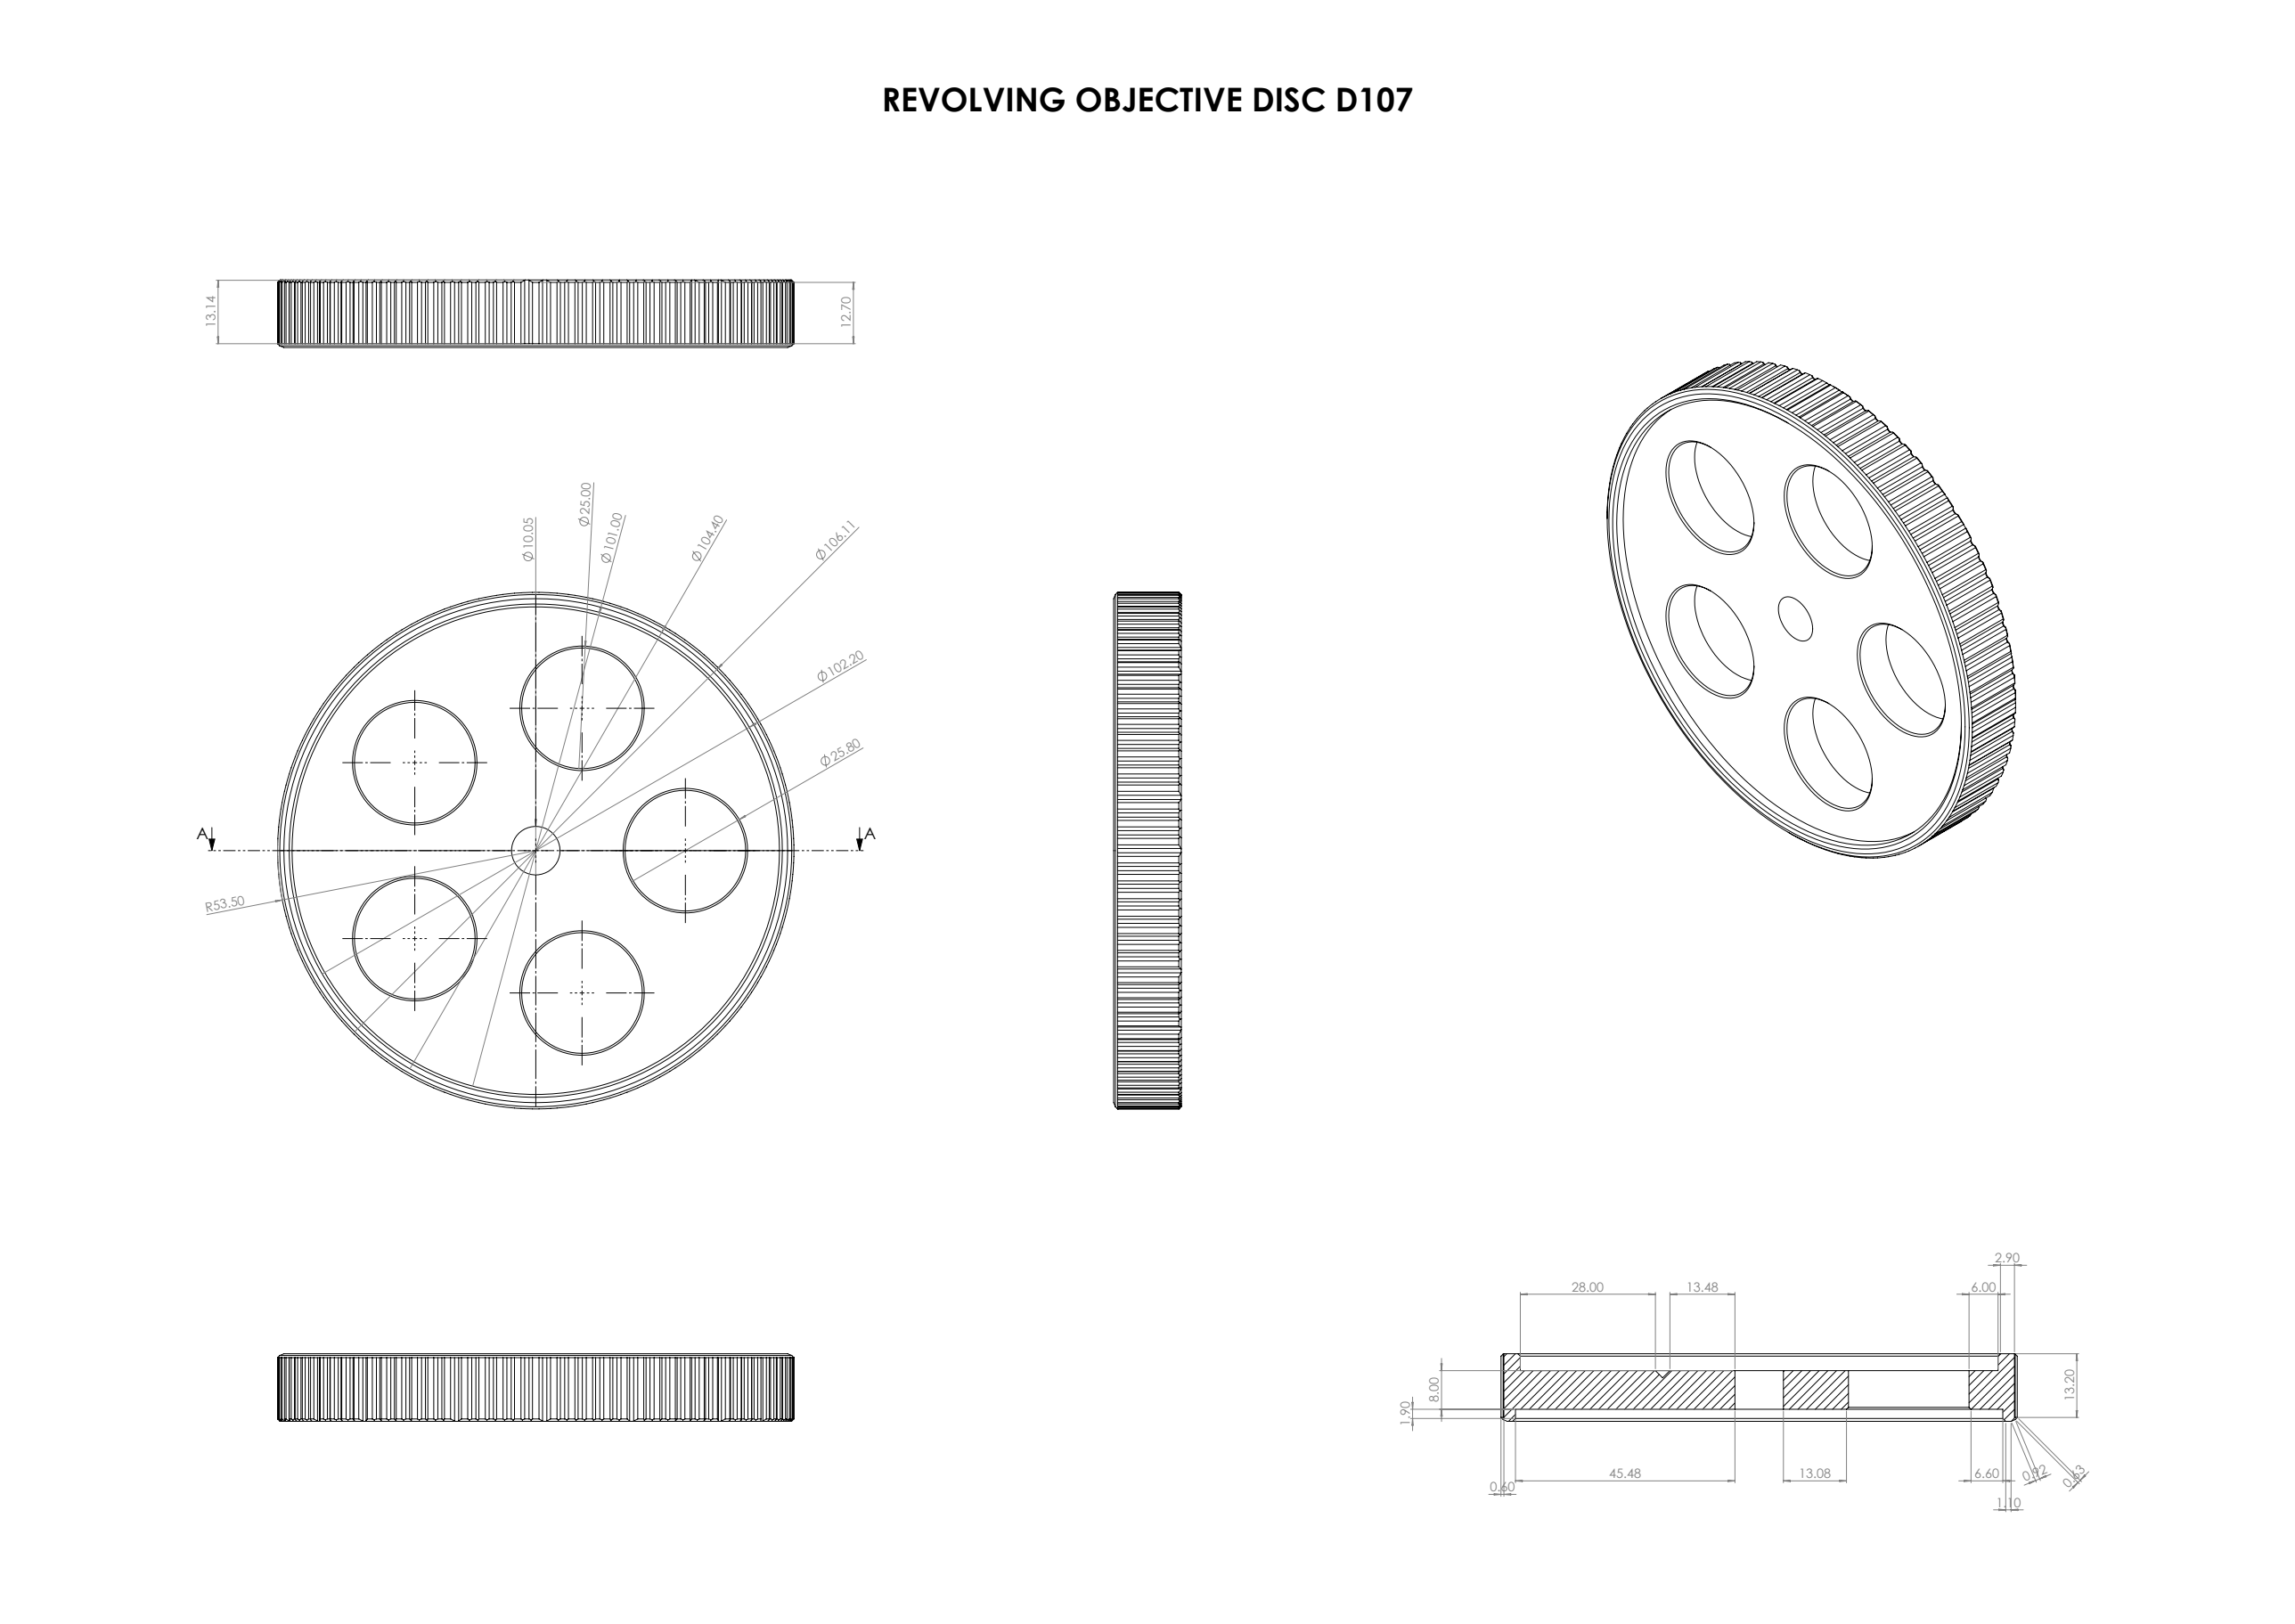
ISO-10303-21;
HEADER;
/* Generated by software containing ST-Developer
 * from STEP Tools, Inc. (www.steptools.com) 
 */

FILE_DESCRIPTION(
/* description */ (''),
/* implementation_level */ '2;1');

FILE_NAME(
/* name */ '02_Revolving_Objective_Disc_D107.step',
/* time_stamp */ '2026-10-21T02:03:06-07:00',
/* author */ (''),
/* organization */ (''),
/* preprocessor_version */ 'ST-DEVELOPER v20.2',
/* originating_system */ 'Autodesk Translation Framework v15.15.0.0',
/* authorisation */ '');

FILE_SCHEMA (('AUTOMOTIVE_DESIGN { 1 0 10303 214 3 1 1 }'));
ENDSEC;

DATA;
#10=MECHANICAL_DESIGN_GEOMETRIC_PRESENTATION_REPRESENTATION('',(#116),#38528);
#92=SHAPE_REPRESENTATION_RELATIONSHIP('SRR','None',#38577,#104);
#104=ADVANCED_BREP_SHAPE_REPRESENTATION('',(#128),#38517);
#116=STYLED_ITEM('',(#38720),#128);
#128=MANIFOLD_SOLID_BREP('Body1',#17073);
#146=CYLINDRICAL_SURFACE('',#17325,53.5);
#147=CYLINDRICAL_SURFACE('',#17331,53.5);
#148=CYLINDRICAL_SURFACE('',#17337,0.700000000000003);
#149=CYLINDRICAL_SURFACE('',#17344,0.700000000000003);
#150=CYLINDRICAL_SURFACE('',#17347,0.700000000000003);
#151=CYLINDRICAL_SURFACE('',#17356,0.700000000000003);
#152=CYLINDRICAL_SURFACE('',#17361,0.700000000000003);
#153=CYLINDRICAL_SURFACE('',#17368,53.5);
#154=CYLINDRICAL_SURFACE('',#17377,53.5);
#155=CYLINDRICAL_SURFACE('',#17384,53.5);
#156=CYLINDRICAL_SURFACE('',#17391,53.5);
#157=CYLINDRICAL_SURFACE('',#17398,53.5);
#158=CYLINDRICAL_SURFACE('',#17405,53.5);
#159=CYLINDRICAL_SURFACE('',#17412,53.5);
#160=CYLINDRICAL_SURFACE('',#17419,53.5);
#161=CYLINDRICAL_SURFACE('',#17426,53.5);
#162=CYLINDRICAL_SURFACE('',#17602,0.700000000000003);
#163=CYLINDRICAL_SURFACE('',#17608,0.700000000000003);
#164=CYLINDRICAL_SURFACE('',#17614,0.700000000000003);
#165=CYLINDRICAL_SURFACE('',#17620,0.700000000000003);
#166=CYLINDRICAL_SURFACE('',#17623,53.5);
#167=CYLINDRICAL_SURFACE('',#17631,53.5);
#168=CYLINDRICAL_SURFACE('',#17637,53.5);
#169=CYLINDRICAL_SURFACE('',#17643,53.5);
#170=CYLINDRICAL_SURFACE('',#17649,53.5);
#171=CYLINDRICAL_SURFACE('',#17655,53.5);
#172=CYLINDRICAL_SURFACE('',#17661,53.5);
#173=CYLINDRICAL_SURFACE('',#17670,53.5);
#174=CYLINDRICAL_SURFACE('',#17672,53.5);
#175=CYLINDRICAL_SURFACE('',#17674,53.5);
#176=CYLINDRICAL_SURFACE('',#17687,0.700000000000003);
#177=CYLINDRICAL_SURFACE('',#17689,0.700000000000003);
#178=CYLINDRICAL_SURFACE('',#17691,0.700000000000003);
#179=CYLINDRICAL_SURFACE('',#17693,0.700000000000003);
#180=CYLINDRICAL_SURFACE('',#17695,0.700000000000003);
#181=CYLINDRICAL_SURFACE('',#17697,0.700000000000003);
#182=CYLINDRICAL_SURFACE('',#17702,0.700000000000003);
#183=CYLINDRICAL_SURFACE('',#17710,0.700000000000003);
#184=CYLINDRICAL_SURFACE('',#17716,0.700000000000003);
#185=CYLINDRICAL_SURFACE('',#17722,0.700000000000003);
#186=CYLINDRICAL_SURFACE('',#17725,53.5);
#187=CYLINDRICAL_SURFACE('',#17733,53.5);
#188=CYLINDRICAL_SURFACE('',#17739,53.5);
#189=CYLINDRICAL_SURFACE('',#17745,53.5);
#190=CYLINDRICAL_SURFACE('',#17751,53.5);
#191=CYLINDRICAL_SURFACE('',#17757,53.5);
#192=CYLINDRICAL_SURFACE('',#17766,53.5);
#193=CYLINDRICAL_SURFACE('',#17768,53.5);
#194=CYLINDRICAL_SURFACE('',#17770,53.5);
#195=CYLINDRICAL_SURFACE('',#17772,53.5);
#196=CYLINDRICAL_SURFACE('',#17783,0.700000000000003);
#197=CYLINDRICAL_SURFACE('',#17785,0.700000000000003);
#198=CYLINDRICAL_SURFACE('',#17787,0.700000000000003);
#199=CYLINDRICAL_SURFACE('',#17789,0.700000000000003);
#200=CYLINDRICAL_SURFACE('',#17791,0.700000000000003);
#201=CYLINDRICAL_SURFACE('',#17796,0.700000000000003);
#202=CYLINDRICAL_SURFACE('',#17802,0.700000000000003);
#203=CYLINDRICAL_SURFACE('',#17808,0.700000000000003);
#204=CYLINDRICAL_SURFACE('',#17814,0.700000000000003);
#205=CYLINDRICAL_SURFACE('',#17820,0.700000000000003);
#206=CYLINDRICAL_SURFACE('',#17823,53.5);
#207=CYLINDRICAL_SURFACE('',#17831,53.5);
#208=CYLINDRICAL_SURFACE('',#17837,53.5);
#209=CYLINDRICAL_SURFACE('',#17843,53.5);
#210=CYLINDRICAL_SURFACE('',#17849,53.5);
#211=CYLINDRICAL_SURFACE('',#17862,53.5);
#212=CYLINDRICAL_SURFACE('',#17864,53.5);
#213=CYLINDRICAL_SURFACE('',#17866,53.5);
#214=CYLINDRICAL_SURFACE('',#17868,53.5);
#215=CYLINDRICAL_SURFACE('',#17870,53.5);
#216=CYLINDRICAL_SURFACE('',#17879,0.700000000000003);
#217=CYLINDRICAL_SURFACE('',#17881,0.700000000000003);
#218=CYLINDRICAL_SURFACE('',#17883,0.700000000000003);
#219=CYLINDRICAL_SURFACE('',#17885,0.700000000000003);
#220=CYLINDRICAL_SURFACE('',#17890,0.700000000000003);
#221=CYLINDRICAL_SURFACE('',#17898,0.700000000000003);
#222=CYLINDRICAL_SURFACE('',#17904,0.700000000000003);
#223=CYLINDRICAL_SURFACE('',#17910,0.700000000000003);
#224=CYLINDRICAL_SURFACE('',#17916,0.700000000000003);
#225=CYLINDRICAL_SURFACE('',#17922,0.700000000000003);
#226=CYLINDRICAL_SURFACE('',#17925,53.5);
#227=CYLINDRICAL_SURFACE('',#17933,53.5);
#228=CYLINDRICAL_SURFACE('',#17939,53.5);
#229=CYLINDRICAL_SURFACE('',#17945,53.5);
#230=CYLINDRICAL_SURFACE('',#17958,53.5);
#231=CYLINDRICAL_SURFACE('',#17960,53.5);
#232=CYLINDRICAL_SURFACE('',#17962,53.5);
#233=CYLINDRICAL_SURFACE('',#17964,53.5);
#234=CYLINDRICAL_SURFACE('',#17966,53.5);
#235=CYLINDRICAL_SURFACE('',#17968,53.5);
#236=CYLINDRICAL_SURFACE('',#17975,0.700000000000003);
#237=CYLINDRICAL_SURFACE('',#17977,0.700000000000003);
#238=CYLINDRICAL_SURFACE('',#17979,0.700000000000003);
#239=CYLINDRICAL_SURFACE('',#17984,0.700000000000003);
#240=CYLINDRICAL_SURFACE('',#17990,0.700000000000003);
#241=CYLINDRICAL_SURFACE('',#17996,0.700000000000003);
#242=CYLINDRICAL_SURFACE('',#18002,0.700000000000003);
#243=CYLINDRICAL_SURFACE('',#18008,0.700000000000003);
#244=CYLINDRICAL_SURFACE('',#18014,0.700000000000003);
#245=CYLINDRICAL_SURFACE('',#18020,0.700000000000003);
#246=CYLINDRICAL_SURFACE('',#18023,53.5);
#247=CYLINDRICAL_SURFACE('',#18031,53.5);
#248=CYLINDRICAL_SURFACE('',#18037,53.5);
#249=CYLINDRICAL_SURFACE('',#18054,53.5);
#250=CYLINDRICAL_SURFACE('',#18056,53.5);
#251=CYLINDRICAL_SURFACE('',#18058,53.5);
#252=CYLINDRICAL_SURFACE('',#18060,53.5);
#253=CYLINDRICAL_SURFACE('',#18062,53.5);
#254=CYLINDRICAL_SURFACE('',#18064,53.5);
#255=CYLINDRICAL_SURFACE('',#18066,53.5);
#256=CYLINDRICAL_SURFACE('',#18071,0.700000000000003);
#257=CYLINDRICAL_SURFACE('',#18073,0.700000000000003);
#258=CYLINDRICAL_SURFACE('',#18078,0.700000000000003);
#259=CYLINDRICAL_SURFACE('',#18084,0.700000000000003);
#260=CYLINDRICAL_SURFACE('',#18090,0.700000000000003);
#261=CYLINDRICAL_SURFACE('',#18096,0.700000000000003);
#262=CYLINDRICAL_SURFACE('',#18102,0.700000000000003);
#263=CYLINDRICAL_SURFACE('',#18108,0.700000000000003);
#264=CYLINDRICAL_SURFACE('',#18114,0.700000000000003);
#265=CYLINDRICAL_SURFACE('',#18120,0.700000000000003);
#266=CYLINDRICAL_SURFACE('',#18123,53.5);
#267=CYLINDRICAL_SURFACE('',#18131,53.5);
#268=CYLINDRICAL_SURFACE('',#18150,53.5);
#269=CYLINDRICAL_SURFACE('',#18152,53.5);
#270=CYLINDRICAL_SURFACE('',#18154,53.5);
#271=CYLINDRICAL_SURFACE('',#18156,53.5);
#272=CYLINDRICAL_SURFACE('',#18158,53.5);
#273=CYLINDRICAL_SURFACE('',#18160,53.5);
#274=CYLINDRICAL_SURFACE('',#18162,53.5);
#275=CYLINDRICAL_SURFACE('',#18164,53.5);
#276=CYLINDRICAL_SURFACE('',#18167,0.700000000000003);
#277=CYLINDRICAL_SURFACE('',#18172,53.5);
#278=CYLINDRICAL_SURFACE('',#18178,53.5);
#279=CYLINDRICAL_SURFACE('',#18184,53.5);
#280=CYLINDRICAL_SURFACE('',#18190,53.5);
#281=CYLINDRICAL_SURFACE('',#18196,53.5);
#282=CYLINDRICAL_SURFACE('',#18202,53.5);
#283=CYLINDRICAL_SURFACE('',#18208,53.5);
#284=CYLINDRICAL_SURFACE('',#18214,53.5);
#285=CYLINDRICAL_SURFACE('',#18220,53.5);
#286=CYLINDRICAL_SURFACE('',#18223,0.700000000000003);
#287=CYLINDRICAL_SURFACE('',#18244,0.700000000000003);
#288=CYLINDRICAL_SURFACE('',#18246,0.700000000000003);
#289=CYLINDRICAL_SURFACE('',#18248,0.700000000000003);
#290=CYLINDRICAL_SURFACE('',#18250,0.700000000000003);
#291=CYLINDRICAL_SURFACE('',#18252,0.700000000000003);
#292=CYLINDRICAL_SURFACE('',#18254,0.700000000000003);
#293=CYLINDRICAL_SURFACE('',#18256,0.700000000000003);
#294=CYLINDRICAL_SURFACE('',#18258,0.700000000000003);
#295=CYLINDRICAL_SURFACE('',#18262,49.5);
#296=CYLINDRICAL_SURFACE('',#18281,0.700000000000003);
#297=CYLINDRICAL_SURFACE('',#18283,0.700000000000003);
#298=CYLINDRICAL_SURFACE('',#18285,0.700000000000003);
#299=CYLINDRICAL_SURFACE('',#18287,0.700000000000003);
#300=CYLINDRICAL_SURFACE('',#18289,0.700000000000003);
#301=CYLINDRICAL_SURFACE('',#18291,0.700000000000003);
#302=CYLINDRICAL_SURFACE('',#18293,0.700000000000003);
#303=CYLINDRICAL_SURFACE('',#18295,0.700000000000003);
#304=CYLINDRICAL_SURFACE('',#18297,0.700000000000003);
#305=CYLINDRICAL_SURFACE('',#18300,0.700000000000003);
#306=CYLINDRICAL_SURFACE('',#18306,0.700000000000003);
#307=CYLINDRICAL_SURFACE('',#18312,0.700000000000003);
#308=CYLINDRICAL_SURFACE('',#18318,0.700000000000003);
#309=CYLINDRICAL_SURFACE('',#18324,0.700000000000003);
#310=CYLINDRICAL_SURFACE('',#18330,0.700000000000003);
#311=CYLINDRICAL_SURFACE('',#18453,12.5);
#312=CYLINDRICAL_SURFACE('',#18457,12.5);
#313=CYLINDRICAL_SURFACE('',#18461,12.5);
#314=CYLINDRICAL_SURFACE('',#18465,12.5);
#315=CYLINDRICAL_SURFACE('',#18469,12.5);
#316=CYLINDRICAL_SURFACE('',#18473,50.5);
#317=CYLINDRICAL_SURFACE('',#18474,53.5);
#318=CYLINDRICAL_SURFACE('',#18475,53.5);
#319=CYLINDRICAL_SURFACE('',#18476,53.5);
#320=CYLINDRICAL_SURFACE('',#18477,53.5);
#321=CYLINDRICAL_SURFACE('',#18478,53.5);
#322=CYLINDRICAL_SURFACE('',#18479,53.5);
#323=CYLINDRICAL_SURFACE('',#18480,53.5);
#324=CYLINDRICAL_SURFACE('',#18481,53.5);
#325=CYLINDRICAL_SURFACE('',#18482,53.5);
#326=CYLINDRICAL_SURFACE('',#18483,53.5);
#327=CYLINDRICAL_SURFACE('',#18490,0.700000000000003);
#328=CYLINDRICAL_SURFACE('',#18502,0.700000000000003);
#329=CYLINDRICAL_SURFACE('',#18514,0.700000000000003);
#330=CYLINDRICAL_SURFACE('',#18558,0.700000000000003);
#331=CYLINDRICAL_SURFACE('',#18568,0.700000000000003);
#332=CYLINDRICAL_SURFACE('',#18580,0.700000000000003);
#333=CYLINDRICAL_SURFACE('',#18596,5.025);
#431=B_SPLINE_CURVE_WITH_KNOTS('',3,(#24013,#24014,#24015,#24016),
 .UNSPECIFIED.,.F.,.F.,(4,4),(0.165217092335985,0.177184346430037),
 .UNSPECIFIED.);
#432=B_SPLINE_CURVE_WITH_KNOTS('',3,(#24020,#24021,#24022,#24023),
 .UNSPECIFIED.,.F.,.F.,(4,4),(0.,0.0446132763744268),.UNSPECIFIED.);
#433=B_SPLINE_CURVE_WITH_KNOTS('',3,(#24050,#24051,#24052,#24053),
 .UNSPECIFIED.,.F.,.F.,(4,4),(0.0319696744346156,0.0766821311551608),
 .UNSPECIFIED.);
#434=B_SPLINE_CURVE_WITH_KNOTS('',3,(#24057,#24058,#24059,#24060),
 .UNSPECIFIED.,.F.,.F.,(4,4),(0.077355308281931,0.0893225623759921),
 .UNSPECIFIED.);
#435=B_SPLINE_CURVE_WITH_KNOTS('',3,(#24072,#24073,#24074,#24075),
 .UNSPECIFIED.,.F.,.F.,(4,4),(0.165217092335986,0.177184346430046),
 .UNSPECIFIED.);
#436=B_SPLINE_CURVE_WITH_KNOTS('',3,(#24102,#24103,#24104,#24105),
 .UNSPECIFIED.,.F.,.F.,(4,4),(0.0319696744346149,0.0766821311551634),
 .UNSPECIFIED.);
#437=B_SPLINE_CURVE_WITH_KNOTS('',3,(#24108,#24109,#24110,#24111),
 .UNSPECIFIED.,.F.,.F.,(4,4),(0.0319696744346139,0.0766821311551655),
 .UNSPECIFIED.);
#438=B_SPLINE_CURVE_WITH_KNOTS('',3,(#24136,#24137,#24138,#24139),
 .UNSPECIFIED.,.F.,.F.,(4,4),(0.031969674434604,0.0766821311551636),
 .UNSPECIFIED.);
#439=B_SPLINE_CURVE_WITH_KNOTS('',3,(#24164,#24165,#24166,#24167),
 .UNSPECIFIED.,.F.,.F.,(4,4),(0.0319696744346154,0.0766821311551577),
 .UNSPECIFIED.);
#440=B_SPLINE_CURVE_WITH_KNOTS('',3,(#24170,#24171,#24172,#24173),
 .UNSPECIFIED.,.F.,.F.,(4,4),(0.0319696744346157,0.0766821311551629),
 .UNSPECIFIED.);
#441=B_SPLINE_CURVE_WITH_KNOTS('',3,(#24207,#24208,#24209,#24210),
 .UNSPECIFIED.,.F.,.F.,(4,4),(0.0773553082819434,0.089322562375993),
 .UNSPECIFIED.);
#442=B_SPLINE_CURVE_WITH_KNOTS('',3,(#24214,#24215,#24216,#24217),
 .UNSPECIFIED.,.F.,.F.,(4,4),(-0.177184216772292,-0.165217092335991),
 .UNSPECIFIED.);
#443=B_SPLINE_CURVE_WITH_KNOTS('',3,(#24225,#24226,#24227,#24228),
 .UNSPECIFIED.,.F.,.F.,(4,4),(0.,0.0964441447221119),.UNSPECIFIED.);
#444=B_SPLINE_CURVE_WITH_KNOTS('',3,(#24230,#24231,#24232,#24233),
 .UNSPECIFIED.,.F.,.F.,(4,4),(0.336279561120239,0.348246685406907),
 .UNSPECIFIED.);
#445=B_SPLINE_CURVE_WITH_KNOTS('',3,(#24258,#24259,#24260,#24261),
 .UNSPECIFIED.,.F.,.F.,(4,4),(0.0319696744346043,0.0766821311551631),
 .UNSPECIFIED.);
#446=B_SPLINE_CURVE_WITH_KNOTS('',3,(#24265,#24266,#24267,#24268),
 .UNSPECIFIED.,.F.,.F.,(4,4),(-0.0893225623759883,-0.0773554379396765),
 .UNSPECIFIED.);
#447=B_SPLINE_CURVE_WITH_KNOTS('',3,(#24269,#24270,#24271,#24272),
 .UNSPECIFIED.,.F.,.F.,(4,4),(0.,0.0964441447217045),.UNSPECIFIED.);
#448=B_SPLINE_CURVE_WITH_KNOTS('',3,(#24296,#24297,#24298,#24299),
 .UNSPECIFIED.,.F.,.F.,(4,4),(0.0319696744346058,0.0766821311551602),
 .UNSPECIFIED.);
#449=B_SPLINE_CURVE_WITH_KNOTS('',3,(#24302,#24303,#24304,#24305),
 .UNSPECIFIED.,.F.,.F.,(4,4),(0.0319696744346046,0.0766821311551621),
 .UNSPECIFIED.);
#450=B_SPLINE_CURVE_WITH_KNOTS('',3,(#24341,#24342,#24343,#24344),
 .UNSPECIFIED.,.F.,.F.,(4,4),(0.0319696744346149,0.0766821311551593),
 .UNSPECIFIED.);
#451=B_SPLINE_CURVE_WITH_KNOTS('',3,(#24347,#24348,#24349,#24350),
 .UNSPECIFIED.,.F.,.F.,(4,4),(0.0319696744346029,0.0766821311551658),
 .UNSPECIFIED.);
#452=B_SPLINE_CURVE_WITH_KNOTS('',3,(#24386,#24387,#24388,#24389),
 .UNSPECIFIED.,.F.,.F.,(4,4),(0.0319696744346075,0.0766821311551552),
 .UNSPECIFIED.);
#453=B_SPLINE_CURVE_WITH_KNOTS('',3,(#24392,#24393,#24394,#24395),
 .UNSPECIFIED.,.F.,.F.,(4,4),(0.0319696744346153,0.0766821311551614),
 .UNSPECIFIED.);
#454=B_SPLINE_CURVE_WITH_KNOTS('',3,(#24431,#24432,#24433,#24434),
 .UNSPECIFIED.,.F.,.F.,(4,4),(0.0319696744346164,0.0766821311551606),
 .UNSPECIFIED.);
#455=B_SPLINE_CURVE_WITH_KNOTS('',3,(#24437,#24438,#24439,#24440),
 .UNSPECIFIED.,.F.,.F.,(4,4),(0.0319696744346151,0.0766821311551609),
 .UNSPECIFIED.);
#456=B_SPLINE_CURVE_WITH_KNOTS('',3,(#24476,#24477,#24478,#24479),
 .UNSPECIFIED.,.F.,.F.,(4,4),(0.0319696744346051,0.076682131155159),
 .UNSPECIFIED.);
#457=B_SPLINE_CURVE_WITH_KNOTS('',3,(#24482,#24483,#24484,#24485),
 .UNSPECIFIED.,.F.,.F.,(4,4),(0.0319696744346129,0.0766821311551604),
 .UNSPECIFIED.);
#458=B_SPLINE_CURVE_WITH_KNOTS('',3,(#24521,#24522,#24523,#24524),
 .UNSPECIFIED.,.F.,.F.,(4,4),(0.0319696744346068,0.0766821311551503),
 .UNSPECIFIED.);
#459=B_SPLINE_CURVE_WITH_KNOTS('',3,(#24527,#24528,#24529,#24530),
 .UNSPECIFIED.,.F.,.F.,(4,4),(0.031969674434606,0.0766821311551618),
 .UNSPECIFIED.);
#460=B_SPLINE_CURVE_WITH_KNOTS('',3,(#24566,#24567,#24568,#24569),
 .UNSPECIFIED.,.F.,.F.,(4,4),(0.0319696744346057,0.0766821311551617),
 .UNSPECIFIED.);
#461=B_SPLINE_CURVE_WITH_KNOTS('',3,(#24572,#24573,#24574,#24575),
 .UNSPECIFIED.,.F.,.F.,(4,4),(0.0319696744346062,0.0766821311551594),
 .UNSPECIFIED.);
#462=B_SPLINE_CURVE_WITH_KNOTS('',3,(#24611,#24612,#24613,#24614),
 .UNSPECIFIED.,.F.,.F.,(4,4),(0.0319696744346062,0.0766821311551613),
 .UNSPECIFIED.);
#463=B_SPLINE_CURVE_WITH_KNOTS('',3,(#24617,#24618,#24619,#24620),
 .UNSPECIFIED.,.F.,.F.,(4,4),(0.0319696744346139,0.0766821311551679),
 .UNSPECIFIED.);
#464=B_SPLINE_CURVE_WITH_KNOTS('',3,(#24641,#24642,#24643,#24644,#24645,
#24646),.UNSPECIFIED.,.F.,.F.,(4,2,4),(1.36037627907923,1.38960835652673,
1.40296484627234),.UNSPECIFIED.);
#465=B_SPLINE_CURVE_WITH_KNOTS('',3,(#24662,#24663,#24664,#24665),
 .UNSPECIFIED.,.F.,.F.,(4,4),(0.16521709233599,0.177184216772299),
 .UNSPECIFIED.);
#466=B_SPLINE_CURVE_WITH_KNOTS('',3,(#24983,#24984,#24985,#24986),
 .UNSPECIFIED.,.F.,.F.,(4,4),(-0.0893225623759853,-0.0773554379396747),
 .UNSPECIFIED.);
#467=B_SPLINE_CURVE_WITH_KNOTS('',3,(#25013,#25014,#25015,#25016),
 .UNSPECIFIED.,.F.,.F.,(4,4),(0.0319696744346003,0.0766821311551615),
 .UNSPECIFIED.);
#468=B_SPLINE_CURVE_WITH_KNOTS('',3,(#25017,#25018,#25019,#25020),
 .UNSPECIFIED.,.F.,.F.,(4,4),(0.0319696744346077,0.0766821311551524),
 .UNSPECIFIED.);
#469=B_SPLINE_CURVE_WITH_KNOTS('',3,(#25055,#25056,#25057,#25058),
 .UNSPECIFIED.,.F.,.F.,(4,4),(0.0319696744346155,0.0766821311551595),
 .UNSPECIFIED.);
#470=B_SPLINE_CURVE_WITH_KNOTS('',3,(#25059,#25060,#25061,#25062),
 .UNSPECIFIED.,.F.,.F.,(4,4),(0.0319696744346145,0.0766821311551639),
 .UNSPECIFIED.);
#471=B_SPLINE_CURVE_WITH_KNOTS('',3,(#25097,#25098,#25099,#25100),
 .UNSPECIFIED.,.F.,.F.,(4,4),(0.0319696744346048,0.0766821311551673),
 .UNSPECIFIED.);
#472=B_SPLINE_CURVE_WITH_KNOTS('',3,(#25101,#25102,#25103,#25104),
 .UNSPECIFIED.,.F.,.F.,(4,4),(0.0319696744346148,0.0766821311551611),
 .UNSPECIFIED.);
#473=B_SPLINE_CURVE_WITH_KNOTS('',3,(#25147,#25148,#25149,#25150),
 .UNSPECIFIED.,.F.,.F.,(4,4),(0.0319696744346167,0.0766821311551506),
 .UNSPECIFIED.);
#474=B_SPLINE_CURVE_WITH_KNOTS('',3,(#25151,#25152,#25153,#25154),
 .UNSPECIFIED.,.F.,.F.,(4,4),(0.0773553082819305,0.0893225623759919),
 .UNSPECIFIED.);
#475=B_SPLINE_CURVE_WITH_KNOTS('',3,(#25189,#25190,#25191,#25192),
 .UNSPECIFIED.,.F.,.F.,(4,4),(0.0319696744346161,0.0766821311551558),
 .UNSPECIFIED.);
#476=B_SPLINE_CURVE_WITH_KNOTS('',3,(#25193,#25194,#25195,#25196),
 .UNSPECIFIED.,.F.,.F.,(4,4),(0.031969674434606,0.0766821311551616),
 .UNSPECIFIED.);
#477=B_SPLINE_CURVE_WITH_KNOTS('',3,(#25231,#25232,#25233,#25234),
 .UNSPECIFIED.,.F.,.F.,(4,4),(0.031969674434617,0.0766821311551659),
 .UNSPECIFIED.);
#478=B_SPLINE_CURVE_WITH_KNOTS('',3,(#25235,#25236,#25237,#25238),
 .UNSPECIFIED.,.F.,.F.,(4,4),(0.0319696744346159,0.0766821311551567),
 .UNSPECIFIED.);
#479=B_SPLINE_CURVE_WITH_KNOTS('',3,(#25273,#25274,#25275,#25276),
 .UNSPECIFIED.,.F.,.F.,(4,4),(0.0319696744346169,0.0766821311551513),
 .UNSPECIFIED.);
#480=B_SPLINE_CURVE_WITH_KNOTS('',3,(#25277,#25278,#25279,#25280),
 .UNSPECIFIED.,.F.,.F.,(4,4),(0.0319696744346152,0.0766821311551648),
 .UNSPECIFIED.);
#481=B_SPLINE_CURVE_WITH_KNOTS('',3,(#25315,#25316,#25317,#25318),
 .UNSPECIFIED.,.F.,.F.,(4,4),(0.0319696744346174,0.0766821311551486),
 .UNSPECIFIED.);
#482=B_SPLINE_CURVE_WITH_KNOTS('',3,(#25319,#25320,#25321,#25322),
 .UNSPECIFIED.,.F.,.F.,(4,4),(0.0319696744346054,0.0766821311551601),
 .UNSPECIFIED.);
#483=B_SPLINE_CURVE_WITH_KNOTS('',3,(#25357,#25358,#25359,#25360),
 .UNSPECIFIED.,.F.,.F.,(4,4),(0.165217092335987,0.177184346430039),
 .UNSPECIFIED.);
#484=B_SPLINE_CURVE_WITH_KNOTS('',3,(#25361,#25362,#25363,#25364),
 .UNSPECIFIED.,.F.,.F.,(4,4),(0.0319696744346053,0.0766821311551563),
 .UNSPECIFIED.);
#485=B_SPLINE_CURVE_WITH_KNOTS('',3,(#25377,#25378,#25379,#25380),
 .UNSPECIFIED.,.F.,.F.,(4,4),(0.,0.0964441447213629),.UNSPECIFIED.);
#486=B_SPLINE_CURVE_WITH_KNOTS('',3,(#25382,#25383,#25384,#25385),
 .UNSPECIFIED.,.F.,.F.,(4,4),(-0.0893225623759869,-0.0773554379396867),
 .UNSPECIFIED.);
#487=B_SPLINE_CURVE_WITH_KNOTS('',3,(#25445,#25446,#25447,#25448),
 .UNSPECIFIED.,.F.,.F.,(4,4),(0.,0.0446132763744278),.UNSPECIFIED.);
#488=B_SPLINE_CURVE_WITH_KNOTS('',3,(#25449,#25450,#25451,#25452),
 .UNSPECIFIED.,.F.,.F.,(4,4),(0.0319696744346159,0.0766821311551664),
 .UNSPECIFIED.);
#489=B_SPLINE_CURVE_WITH_KNOTS('',3,(#25472,#25473,#25474,#25475),
 .UNSPECIFIED.,.F.,.F.,(4,4),(0.0319696744346157,0.0766821311551561),
 .UNSPECIFIED.);
#490=B_SPLINE_CURVE_WITH_KNOTS('',3,(#25493,#25494,#25495,#25496),
 .UNSPECIFIED.,.F.,.F.,(4,4),(0.0319696744346008,0.076682131155157),
 .UNSPECIFIED.);
#491=B_SPLINE_CURVE_WITH_KNOTS('',3,(#25531,#25532,#25533,#25534),
 .UNSPECIFIED.,.F.,.F.,(4,4),(0.0319696744346162,0.0766821311551517),
 .UNSPECIFIED.);
#492=B_SPLINE_CURVE_WITH_KNOTS('',3,(#25535,#25536,#25537,#25538),
 .UNSPECIFIED.,.F.,.F.,(4,4),(0.031969674434614,0.0766821311551579),
 .UNSPECIFIED.);
#493=B_SPLINE_CURVE_WITH_KNOTS('',3,(#25573,#25574,#25575,#25576),
 .UNSPECIFIED.,.F.,.F.,(4,4),(0.0319696744346152,0.0766821311551576),
 .UNSPECIFIED.);
#494=B_SPLINE_CURVE_WITH_KNOTS('',3,(#25577,#25578,#25579,#25580),
 .UNSPECIFIED.,.F.,.F.,(4,4),(0.0319696744346146,0.076682131155164),
 .UNSPECIFIED.);
#495=B_SPLINE_CURVE_WITH_KNOTS('',3,(#25603,#25604,#25605,#25606),
 .UNSPECIFIED.,.F.,.F.,(4,4),(0.165217092335987,0.177184346430036),
 .UNSPECIFIED.);
#496=B_SPLINE_CURVE_WITH_KNOTS('',3,(#25630,#25631,#25632,#25633),
 .UNSPECIFIED.,.F.,.F.,(4,4),(0.0319696744346059,0.0766821311551569),
 .UNSPECIFIED.);
#497=B_SPLINE_CURVE_WITH_KNOTS('',3,(#25634,#25635,#25636,#25637),
 .UNSPECIFIED.,.F.,.F.,(4,4),(0.0773553082819314,0.0893225623759902),
 .UNSPECIFIED.);
#498=B_SPLINE_CURVE_WITH_KNOTS('',3,(#25672,#25673,#25674,#25675),
 .UNSPECIFIED.,.F.,.F.,(4,4),(0.0319696744345999,0.0766821311551614),
 .UNSPECIFIED.);
#499=B_SPLINE_CURVE_WITH_KNOTS('',3,(#25676,#25677,#25678,#25679),
 .UNSPECIFIED.,.F.,.F.,(4,4),(0.0319696744346005,0.0766821311551545),
 .UNSPECIFIED.);
#500=B_SPLINE_CURVE_WITH_KNOTS('',3,(#25714,#25715,#25716,#25717),
 .UNSPECIFIED.,.F.,.F.,(4,4),(0.0319696744346044,0.0766821311551586),
 .UNSPECIFIED.);
#501=B_SPLINE_CURVE_WITH_KNOTS('',3,(#25718,#25719,#25720,#25721),
 .UNSPECIFIED.,.F.,.F.,(4,4),(0.0319696744346146,0.0766821311551602),
 .UNSPECIFIED.);
#502=B_SPLINE_CURVE_WITH_KNOTS('',3,(#25756,#25757,#25758,#25759),
 .UNSPECIFIED.,.F.,.F.,(4,4),(0.0319696744345999,0.0766821311551589),
 .UNSPECIFIED.);
#503=B_SPLINE_CURVE_WITH_KNOTS('',3,(#25760,#25761,#25762,#25763),
 .UNSPECIFIED.,.F.,.F.,(4,4),(0.0319696744346151,0.0766821311551586),
 .UNSPECIFIED.);
#504=B_SPLINE_CURVE_WITH_KNOTS('',3,(#25798,#25799,#25800,#25801),
 .UNSPECIFIED.,.F.,.F.,(4,4),(0.165217092335985,0.177184346430047),
 .UNSPECIFIED.);
#505=B_SPLINE_CURVE_WITH_KNOTS('',3,(#25802,#25803,#25804,#25805),
 .UNSPECIFIED.,.F.,.F.,(4,4),(0.,0.0446132763744527),.UNSPECIFIED.);
#506=B_SPLINE_CURVE_WITH_KNOTS('',3,(#25818,#25819,#25820,#25821),
 .UNSPECIFIED.,.F.,.F.,(4,4),(0.,0.0964441447213381),.UNSPECIFIED.);
#507=B_SPLINE_CURVE_WITH_KNOTS('',3,(#25823,#25824,#25825,#25826),
 .UNSPECIFIED.,.F.,.F.,(4,4),(-0.0893225623759864,-0.0773554379396737),
 .UNSPECIFIED.);
#508=B_SPLINE_CURVE_WITH_KNOTS('',3,(#25884,#25885,#25886,#25887),
 .UNSPECIFIED.,.F.,.F.,(4,4),(0.0319696744346151,0.0766821311551646),
 .UNSPECIFIED.);
#509=B_SPLINE_CURVE_WITH_KNOTS('',3,(#25888,#25889,#25890,#25891),
 .UNSPECIFIED.,.F.,.F.,(4,4),(0.0319696744346152,0.0766821311551612),
 .UNSPECIFIED.);
#510=B_SPLINE_CURVE_WITH_KNOTS('',3,(#25926,#25927,#25928,#25929),
 .UNSPECIFIED.,.F.,.F.,(4,4),(0.031969674434616,0.0766821311551564),
 .UNSPECIFIED.);
#511=B_SPLINE_CURVE_WITH_KNOTS('',3,(#25930,#25931,#25932,#25933),
 .UNSPECIFIED.,.F.,.F.,(4,4),(0.0319696744346053,0.0766821311551682),
 .UNSPECIFIED.);
#512=B_SPLINE_CURVE_WITH_KNOTS('',3,(#25968,#25969,#25970,#25971),
 .UNSPECIFIED.,.F.,.F.,(4,4),(0.0319696744346154,0.0766821311551632),
 .UNSPECIFIED.);
#513=B_SPLINE_CURVE_WITH_KNOTS('',3,(#25972,#25973,#25974,#25975),
 .UNSPECIFIED.,.F.,.F.,(4,4),(0.0319696744346182,0.0766821311551516),
 .UNSPECIFIED.);
#514=B_SPLINE_CURVE_WITH_KNOTS('',3,(#26010,#26011,#26012,#26013),
 .UNSPECIFIED.,.F.,.F.,(4,4),(0.0319696744346054,0.076682131155166),
 .UNSPECIFIED.);
#515=B_SPLINE_CURVE_WITH_KNOTS('',3,(#26014,#26015,#26016,#26017),
 .UNSPECIFIED.,.F.,.F.,(4,4),(0.0319696744346067,0.0766821311551598),
 .UNSPECIFIED.);
#516=B_SPLINE_CURVE_WITH_KNOTS('',3,(#26052,#26053,#26054,#26055),
 .UNSPECIFIED.,.F.,.F.,(4,4),(0.0319696744346162,0.0766821311551578),
 .UNSPECIFIED.);
#517=B_SPLINE_CURVE_WITH_KNOTS('',3,(#26056,#26057,#26058,#26059),
 .UNSPECIFIED.,.F.,.F.,(4,4),(0.0319696744346034,0.0766821311551686),
 .UNSPECIFIED.);
#518=B_SPLINE_CURVE_WITH_KNOTS('',3,(#26082,#26083,#26084,#26085),
 .UNSPECIFIED.,.F.,.F.,(4,4),(0.165217092335987,0.17718434643005),
 .UNSPECIFIED.);
#519=B_SPLINE_CURVE_WITH_KNOTS('',3,(#26109,#26110,#26111,#26112),
 .UNSPECIFIED.,.F.,.F.,(4,4),(0.0319696744346091,0.0766821311551474),
 .UNSPECIFIED.);
#520=B_SPLINE_CURVE_WITH_KNOTS('',3,(#26113,#26114,#26115,#26116),
 .UNSPECIFIED.,.F.,.F.,(4,4),(0.077355308281932,0.0893225623759954),
 .UNSPECIFIED.);
#521=B_SPLINE_CURVE_WITH_KNOTS('',3,(#26151,#26152,#26153,#26154),
 .UNSPECIFIED.,.F.,.F.,(4,4),(0.0319696744346146,0.0766821311551647),
 .UNSPECIFIED.);
#522=B_SPLINE_CURVE_WITH_KNOTS('',3,(#26155,#26156,#26157,#26158),
 .UNSPECIFIED.,.F.,.F.,(4,4),(0.0319696744346137,0.0766821311551644),
 .UNSPECIFIED.);
#523=B_SPLINE_CURVE_WITH_KNOTS('',3,(#26193,#26194,#26195,#26196),
 .UNSPECIFIED.,.F.,.F.,(4,4),(0.0319696744346069,0.0766821311551582),
 .UNSPECIFIED.);
#524=B_SPLINE_CURVE_WITH_KNOTS('',3,(#26197,#26198,#26199,#26200),
 .UNSPECIFIED.,.F.,.F.,(4,4),(0.0319696744346155,0.0766821311551643),
 .UNSPECIFIED.);
#525=B_SPLINE_CURVE_WITH_KNOTS('',3,(#26235,#26236,#26237,#26238),
 .UNSPECIFIED.,.F.,.F.,(4,4),(0.165217092335985,0.177184346430037),
 .UNSPECIFIED.);
#526=B_SPLINE_CURVE_WITH_KNOTS('',3,(#26239,#26240,#26241,#26242),
 .UNSPECIFIED.,.F.,.F.,(4,4),(0.031969674434605,0.0766821311551589),
 .UNSPECIFIED.);
#527=B_SPLINE_CURVE_WITH_KNOTS('',3,(#26255,#26256,#26257,#26258),
 .UNSPECIFIED.,.F.,.F.,(4,4),(0.,0.0964441447218811),.UNSPECIFIED.);
#528=B_SPLINE_CURVE_WITH_KNOTS('',3,(#26260,#26261,#26262,#26263),
 .UNSPECIFIED.,.F.,.F.,(4,4),(-0.0893225623759877,-0.0773554379396747),
 .UNSPECIFIED.);
#529=B_SPLINE_CURVE_WITH_KNOTS('',3,(#26323,#26324,#26325,#26326),
 .UNSPECIFIED.,.F.,.F.,(4,4),(0.,0.0446132763744454),.UNSPECIFIED.);
#530=B_SPLINE_CURVE_WITH_KNOTS('',3,(#26327,#26328,#26329,#26330),
 .UNSPECIFIED.,.F.,.F.,(4,4),(0.0319696744346051,0.0766821311551664),
 .UNSPECIFIED.);
#531=B_SPLINE_CURVE_WITH_KNOTS('',3,(#26350,#26351,#26352,#26353),
 .UNSPECIFIED.,.F.,.F.,(4,4),(0.0319696744346155,0.0766821311551594),
 .UNSPECIFIED.);
#532=B_SPLINE_CURVE_WITH_KNOTS('',3,(#26371,#26372,#26373,#26374),
 .UNSPECIFIED.,.F.,.F.,(4,4),(0.0319696744346062,0.0766821311551557),
 .UNSPECIFIED.);
#533=B_SPLINE_CURVE_WITH_KNOTS('',3,(#26409,#26410,#26411,#26412),
 .UNSPECIFIED.,.F.,.F.,(4,4),(0.0319696744346158,0.07668213115516),
 .UNSPECIFIED.);
#534=B_SPLINE_CURVE_WITH_KNOTS('',3,(#26413,#26414,#26415,#26416),
 .UNSPECIFIED.,.F.,.F.,(4,4),(0.0319696744346155,0.0766821311551679),
 .UNSPECIFIED.);
#535=B_SPLINE_CURVE_WITH_KNOTS('',3,(#26451,#26452,#26453,#26454),
 .UNSPECIFIED.,.F.,.F.,(4,4),(0.0319696744346141,0.0766821311551622),
 .UNSPECIFIED.);
#536=B_SPLINE_CURVE_WITH_KNOTS('',3,(#26455,#26456,#26457,#26458),
 .UNSPECIFIED.,.F.,.F.,(4,4),(0.0319696744346023,0.0766821311551525),
 .UNSPECIFIED.);
#537=B_SPLINE_CURVE_WITH_KNOTS('',3,(#26493,#26494,#26495,#26496),
 .UNSPECIFIED.,.F.,.F.,(4,4),(0.0319696744346052,0.0766821311551627),
 .UNSPECIFIED.);
#538=B_SPLINE_CURVE_WITH_KNOTS('',3,(#26497,#26498,#26499,#26500),
 .UNSPECIFIED.,.F.,.F.,(4,4),(0.031969674434614,0.076682131155166),
 .UNSPECIFIED.);
#539=B_SPLINE_CURVE_WITH_KNOTS('',3,(#26535,#26536,#26537,#26538),
 .UNSPECIFIED.,.F.,.F.,(4,4),(0.0319696744345985,0.0766821311551622),
 .UNSPECIFIED.);
#540=B_SPLINE_CURVE_WITH_KNOTS('',3,(#26539,#26540,#26541,#26542),
 .UNSPECIFIED.,.F.,.F.,(4,4),(0.031969674434617,0.0766821311551562),
 .UNSPECIFIED.);
#541=B_SPLINE_CURVE_WITH_KNOTS('',3,(#26565,#26566,#26567,#26568),
 .UNSPECIFIED.,.F.,.F.,(4,4),(0.165217092335983,0.177184346430045),
 .UNSPECIFIED.);
#542=B_SPLINE_CURVE_WITH_KNOTS('',3,(#26592,#26593,#26594,#26595),
 .UNSPECIFIED.,.F.,.F.,(4,4),(0.0319696744346161,0.0766821311551627),
 .UNSPECIFIED.);
#543=B_SPLINE_CURVE_WITH_KNOTS('',3,(#26596,#26597,#26598,#26599),
 .UNSPECIFIED.,.F.,.F.,(4,4),(0.0773553082819429,0.089322562375992),
 .UNSPECIFIED.);
#544=B_SPLINE_CURVE_WITH_KNOTS('',3,(#26634,#26635,#26636,#26637),
 .UNSPECIFIED.,.F.,.F.,(4,4),(0.0319696744346067,0.0766821311551616),
 .UNSPECIFIED.);
#545=B_SPLINE_CURVE_WITH_KNOTS('',3,(#26638,#26639,#26640,#26641),
 .UNSPECIFIED.,.F.,.F.,(4,4),(0.0319696744346059,0.0766821311551612),
 .UNSPECIFIED.);
#546=B_SPLINE_CURVE_WITH_KNOTS('',3,(#26676,#26677,#26678,#26679),
 .UNSPECIFIED.,.F.,.F.,(4,4),(0.165217092335982,0.177184346430035),
 .UNSPECIFIED.);
#547=B_SPLINE_CURVE_WITH_KNOTS('',3,(#26680,#26681,#26682,#26683),
 .UNSPECIFIED.,.F.,.F.,(4,4),(0.,0.0446132763744144),.UNSPECIFIED.);
#548=B_SPLINE_CURVE_WITH_KNOTS('',3,(#26696,#26697,#26698,#26699),
 .UNSPECIFIED.,.F.,.F.,(4,4),(0.,0.0964441447215326),.UNSPECIFIED.);
#549=B_SPLINE_CURVE_WITH_KNOTS('',3,(#26701,#26702,#26703,#26704),
 .UNSPECIFIED.,.F.,.F.,(4,4),(-0.0893225623759896,-0.077355437939685),
 .UNSPECIFIED.);
#550=B_SPLINE_CURVE_WITH_KNOTS('',3,(#26762,#26763,#26764,#26765),
 .UNSPECIFIED.,.F.,.F.,(4,4),(0.0319696744346159,0.0766821311551599),
 .UNSPECIFIED.);
#551=B_SPLINE_CURVE_WITH_KNOTS('',3,(#26766,#26767,#26768,#26769),
 .UNSPECIFIED.,.F.,.F.,(4,4),(0.0319696744346145,0.0766821311551639),
 .UNSPECIFIED.);
#552=B_SPLINE_CURVE_WITH_KNOTS('',3,(#26804,#26805,#26806,#26807),
 .UNSPECIFIED.,.F.,.F.,(4,4),(0.0319696744346048,0.0766821311551603),
 .UNSPECIFIED.);
#553=B_SPLINE_CURVE_WITH_KNOTS('',3,(#26808,#26809,#26810,#26811),
 .UNSPECIFIED.,.F.,.F.,(4,4),(0.0319696744346048,0.0766821311551578),
 .UNSPECIFIED.);
#554=B_SPLINE_CURVE_WITH_KNOTS('',3,(#26846,#26847,#26848,#26849),
 .UNSPECIFIED.,.F.,.F.,(4,4),(0.0319696744346148,0.0766821311551675),
 .UNSPECIFIED.);
#555=B_SPLINE_CURVE_WITH_KNOTS('',3,(#26850,#26851,#26852,#26853),
 .UNSPECIFIED.,.F.,.F.,(4,4),(0.0319696744346143,0.0766821311551628),
 .UNSPECIFIED.);
#556=B_SPLINE_CURVE_WITH_KNOTS('',3,(#26888,#26889,#26890,#26891),
 .UNSPECIFIED.,.F.,.F.,(4,4),(0.031969674434616,0.07668213115516),
 .UNSPECIFIED.);
#557=B_SPLINE_CURVE_WITH_KNOTS('',3,(#26892,#26893,#26894,#26895),
 .UNSPECIFIED.,.F.,.F.,(4,4),(0.0319696744346167,0.0766821311551533),
 .UNSPECIFIED.);
#558=B_SPLINE_CURVE_WITH_KNOTS('',3,(#26930,#26931,#26932,#26933),
 .UNSPECIFIED.,.F.,.F.,(4,4),(0.031969674434616,0.0766821311551576),
 .UNSPECIFIED.);
#559=B_SPLINE_CURVE_WITH_KNOTS('',3,(#26934,#26935,#26936,#26937),
 .UNSPECIFIED.,.F.,.F.,(4,4),(0.0319696744346139,0.0766821311551655),
 .UNSPECIFIED.);
#560=B_SPLINE_CURVE_WITH_KNOTS('',3,(#26972,#26973,#26974,#26975),
 .UNSPECIFIED.,.F.,.F.,(4,4),(0.0319696744346157,0.0766821311551638),
 .UNSPECIFIED.);
#561=B_SPLINE_CURVE_WITH_KNOTS('',3,(#26976,#26977,#26978,#26979),
 .UNSPECIFIED.,.F.,.F.,(4,4),(0.0319696744346155,0.0766821311551616),
 .UNSPECIFIED.);
#562=B_SPLINE_CURVE_WITH_KNOTS('',3,(#27014,#27015,#27016,#27017),
 .UNSPECIFIED.,.F.,.F.,(4,4),(0.0319696744346065,0.0766821311551571),
 .UNSPECIFIED.);
#563=B_SPLINE_CURVE_WITH_KNOTS('',3,(#27018,#27019,#27020,#27021),
 .UNSPECIFIED.,.F.,.F.,(4,4),(0.0319696744346042,0.0766821311551645),
 .UNSPECIFIED.);
#564=B_SPLINE_CURVE_WITH_KNOTS('',3,(#27044,#27045,#27046,#27047),
 .UNSPECIFIED.,.F.,.F.,(4,4),(0.165217092335988,0.177184346430048),
 .UNSPECIFIED.);
#565=B_SPLINE_CURVE_WITH_KNOTS('',3,(#27071,#27072,#27073,#27074),
 .UNSPECIFIED.,.F.,.F.,(4,4),(0.0319696744346034,0.0766821311551701),
 .UNSPECIFIED.);
#566=B_SPLINE_CURVE_WITH_KNOTS('',3,(#27075,#27076,#27077,#27078),
 .UNSPECIFIED.,.F.,.F.,(4,4),(0.0773553082819422,0.0893225623759928),
 .UNSPECIFIED.);
#567=B_SPLINE_CURVE_WITH_KNOTS('',3,(#27113,#27114,#27115,#27116),
 .UNSPECIFIED.,.F.,.F.,(4,4),(0.165217092335984,0.177184346430047),
 .UNSPECIFIED.);
#568=B_SPLINE_CURVE_WITH_KNOTS('',3,(#27117,#27118,#27119,#27120),
 .UNSPECIFIED.,.F.,.F.,(4,4),(0.0319696744346047,0.0766821311551648),
 .UNSPECIFIED.);
#569=B_SPLINE_CURVE_WITH_KNOTS('',3,(#27133,#27134,#27135,#27136),
 .UNSPECIFIED.,.F.,.F.,(4,4),(0.,0.0964441447216793),.UNSPECIFIED.);
#570=B_SPLINE_CURVE_WITH_KNOTS('',3,(#27138,#27139,#27140,#27141),
 .UNSPECIFIED.,.F.,.F.,(4,4),(-0.0893225623759868,-0.077355437939685),
 .UNSPECIFIED.);
#571=B_SPLINE_CURVE_WITH_KNOTS('',3,(#27201,#27202,#27203,#27204),
 .UNSPECIFIED.,.F.,.F.,(4,4),(0.0319696744346011,0.0766821311551579),
 .UNSPECIFIED.);
#572=B_SPLINE_CURVE_WITH_KNOTS('',3,(#27205,#27206,#27207,#27208),
 .UNSPECIFIED.,.F.,.F.,(4,4),(0.031969674434615,0.0766821311551662),
 .UNSPECIFIED.);
#573=B_SPLINE_CURVE_WITH_KNOTS('',3,(#27243,#27244,#27245,#27246),
 .UNSPECIFIED.,.F.,.F.,(4,4),(0.0319696744346163,0.0766821311551522),
 .UNSPECIFIED.);
#574=B_SPLINE_CURVE_WITH_KNOTS('',3,(#27247,#27248,#27249,#27250),
 .UNSPECIFIED.,.F.,.F.,(4,4),(0.0319696744346142,0.0766821311551595),
 .UNSPECIFIED.);
#575=B_SPLINE_CURVE_WITH_KNOTS('',3,(#27285,#27286,#27287,#27288),
 .UNSPECIFIED.,.F.,.F.,(4,4),(0.0319696744346053,0.0766821311551585),
 .UNSPECIFIED.);
#576=B_SPLINE_CURVE_WITH_KNOTS('',3,(#27289,#27290,#27291,#27292),
 .UNSPECIFIED.,.F.,.F.,(4,4),(0.0319696744346046,0.0766821311551665),
 .UNSPECIFIED.);
#577=B_SPLINE_CURVE_WITH_KNOTS('',3,(#27327,#27328,#27329,#27330),
 .UNSPECIFIED.,.F.,.F.,(4,4),(0.0319696744346158,0.0766821311551619),
 .UNSPECIFIED.);
#578=B_SPLINE_CURVE_WITH_KNOTS('',3,(#27331,#27332,#27333,#27334),
 .UNSPECIFIED.,.F.,.F.,(4,4),(0.0319696744346162,0.0766821311551531),
 .UNSPECIFIED.);
#579=B_SPLINE_CURVE_WITH_KNOTS('',3,(#27369,#27370,#27371,#27372),
 .UNSPECIFIED.,.F.,.F.,(4,4),(0.0319696744346129,0.0766821311551683),
 .UNSPECIFIED.);
#580=B_SPLINE_CURVE_WITH_KNOTS('',3,(#27373,#27374,#27375,#27376),
 .UNSPECIFIED.,.F.,.F.,(4,4),(0.0319696744346159,0.0766821311551596),
 .UNSPECIFIED.);
#581=B_SPLINE_CURVE_WITH_KNOTS('',3,(#27411,#27412,#27413,#27414),
 .UNSPECIFIED.,.F.,.F.,(4,4),(0.0319696744346056,0.076682131155164),
 .UNSPECIFIED.);
#582=B_SPLINE_CURVE_WITH_KNOTS('',3,(#27415,#27416,#27417,#27418),
 .UNSPECIFIED.,.F.,.F.,(4,4),(0.031969674434616,0.0766821311551558),
 .UNSPECIFIED.);
#583=B_SPLINE_CURVE_WITH_KNOTS('',3,(#27453,#27454,#27455,#27456),
 .UNSPECIFIED.,.F.,.F.,(4,4),(0.0319696744346056,0.0766821311551581),
 .UNSPECIFIED.);
#584=B_SPLINE_CURVE_WITH_KNOTS('',3,(#27457,#27458,#27459,#27460),
 .UNSPECIFIED.,.F.,.F.,(4,4),(0.0319696744346045,0.0766821311551705),
 .UNSPECIFIED.);
#585=B_SPLINE_CURVE_WITH_KNOTS('',3,(#27495,#27496,#27497,#27498),
 .UNSPECIFIED.,.F.,.F.,(4,4),(0.0319696744346149,0.0766821311551601),
 .UNSPECIFIED.);
#586=B_SPLINE_CURVE_WITH_KNOTS('',3,(#27499,#27500,#27501,#27502),
 .UNSPECIFIED.,.F.,.F.,(4,4),(0.0319696744346128,0.0766821311551717),
 .UNSPECIFIED.);
#587=B_SPLINE_CURVE_WITH_KNOTS('',3,(#27525,#27526,#27527,#27528),
 .UNSPECIFIED.,.F.,.F.,(4,4),(0.165217092335982,0.177184346430046),
 .UNSPECIFIED.);
#588=B_SPLINE_CURVE_WITH_KNOTS('',3,(#27552,#27553,#27554,#27555),
 .UNSPECIFIED.,.F.,.F.,(4,4),(0.165217092335986,0.177184346430048),
 .UNSPECIFIED.);
#589=B_SPLINE_CURVE_WITH_KNOTS('',3,(#27556,#27557,#27558,#27559),
 .UNSPECIFIED.,.F.,.F.,(4,4),(0.077355308281931,0.0893225623759923),
 .UNSPECIFIED.);
#590=B_SPLINE_CURVE_WITH_KNOTS('',3,(#27572,#27573,#27574,#27575),
 .UNSPECIFIED.,.F.,.F.,(4,4),(0.,0.096444144720994),.UNSPECIFIED.);
#591=B_SPLINE_CURVE_WITH_KNOTS('',3,(#27577,#27578,#27579,#27580),
 .UNSPECIFIED.,.F.,.F.,(4,4),(-0.0893225623759868,-0.0773554379396859),
 .UNSPECIFIED.);
#592=B_SPLINE_CURVE_WITH_KNOTS('',3,(#27635,#27636,#27637,#27638),
 .UNSPECIFIED.,.F.,.F.,(4,4),(0.0319696744346056,0.0766821311551627),
 .UNSPECIFIED.);
#593=B_SPLINE_CURVE_WITH_KNOTS('',3,(#27673,#27674,#27675,#27676),
 .UNSPECIFIED.,.F.,.F.,(4,4),(0.0319696744346165,0.0766821311551601),
 .UNSPECIFIED.);
#594=B_SPLINE_CURVE_WITH_KNOTS('',3,(#27677,#27678,#27679,#27680),
 .UNSPECIFIED.,.F.,.F.,(4,4),(0.0319696744346167,0.0766821311551504),
 .UNSPECIFIED.);
#595=B_SPLINE_CURVE_WITH_KNOTS('',3,(#27715,#27716,#27717,#27718),
 .UNSPECIFIED.,.F.,.F.,(4,4),(0.031969674434606,0.0766821311551567),
 .UNSPECIFIED.);
#596=B_SPLINE_CURVE_WITH_KNOTS('',3,(#27719,#27720,#27721,#27722),
 .UNSPECIFIED.,.F.,.F.,(4,4),(0.0319696744346156,0.0766821311551527),
 .UNSPECIFIED.);
#597=B_SPLINE_CURVE_WITH_KNOTS('',3,(#27757,#27758,#27759,#27760),
 .UNSPECIFIED.,.F.,.F.,(4,4),(0.0319696744346135,0.0766821311551671),
 .UNSPECIFIED.);
#598=B_SPLINE_CURVE_WITH_KNOTS('',3,(#27761,#27762,#27763,#27764),
 .UNSPECIFIED.,.F.,.F.,(4,4),(0.0319696744346146,0.076682131155166),
 .UNSPECIFIED.);
#599=B_SPLINE_CURVE_WITH_KNOTS('',3,(#27799,#27800,#27801,#27802),
 .UNSPECIFIED.,.F.,.F.,(4,4),(0.0319696744346137,0.0766821311551702),
 .UNSPECIFIED.);
#600=B_SPLINE_CURVE_WITH_KNOTS('',3,(#27803,#27804,#27805,#27806),
 .UNSPECIFIED.,.F.,.F.,(4,4),(0.0319696744346153,0.0766821311551645),
 .UNSPECIFIED.);
#601=B_SPLINE_CURVE_WITH_KNOTS('',3,(#27841,#27842,#27843,#27844),
 .UNSPECIFIED.,.F.,.F.,(4,4),(0.0319696744346044,0.0766821311551661),
 .UNSPECIFIED.);
#602=B_SPLINE_CURVE_WITH_KNOTS('',3,(#27845,#27846,#27847,#27848),
 .UNSPECIFIED.,.F.,.F.,(4,4),(0.031969674434616,0.0766821311551596),
 .UNSPECIFIED.);
#603=B_SPLINE_CURVE_WITH_KNOTS('',3,(#27883,#27884,#27885,#27886),
 .UNSPECIFIED.,.F.,.F.,(4,4),(0.0319696744346171,0.0766821311551567),
 .UNSPECIFIED.);
#604=B_SPLINE_CURVE_WITH_KNOTS('',3,(#27887,#27888,#27889,#27890),
 .UNSPECIFIED.,.F.,.F.,(4,4),(0.0319696744346159,0.0766821311551545),
 .UNSPECIFIED.);
#605=B_SPLINE_CURVE_WITH_KNOTS('',3,(#27925,#27926,#27927,#27928),
 .UNSPECIFIED.,.F.,.F.,(4,4),(0.0319696744346147,0.0766821311551627),
 .UNSPECIFIED.);
#606=B_SPLINE_CURVE_WITH_KNOTS('',3,(#27929,#27930,#27931,#27932),
 .UNSPECIFIED.,.F.,.F.,(4,4),(0.031969674434614,0.0766821311551628),
 .UNSPECIFIED.);
#607=B_SPLINE_CURVE_WITH_KNOTS('',3,(#27967,#27968,#27969,#27970),
 .UNSPECIFIED.,.F.,.F.,(4,4),(0.0319696744346007,0.0766821311551619),
 .UNSPECIFIED.);
#608=B_SPLINE_CURVE_WITH_KNOTS('',3,(#27971,#27972,#27973,#27974),
 .UNSPECIFIED.,.F.,.F.,(4,4),(0.0319696744346149,0.0766821311551584),
 .UNSPECIFIED.);
#609=B_SPLINE_CURVE_WITH_KNOTS('',3,(#28090,#28091,#28092,#28093),
 .UNSPECIFIED.,.F.,.F.,(4,4),(0.,0.0964441447212768),.UNSPECIFIED.);
#610=B_SPLINE_CURVE_WITH_KNOTS('',3,(#28098,#28099,#28100,#28101),
 .UNSPECIFIED.,.F.,.F.,(4,4),(0.,0.0964441447214986),.UNSPECIFIED.);
#611=B_SPLINE_CURVE_WITH_KNOTS('',3,(#28102,#28103,#28104,#28105),
 .UNSPECIFIED.,.F.,.F.,(4,4),(0.336279561120233,0.34824668540691),
 .UNSPECIFIED.);
#612=B_SPLINE_CURVE_WITH_KNOTS('',3,(#28117,#28118,#28119,#28120),
 .UNSPECIFIED.,.F.,.F.,(4,4),(-0.0893225623759864,-0.0773554379396748),
 .UNSPECIFIED.);
#613=B_SPLINE_CURVE_WITH_KNOTS('',3,(#28129,#28130,#28131,#28132),
 .UNSPECIFIED.,.F.,.F.,(4,4),(0.,0.0964441447214225),.UNSPECIFIED.);
#614=B_SPLINE_CURVE_WITH_KNOTS('',3,(#28136,#28137,#28138,#28139),
 .UNSPECIFIED.,.F.,.F.,(4,4),(0.,0.096444144721337),.UNSPECIFIED.);
#615=B_SPLINE_CURVE_WITH_KNOTS('',3,(#28140,#28141,#28142,#28143),
 .UNSPECIFIED.,.F.,.F.,(4,4),(-0.0893225623759897,-0.0773554379396767),
 .UNSPECIFIED.);
#616=B_SPLINE_CURVE_WITH_KNOTS('',3,(#28150,#28151,#28152,#28153),
 .UNSPECIFIED.,.F.,.F.,(4,4),(-0.177184216772303,-0.165217092335987),
 .UNSPECIFIED.);
#617=B_SPLINE_CURVE_WITH_KNOTS('',3,(#28162,#28163,#28164,#28165),
 .UNSPECIFIED.,.F.,.F.,(4,4),(0.,0.0964441447210733),.UNSPECIFIED.);
#618=B_SPLINE_CURVE_WITH_KNOTS('',3,(#28170,#28171,#28172,#28173),
 .UNSPECIFIED.,.F.,.F.,(4,4),(0.,0.0964441447210223),.UNSPECIFIED.);
#619=B_SPLINE_CURVE_WITH_KNOTS('',3,(#28174,#28175,#28176,#28177),
 .UNSPECIFIED.,.F.,.F.,(4,4),(-0.177184216772304,-0.165217092335993),
 .UNSPECIFIED.);
#620=B_SPLINE_CURVE_WITH_KNOTS('',3,(#28189,#28190,#28191,#28192),
 .UNSPECIFIED.,.F.,.F.,(4,4),(-0.0893225623759886,-0.0773554379396872),
 .UNSPECIFIED.);
#621=B_SPLINE_CURVE_WITH_KNOTS('',3,(#28201,#28202,#28203,#28204),
 .UNSPECIFIED.,.F.,.F.,(4,4),(0.,0.0964441447215364),.UNSPECIFIED.);
#622=B_SPLINE_CURVE_WITH_KNOTS('',3,(#28208,#28209,#28210,#28211),
 .UNSPECIFIED.,.F.,.F.,(4,4),(0.,0.0964441447215273),.UNSPECIFIED.);
#623=B_SPLINE_CURVE_WITH_KNOTS('',3,(#28212,#28213,#28214,#28215),
 .UNSPECIFIED.,.F.,.F.,(4,4),(-0.0893225623759895,-0.077355437939685),
 .UNSPECIFIED.);
#624=B_SPLINE_CURVE_WITH_KNOTS('',3,(#28222,#28223,#28224,#28225),
 .UNSPECIFIED.,.F.,.F.,(4,4),(-0.177184216772292,-0.165217092335987),
 .UNSPECIFIED.);
#625=B_SPLINE_CURVE_WITH_KNOTS('',3,(#28234,#28235,#28236,#28237),
 .UNSPECIFIED.,.F.,.F.,(4,4),(0.,0.0964441447214411),.UNSPECIFIED.);
#626=B_SPLINE_CURVE_WITH_KNOTS('',3,(#28242,#28243,#28244,#28245),
 .UNSPECIFIED.,.F.,.F.,(4,4),(0.,0.0964441447215376),.UNSPECIFIED.);
#627=B_SPLINE_CURVE_WITH_KNOTS('',3,(#28246,#28247,#28248,#28249),
 .UNSPECIFIED.,.F.,.F.,(4,4),(-0.177184216772293,-0.165217092335991),
 .UNSPECIFIED.);
#628=B_SPLINE_CURVE_WITH_KNOTS('',3,(#28261,#28262,#28263,#28264),
 .UNSPECIFIED.,.F.,.F.,(4,4),(-0.0893225623759893,-0.0773554379396748),
 .UNSPECIFIED.);
#629=B_SPLINE_CURVE_WITH_KNOTS('',3,(#28270,#28271,#28272,#28273),
 .UNSPECIFIED.,.F.,.F.,(4,4),(0.,0.0964441447215519),.UNSPECIFIED.);
#630=B_SPLINE_CURVE_WITH_KNOTS('',3,(#28277,#28278,#28279,#28280),
 .UNSPECIFIED.,.F.,.F.,(4,4),(0.,0.0964441447216442),.UNSPECIFIED.);
#855=CONICAL_SURFACE('',#17328,53.25,0.785398163397446);
#856=CONICAL_SURFACE('',#17334,53.25,0.785398163397446);
#857=CONICAL_SURFACE('',#17341,0.950000000000001,0.785398163397444);
#858=CONICAL_SURFACE('',#17350,0.950000000000001,0.785398163397445);
#859=CONICAL_SURFACE('',#17353,0.950000000000004,0.785398163397449);
#860=CONICAL_SURFACE('',#17364,53.25,0.785398163397446);
#861=CONICAL_SURFACE('',#17371,53.25,0.785398163397446);
#862=CONICAL_SURFACE('',#17374,53.25,0.785398163397446);
#863=CONICAL_SURFACE('',#17381,53.25,0.785398163397455);
#864=CONICAL_SURFACE('',#17388,53.25,0.785398163397446);
#865=CONICAL_SURFACE('',#17395,53.25,0.785398163397446);
#866=CONICAL_SURFACE('',#17402,53.25,0.785398163397446);
#867=CONICAL_SURFACE('',#17409,53.25,0.785398163397446);
#868=CONICAL_SURFACE('',#17416,53.25,0.785398163397446);
#869=CONICAL_SURFACE('',#17423,53.25,0.785398163397446);
#870=CONICAL_SURFACE('',#17429,0.950000000000002,0.785398163397447);
#871=CONICAL_SURFACE('',#17432,53.25,0.785398163397437);
#872=CONICAL_SURFACE('',#17435,53.25,0.785398163397455);
#873=CONICAL_SURFACE('',#17438,53.25,0.785398163397437);
#874=CONICAL_SURFACE('',#17606,0.950000000000002,0.785398163397447);
#875=CONICAL_SURFACE('',#17612,0.950000000000002,0.785398163397446);
#876=CONICAL_SURFACE('',#17618,0.950000000000005,0.785398163397452);
#877=CONICAL_SURFACE('',#17626,53.25,0.785398163397446);
#878=CONICAL_SURFACE('',#17629,53.25,0.785398163397437);
#879=CONICAL_SURFACE('',#17635,53.25,0.785398163397446);
#880=CONICAL_SURFACE('',#17641,53.25,0.785398163397446);
#881=CONICAL_SURFACE('',#17647,53.25,0.785398163397446);
#882=CONICAL_SURFACE('',#17653,53.25,0.785398163397455);
#883=CONICAL_SURFACE('',#17659,53.25,0.785398163397437);
#884=CONICAL_SURFACE('',#17664,53.25,0.785398163397437);
#885=CONICAL_SURFACE('',#17666,53.25,0.785398163397446);
#886=CONICAL_SURFACE('',#17668,53.25,0.785398163397437);
#887=CONICAL_SURFACE('',#17677,0.950000000000005,0.785398163397451);
#888=CONICAL_SURFACE('',#17679,0.950000000000004,0.78539816339745);
#889=CONICAL_SURFACE('',#17681,0.950000000000002,0.785398163397445);
#890=CONICAL_SURFACE('',#17683,0.950000000000003,0.785398163397449);
#891=CONICAL_SURFACE('',#17685,0.950000000000004,0.78539816339745);
#892=CONICAL_SURFACE('',#17700,0.950000000000005,0.785398163397451);
#893=CONICAL_SURFACE('',#17705,53.25,0.785398163397437);
#894=CONICAL_SURFACE('',#17708,0.950000000000001,0.785398163397444);
#895=CONICAL_SURFACE('',#17714,0.950000000000003,0.785398163397448);
#896=CONICAL_SURFACE('',#17720,0.950000000000003,0.785398163397447);
#897=CONICAL_SURFACE('',#17728,53.25,0.785398163397437);
#898=CONICAL_SURFACE('',#17731,53.25,0.785398163397437);
#899=CONICAL_SURFACE('',#17737,53.25,0.785398163397446);
#900=CONICAL_SURFACE('',#17743,53.25,0.785398163397446);
#901=CONICAL_SURFACE('',#17749,53.25,0.785398163397446);
#902=CONICAL_SURFACE('',#17755,53.25,0.785398163397446);
#903=CONICAL_SURFACE('',#17760,53.25,0.785398163397446);
#904=CONICAL_SURFACE('',#17762,53.25,0.785398163397437);
#905=CONICAL_SURFACE('',#17764,53.25,0.785398163397437);
#906=CONICAL_SURFACE('',#17775,0.950000000000002,0.785398163397446);
#907=CONICAL_SURFACE('',#17777,0.950000000000002,0.785398163397447);
#908=CONICAL_SURFACE('',#17779,0.950000000000003,0.785398163397448);
#909=CONICAL_SURFACE('',#17781,0.950000000000001,0.785398163397444);
#910=CONICAL_SURFACE('',#17794,0.950000000000002,0.785398163397447);
#911=CONICAL_SURFACE('',#17800,0.950000000000004,0.78539816339745);
#912=CONICAL_SURFACE('',#17806,0.950000000000003,0.785398163397449);
#913=CONICAL_SURFACE('',#17812,0.950000000000002,0.785398163397445);
#914=CONICAL_SURFACE('',#17818,0.950000000000004,0.78539816339745);
#915=CONICAL_SURFACE('',#17826,53.25,0.785398163397446);
#916=CONICAL_SURFACE('',#17829,53.25,0.785398163397446);
#917=CONICAL_SURFACE('',#17835,53.25,0.785398163397446);
#918=CONICAL_SURFACE('',#17841,53.25,0.785398163397446);
#919=CONICAL_SURFACE('',#17847,53.25,0.785398163397446);
#920=CONICAL_SURFACE('',#17852,53.25,0.785398163397446);
#921=CONICAL_SURFACE('',#17854,53.25,0.785398163397446);
#922=CONICAL_SURFACE('',#17856,53.25,0.785398163397455);
#923=CONICAL_SURFACE('',#17858,53.25,0.785398163397446);
#924=CONICAL_SURFACE('',#17860,53.25,0.785398163397446);
#925=CONICAL_SURFACE('',#17873,0.950000000000003,0.785398163397447);
#926=CONICAL_SURFACE('',#17875,0.950000000000005,0.785398163397452);
#927=CONICAL_SURFACE('',#17877,0.950000000000002,0.785398163397446);
#928=CONICAL_SURFACE('',#17888,0.950000000000001,0.785398163397445);
#929=CONICAL_SURFACE('',#17893,53.25,0.785398163397437);
#930=CONICAL_SURFACE('',#17896,0.950000000000003,0.785398163397449);
#931=CONICAL_SURFACE('',#17902,0.950000000000001,0.785398163397444);
#932=CONICAL_SURFACE('',#17908,0.950000000000004,0.785398163397449);
#933=CONICAL_SURFACE('',#17914,0.950000000000004,0.78539816339745);
#934=CONICAL_SURFACE('',#17920,0.950000000000001,0.785398163397444);
#935=CONICAL_SURFACE('',#17928,53.25,0.785398163397446);
#936=CONICAL_SURFACE('',#17931,53.25,0.785398163397437);
#937=CONICAL_SURFACE('',#17937,53.25,0.785398163397446);
#938=CONICAL_SURFACE('',#17943,53.25,0.785398163397455);
#939=CONICAL_SURFACE('',#17948,53.25,0.785398163397455);
#940=CONICAL_SURFACE('',#17950,53.25,0.785398163397437);
#941=CONICAL_SURFACE('',#17952,53.25,0.785398163397437);
#942=CONICAL_SURFACE('',#17954,53.25,0.785398163397446);
#943=CONICAL_SURFACE('',#17956,53.25,0.785398163397455);
#944=CONICAL_SURFACE('',#17971,0.950000000000003,0.785398163397448);
#945=CONICAL_SURFACE('',#17973,0.950000000000001,0.785398163397445);
#946=CONICAL_SURFACE('',#17982,0.950000000000002,0.785398163397446);
#947=CONICAL_SURFACE('',#17988,0.950000000000004,0.78539816339745);
#948=CONICAL_SURFACE('',#17994,0.950000000000002,0.785398163397447);
#949=CONICAL_SURFACE('',#18000,0.950000000000002,0.785398163397445);
#950=CONICAL_SURFACE('',#18006,0.950000000000001,0.785398163397444);
#951=CONICAL_SURFACE('',#18012,0.950000000000004,0.78539816339745);
#952=CONICAL_SURFACE('',#18018,0.950000000000004,0.78539816339745);
#953=CONICAL_SURFACE('',#18026,53.25,0.785398163397437);
#954=CONICAL_SURFACE('',#18029,53.25,0.785398163397446);
#955=CONICAL_SURFACE('',#18035,53.25,0.785398163397446);
#956=CONICAL_SURFACE('',#18040,53.25,0.785398163397446);
#957=CONICAL_SURFACE('',#18042,53.25,0.785398163397446);
#958=CONICAL_SURFACE('',#18044,53.25,0.785398163397437);
#959=CONICAL_SURFACE('',#18046,53.25,0.785398163397446);
#960=CONICAL_SURFACE('',#18048,53.25,0.785398163397437);
#961=CONICAL_SURFACE('',#18050,53.25,0.785398163397446);
#962=CONICAL_SURFACE('',#18052,53.25,0.785398163397446);
#963=CONICAL_SURFACE('',#18069,0.950000000000002,0.785398163397447);
#964=CONICAL_SURFACE('',#18076,0.950000000000001,0.785398163397444);
#965=CONICAL_SURFACE('',#18082,0.950000000000003,0.785398163397448);
#966=CONICAL_SURFACE('',#18088,0.950000000000003,0.785398163397447);
#967=CONICAL_SURFACE('',#18094,0.950000000000002,0.785398163397446);
#968=CONICAL_SURFACE('',#18100,0.950000000000005,0.785398163397452);
#969=CONICAL_SURFACE('',#18106,0.950000000000004,0.78539816339745);
#970=CONICAL_SURFACE('',#18112,0.950000000000002,0.785398163397445);
#971=CONICAL_SURFACE('',#18118,0.950000000000003,0.785398163397449);
#972=CONICAL_SURFACE('',#18126,53.25,0.785398163397455);
#973=CONICAL_SURFACE('',#18129,53.25,0.785398163397446);
#974=CONICAL_SURFACE('',#18134,53.25,0.785398163397437);
#975=CONICAL_SURFACE('',#18136,53.25,0.785398163397437);
#976=CONICAL_SURFACE('',#18138,53.25,0.785398163397446);
#977=CONICAL_SURFACE('',#18140,53.25,0.785398163397437);
#978=CONICAL_SURFACE('',#18142,53.25,0.785398163397446);
#979=CONICAL_SURFACE('',#18144,53.25,0.785398163397446);
#980=CONICAL_SURFACE('',#18146,53.25,0.785398163397446);
#981=CONICAL_SURFACE('',#18148,53.25,0.785398163397446);
#982=CONICAL_SURFACE('',#18170,53.25,0.785398163397446);
#983=CONICAL_SURFACE('',#18176,53.25,0.785398163397446);
#984=CONICAL_SURFACE('',#18182,53.25,0.785398163397446);
#985=CONICAL_SURFACE('',#18188,53.25,0.785398163397446);
#986=CONICAL_SURFACE('',#18194,53.25,0.785398163397446);
#987=CONICAL_SURFACE('',#18200,53.25,0.785398163397437);
#988=CONICAL_SURFACE('',#18206,53.25,0.785398163397446);
#989=CONICAL_SURFACE('',#18212,53.25,0.785398163397446);
#990=CONICAL_SURFACE('',#18218,53.25,0.785398163397446);
#991=CONICAL_SURFACE('',#18226,0.950000000000001,0.785398163397444);
#992=CONICAL_SURFACE('',#18228,0.950000000000004,0.78539816339745);
#993=CONICAL_SURFACE('',#18230,0.950000000000003,0.785398163397449);
#994=CONICAL_SURFACE('',#18232,0.950000000000002,0.785398163397445);
#995=CONICAL_SURFACE('',#18234,0.950000000000004,0.78539816339745);
#996=CONICAL_SURFACE('',#18236,0.950000000000005,0.785398163397452);
#997=CONICAL_SURFACE('',#18238,0.950000000000002,0.785398163397446);
#998=CONICAL_SURFACE('',#18240,0.950000000000003,0.785398163397447);
#999=CONICAL_SURFACE('',#18242,0.950000000000003,0.785398163397448);
#1000=CONICAL_SURFACE('',#18260,49.75,0.785398163397446);
#1001=CONICAL_SURFACE('',#18265,0.950000000000004,0.78539816339745);
#1002=CONICAL_SURFACE('',#18267,0.950000000000004,0.78539816339745);
#1003=CONICAL_SURFACE('',#18269,0.950000000000001,0.785398163397444);
#1004=CONICAL_SURFACE('',#18271,0.950000000000001,0.785398163397445);
#1005=CONICAL_SURFACE('',#18273,0.950000000000002,0.785398163397447);
#1006=CONICAL_SURFACE('',#18275,0.950000000000004,0.78539816339745);
#1007=CONICAL_SURFACE('',#18277,0.950000000000002,0.785398163397446);
#1008=CONICAL_SURFACE('',#18279,0.950000000000002,0.785398163397447);
#1009=CONICAL_SURFACE('',#18303,53.25,0.785398163397437);
#1010=CONICAL_SURFACE('',#18309,53.25,0.785398163397446);
#1011=CONICAL_SURFACE('',#18315,53.25,0.785398163397437);
#1012=CONICAL_SURFACE('',#18321,53.25,0.785398163397455);
#1013=CONICAL_SURFACE('',#18327,53.25,0.785398163397446);
#1014=CONICAL_SURFACE('',#18333,53.25,0.785398163397455);
#1015=CONICAL_SURFACE('',#18336,52.6267766952966,1.17809724509617);
#1016=CONICAL_SURFACE('',#18341,53.1,0.785398163397448);
#1017=CONICAL_SURFACE('',#18443,12.7,0.785398163397448);
#1018=CONICAL_SURFACE('',#18455,12.7,0.785398163397448);
#1019=CONICAL_SURFACE('',#18459,12.7,0.785398163397448);
#1020=CONICAL_SURFACE('',#18463,12.7,0.785398163397448);
#1021=CONICAL_SURFACE('',#18467,12.7,0.785398163397448);
#1022=CONICAL_SURFACE('',#18471,50.8,0.785398163397444);
#1023=CONICAL_SURFACE('',#18586,1.5,0.785398163397448);
#1024=CONICAL_SURFACE('',#18588,1.5,0.785398163397448);
#1025=CONICAL_SURFACE('',#18590,1.5,0.785398163397448);
#1026=CONICAL_SURFACE('',#18592,1.5,0.785398163397448);
#1027=CONICAL_SURFACE('',#18594,1.5,0.785398163397448);
#1053=(
BOUNDED_CURVE()
B_SPLINE_CURVE(2,(#23997,#23998,#23999),.UNSPECIFIED.,.F.,.F.)
B_SPLINE_CURVE_WITH_KNOTS((3,3),(0.014211217125653,0.110567648737549),
 .UNSPECIFIED.)
CURVE()
GEOMETRIC_REPRESENTATION_ITEM()
RATIONAL_B_SPLINE_CURVE((1.00000961767885,1.00003742651076,1.00000019074343))
REPRESENTATION_ITEM('')
);
#1054=(
BOUNDED_CURVE()
B_SPLINE_CURVE(2,(#24024,#24025,#24026),.UNSPECIFIED.,.F.,.F.)
B_SPLINE_CURVE_WITH_KNOTS((3,3),(0.000246247416175969,0.0445514940289779),
 .UNSPECIFIED.)
CURVE()
GEOMETRIC_REPRESENTATION_ITEM()
RATIONAL_B_SPLINE_CURVE((1.00000019074342,1.00001731196463,1.00002068136762))
REPRESENTATION_ITEM('')
);
#1055=(
BOUNDED_CURVE()
B_SPLINE_CURVE(2,(#24030,#24031,#24032),.UNSPECIFIED.,.F.,.F.)
B_SPLINE_CURVE_WITH_KNOTS((3,3),(0.0662613029802821,0.11056581047863),
 .UNSPECIFIED.)
CURVE()
GEOMETRIC_REPRESENTATION_ITEM()
RATIONAL_B_SPLINE_CURVE((1.00002056800856,1.00001716071035,1.00000000159957))
REPRESENTATION_ITEM('')
);
#1056=(
BOUNDED_CURVE()
B_SPLINE_CURVE(2,(#24039,#24040,#24041),.UNSPECIFIED.,.F.,.F.)
B_SPLINE_CURVE_WITH_KNOTS((3,3),(7.8655962319518E-6,0.0612396373727806),
 .UNSPECIFIED.)
CURVE()
GEOMETRIC_REPRESENTATION_ITEM()
RATIONAL_B_SPLINE_CURVE((1.0000191574532,1.07458139657232,1.05821963517917))
REPRESENTATION_ITEM('')
);
#1057=(
BOUNDED_CURVE()
B_SPLINE_CURVE(2,(#24061,#24062,#24063),.UNSPECIFIED.,.F.,.F.)
B_SPLINE_CURVE_WITH_KNOTS((3,3),(0.000246247416178877,0.0966026790274259),
 .UNSPECIFIED.)
CURVE()
GEOMETRIC_REPRESENTATION_ITEM()
RATIONAL_B_SPLINE_CURVE((1.00000019074342,1.00003742650866,1.00000961767831))
REPRESENTATION_ITEM('')
);
#1058=(
BOUNDED_CURVE()
B_SPLINE_CURVE(2,(#24082,#24083,#24084),.UNSPECIFIED.,.F.,.F.)
B_SPLINE_CURVE_WITH_KNOTS((3,3),(0.0660091927117484,0.110314456526714),
 .UNSPECIFIED.)
CURVE()
GEOMETRIC_REPRESENTATION_ITEM()
RATIONAL_B_SPLINE_CURVE((1.00002048940956,1.0000171214116,1.00000000159591))
REPRESENTATION_ITEM('')
);
#1059=(
BOUNDED_CURVE()
B_SPLINE_CURVE(2,(#24091,#24092,#24093),.UNSPECIFIED.,.F.,.F.)
B_SPLINE_CURVE_WITH_KNOTS((3,3),(7.86559624534418E-6,0.0612396373727898),
 .UNSPECIFIED.)
CURVE()
GEOMETRIC_REPRESENTATION_ITEM()
RATIONAL_B_SPLINE_CURVE((1.00001915745323,1.07458139657225,1.05821963517912))
REPRESENTATION_ITEM('')
);
#1060=(
BOUNDED_CURVE()
B_SPLINE_CURVE(2,(#24098,#24099,#24100),.UNSPECIFIED.,.F.,.F.)
B_SPLINE_CURVE_WITH_KNOTS((3,3),(0.039202339545078,0.100434111321632),
 .UNSPECIFIED.)
CURVE()
GEOMETRIC_REPRESENTATION_ITEM()
RATIONAL_B_SPLINE_CURVE((1.05821963517908,1.0745813965722,1.00001915745321))
REPRESENTATION_ITEM('')
);
#1061=(
BOUNDED_CURVE()
B_SPLINE_CURVE(2,(#24123,#24124,#24125),.UNSPECIFIED.,.F.,.F.)
B_SPLINE_CURVE_WITH_KNOTS((3,3),(2.06502885214965E-6,0.0443073288438628),
 .UNSPECIFIED.)
CURVE()
GEOMETRIC_REPRESENTATION_ITEM()
RATIONAL_B_SPLINE_CURVE((1.00000000159591,1.00001712140826,1.00002048940556))
REPRESENTATION_ITEM('')
);
#1062=(
BOUNDED_CURVE()
B_SPLINE_CURVE(2,(#24127,#24128,#24129),.UNSPECIFIED.,.F.,.F.)
B_SPLINE_CURVE_WITH_KNOTS((3,3),(0.0392023395450862,0.100434111321651),
 .UNSPECIFIED.)
CURVE()
GEOMETRIC_REPRESENTATION_ITEM()
RATIONAL_B_SPLINE_CURVE((1.0582196351792,1.07458139657236,1.00001915745321))
REPRESENTATION_ITEM('')
);
#1063=(
BOUNDED_CURVE()
B_SPLINE_CURVE(2,(#24144,#24145,#24146),.UNSPECIFIED.,.F.,.F.)
B_SPLINE_CURVE_WITH_KNOTS((3,3),(0.0660091927116512,0.110314456526713),
 .UNSPECIFIED.)
CURVE()
GEOMETRIC_REPRESENTATION_ITEM()
RATIONAL_B_SPLINE_CURVE((1.00002048940626,1.00001712140884,1.00000000159591))
REPRESENTATION_ITEM('')
);
#1064=(
BOUNDED_CURVE()
B_SPLINE_CURVE(2,(#24153,#24154,#24155),.UNSPECIFIED.,.F.,.F.)
B_SPLINE_CURVE_WITH_KNOTS((3,3),(7.86559624825463E-6,0.0612396373727913),
 .UNSPECIFIED.)
CURVE()
GEOMETRIC_REPRESENTATION_ITEM()
RATIONAL_B_SPLINE_CURVE((1.00001915745324,1.07458139657224,1.0582196351791))
REPRESENTATION_ITEM('')
);
#1065=(
BOUNDED_CURVE()
B_SPLINE_CURVE(2,(#24160,#24161,#24162),.UNSPECIFIED.,.F.,.F.)
B_SPLINE_CURVE_WITH_KNOTS((3,3),(0.0392023395450792,0.100434111321637),
 .UNSPECIFIED.)
CURVE()
GEOMETRIC_REPRESENTATION_ITEM()
RATIONAL_B_SPLINE_CURVE((1.05821963517906,1.07458139657217,1.00001915745318))
REPRESENTATION_ITEM('')
);
#1066=(
BOUNDED_CURVE()
B_SPLINE_CURVE(2,(#24183,#24184,#24185),.UNSPECIFIED.,.F.,.F.)
B_SPLINE_CURVE_WITH_KNOTS((3,3),(2.06502885258463E-6,0.0443073288438806),
 .UNSPECIFIED.)
CURVE()
GEOMETRIC_REPRESENTATION_ITEM()
RATIONAL_B_SPLINE_CURVE((1.00000000159591,1.00001712141144,1.00002048940937))
REPRESENTATION_ITEM('')
);
#1067=(
BOUNDED_CURVE()
B_SPLINE_CURVE(2,(#24191,#24192,#24193),.UNSPECIFIED.,.F.,.F.)
B_SPLINE_CURVE_WITH_KNOTS((3,3),(2.06499351918632E-6,0.0443065724919368),
 .UNSPECIFIED.)
CURVE()
GEOMETRIC_REPRESENTATION_ITEM()
RATIONAL_B_SPLINE_CURVE((1.00000000159957,1.00001716071329,1.00002056801208))
REPRESENTATION_ITEM('')
);
#1068=(
BOUNDED_CURVE()
B_SPLINE_CURVE(2,(#24201,#24202,#24203),.UNSPECIFIED.,.F.,.F.)
B_SPLINE_CURVE_WITH_KNOTS((3,3),(0.000246247280288311,0.0966026259860039),
 .UNSPECIFIED.)
CURVE()
GEOMETRIC_REPRESENTATION_ITEM()
RATIONAL_B_SPLINE_CURVE((1.00000019075751,1.00003742928082,1.00000962320604))
REPRESENTATION_ITEM('')
);
#1069=(
BOUNDED_CURVE()
B_SPLINE_CURVE(2,(#24238,#24239,#24240),.UNSPECIFIED.,.F.,.F.)
B_SPLINE_CURVE_WITH_KNOTS((3,3),(0.0662687847811497,0.110573269834419),
 .UNSPECIFIED.)
CURVE()
GEOMETRIC_REPRESENTATION_ITEM()
RATIONAL_B_SPLINE_CURVE((1.00002057035038,1.00001716188432,1.00000000159968))
REPRESENTATION_ITEM('')
);
#1070=(
BOUNDED_CURVE()
B_SPLINE_CURVE(2,(#24247,#24248,#24249),.UNSPECIFIED.,.F.,.F.)
B_SPLINE_CURVE_WITH_KNOTS((3,3),(7.86559623378178E-6,0.0612396373727884),
 .UNSPECIFIED.)
CURVE()
GEOMETRIC_REPRESENTATION_ITEM()
RATIONAL_B_SPLINE_CURVE((1.00001915745321,1.07458139657226,1.05821963517913))
REPRESENTATION_ITEM('')
);
#1071=(
BOUNDED_CURVE()
B_SPLINE_CURVE(2,(#24280,#24281,#24282),.UNSPECIFIED.,.F.,.F.)
B_SPLINE_CURVE_WITH_KNOTS((3,3),(2.06502884978116E-6,0.0443073288439222),
 .UNSPECIFIED.)
CURVE()
GEOMETRIC_REPRESENTATION_ITEM()
RATIONAL_B_SPLINE_CURVE((1.00000000159591,1.0000171214099,1.00002048940752))
REPRESENTATION_ITEM('')
);
#1072=(
BOUNDED_CURVE()
B_SPLINE_CURVE(2,(#24284,#24285,#24286),.UNSPECIFIED.,.F.,.F.)
B_SPLINE_CURVE_WITH_KNOTS((3,3),(0.0392023395450863,0.100434111321653),
 .UNSPECIFIED.)
CURVE()
GEOMETRIC_REPRESENTATION_ITEM()
RATIONAL_B_SPLINE_CURVE((1.0582196351792,1.07458139657235,1.00001915745318))
REPRESENTATION_ITEM('')
);
#1073=(
BOUNDED_CURVE()
B_SPLINE_CURVE(2,(#24292,#24293,#24294),.UNSPECIFIED.,.F.,.F.)
B_SPLINE_CURVE_WITH_KNOTS((3,3),(0.0660091927117005,0.110314456526681),
 .UNSPECIFIED.)
CURVE()
GEOMETRIC_REPRESENTATION_ITEM()
RATIONAL_B_SPLINE_CURVE((1.00002048940979,1.0000171214118,1.00000000159591))
REPRESENTATION_ITEM('')
);
#1074=(
BOUNDED_CURVE()
B_SPLINE_CURVE(2,(#24315,#24316,#24317),.UNSPECIFIED.,.F.,.F.)
B_SPLINE_CURVE_WITH_KNOTS((3,3),(7.86559623866961E-6,0.0612396373727917),
 .UNSPECIFIED.)
CURVE()
GEOMETRIC_REPRESENTATION_ITEM()
RATIONAL_B_SPLINE_CURVE((1.00001915745322,1.07458139657226,1.05821963517913))
REPRESENTATION_ITEM('')
);
#1075=(
BOUNDED_CURVE()
B_SPLINE_CURVE(2,(#24325,#24326,#24327),.UNSPECIFIED.,.F.,.F.)
B_SPLINE_CURVE_WITH_KNOTS((3,3),(2.06502884929736E-6,0.0443073288439272),
 .UNSPECIFIED.)
CURVE()
GEOMETRIC_REPRESENTATION_ITEM()
RATIONAL_B_SPLINE_CURVE((1.00000000159591,1.0000171214054,1.00002048940214))
REPRESENTATION_ITEM('')
);
#1076=(
BOUNDED_CURVE()
B_SPLINE_CURVE(2,(#24329,#24330,#24331),.UNSPECIFIED.,.F.,.F.)
B_SPLINE_CURVE_WITH_KNOTS((3,3),(0.0392023395450894,0.100434111321656),
 .UNSPECIFIED.)
CURVE()
GEOMETRIC_REPRESENTATION_ITEM()
RATIONAL_B_SPLINE_CURVE((1.05821963517919,1.07458139657234,1.00001915745318))
REPRESENTATION_ITEM('')
);
#1077=(
BOUNDED_CURVE()
B_SPLINE_CURVE(2,(#24337,#24338,#24339),.UNSPECIFIED.,.F.,.F.)
B_SPLINE_CURVE_WITH_KNOTS((3,3),(0.066009192711667,0.110314456526716),
 .UNSPECIFIED.)
CURVE()
GEOMETRIC_REPRESENTATION_ITEM()
RATIONAL_B_SPLINE_CURVE((1.00002048940695,1.00001712140941,1.00000000159591))
REPRESENTATION_ITEM('')
);
#1078=(
BOUNDED_CURVE()
B_SPLINE_CURVE(2,(#24360,#24361,#24362),.UNSPECIFIED.,.F.,.F.)
B_SPLINE_CURVE_WITH_KNOTS((3,3),(7.86559624154099E-6,0.061239637372789),
 .UNSPECIFIED.)
CURVE()
GEOMETRIC_REPRESENTATION_ITEM()
RATIONAL_B_SPLINE_CURVE((1.00001915745323,1.07458139657237,1.05821963517921))
REPRESENTATION_ITEM('')
);
#1079=(
BOUNDED_CURVE()
B_SPLINE_CURVE(2,(#24370,#24371,#24372),.UNSPECIFIED.,.F.,.F.)
B_SPLINE_CURVE_WITH_KNOTS((3,3),(2.06502884995711E-6,0.0443073288438823),
 .UNSPECIFIED.)
CURVE()
GEOMETRIC_REPRESENTATION_ITEM()
RATIONAL_B_SPLINE_CURVE((1.00000000159591,1.00001712141098,1.00002048940882))
REPRESENTATION_ITEM('')
);
#1080=(
BOUNDED_CURVE()
B_SPLINE_CURVE(2,(#24374,#24375,#24376),.UNSPECIFIED.,.F.,.F.)
B_SPLINE_CURVE_WITH_KNOTS((3,3),(0.0392023395450777,0.100434111321635),
 .UNSPECIFIED.)
CURVE()
GEOMETRIC_REPRESENTATION_ITEM()
RATIONAL_B_SPLINE_CURVE((1.05821963517909,1.07458139657222,1.0000191574532))
REPRESENTATION_ITEM('')
);
#1081=(
BOUNDED_CURVE()
B_SPLINE_CURVE(2,(#24382,#24383,#24384),.UNSPECIFIED.,.F.,.F.)
B_SPLINE_CURVE_WITH_KNOTS((3,3),(0.066009192711704,0.110314456526683),
 .UNSPECIFIED.)
CURVE()
GEOMETRIC_REPRESENTATION_ITEM()
RATIONAL_B_SPLINE_CURVE((1.0000204894117,1.00001712141339,1.00000000159591))
REPRESENTATION_ITEM('')
);
#1082=(
BOUNDED_CURVE()
B_SPLINE_CURVE(2,(#24405,#24406,#24407),.UNSPECIFIED.,.F.,.F.)
B_SPLINE_CURVE_WITH_KNOTS((3,3),(7.86559624762531E-6,0.0612396373728004),
 .UNSPECIFIED.)
CURVE()
GEOMETRIC_REPRESENTATION_ITEM()
RATIONAL_B_SPLINE_CURVE((1.00001915745324,1.07458139657236,1.0582196351792))
REPRESENTATION_ITEM('')
);
#1083=(
BOUNDED_CURVE()
B_SPLINE_CURVE(2,(#24415,#24416,#24417),.UNSPECIFIED.,.F.,.F.)
B_SPLINE_CURVE_WITH_KNOTS((3,3),(2.06502884960702E-6,0.0443073288440253),
 .UNSPECIFIED.)
CURVE()
GEOMETRIC_REPRESENTATION_ITEM()
RATIONAL_B_SPLINE_CURVE((1.00000000159591,1.00001712140153,1.00002048939751))
REPRESENTATION_ITEM('')
);
#1084=(
BOUNDED_CURVE()
B_SPLINE_CURVE(2,(#24419,#24420,#24421),.UNSPECIFIED.,.F.,.F.)
B_SPLINE_CURVE_WITH_KNOTS((3,3),(0.0392023395450754,0.100434111321632),
 .UNSPECIFIED.)
CURVE()
GEOMETRIC_REPRESENTATION_ITEM()
RATIONAL_B_SPLINE_CURVE((1.05821963517911,1.07458139657224,1.00001915745321))
REPRESENTATION_ITEM('')
);
#1085=(
BOUNDED_CURVE()
B_SPLINE_CURVE(2,(#24427,#24428,#24429),.UNSPECIFIED.,.F.,.F.)
B_SPLINE_CURVE_WITH_KNOTS((3,3),(0.066009192711622,0.110314456526713),
 .UNSPECIFIED.)
CURVE()
GEOMETRIC_REPRESENTATION_ITEM()
RATIONAL_B_SPLINE_CURVE((1.00002048940407,1.00001712140701,1.00000000159591))
REPRESENTATION_ITEM('')
);
#1086=(
BOUNDED_CURVE()
B_SPLINE_CURVE(2,(#24450,#24451,#24452),.UNSPECIFIED.,.F.,.F.)
B_SPLINE_CURVE_WITH_KNOTS((3,3),(7.86559623771071E-6,0.0612396373727852),
 .UNSPECIFIED.)
CURVE()
GEOMETRIC_REPRESENTATION_ITEM()
RATIONAL_B_SPLINE_CURVE((1.00001915745322,1.07458139657238,1.05821963517921))
REPRESENTATION_ITEM('')
);
#1087=(
BOUNDED_CURVE()
B_SPLINE_CURVE(2,(#24460,#24461,#24462),.UNSPECIFIED.,.F.,.F.)
B_SPLINE_CURVE_WITH_KNOTS((3,3),(2.06502884816085E-6,0.0443073288439097),
 .UNSPECIFIED.)
CURVE()
GEOMETRIC_REPRESENTATION_ITEM()
RATIONAL_B_SPLINE_CURVE((1.00000000159591,1.00001712140925,1.00002048940675))
REPRESENTATION_ITEM('')
);
#1088=(
BOUNDED_CURVE()
B_SPLINE_CURVE(2,(#24464,#24465,#24466),.UNSPECIFIED.,.F.,.F.)
B_SPLINE_CURVE_WITH_KNOTS((3,3),(0.0392023395450782,0.100434111321637),
 .UNSPECIFIED.)
CURVE()
GEOMETRIC_REPRESENTATION_ITEM()
RATIONAL_B_SPLINE_CURVE((1.05821963517907,1.07458139657219,1.00001915745318))
REPRESENTATION_ITEM('')
);
#1089=(
BOUNDED_CURVE()
B_SPLINE_CURVE(2,(#24472,#24473,#24474),.UNSPECIFIED.,.F.,.F.)
B_SPLINE_CURVE_WITH_KNOTS((3,3),(0.0660091927116034,0.110314456526687),
 .UNSPECIFIED.)
CURVE()
GEOMETRIC_REPRESENTATION_ITEM()
RATIONAL_B_SPLINE_CURVE((1.00002048940631,1.00001712140889,1.00000000159591))
REPRESENTATION_ITEM('')
);
#1090=(
BOUNDED_CURVE()
B_SPLINE_CURVE(2,(#24495,#24496,#24497),.UNSPECIFIED.,.F.,.F.)
B_SPLINE_CURVE_WITH_KNOTS((3,3),(7.86559625577519E-6,0.061239637372806),
 .UNSPECIFIED.)
CURVE()
GEOMETRIC_REPRESENTATION_ITEM()
RATIONAL_B_SPLINE_CURVE((1.00001915745326,1.07458139657232,1.05821963517917))
REPRESENTATION_ITEM('')
);
#1091=(
BOUNDED_CURVE()
B_SPLINE_CURVE(2,(#24505,#24506,#24507),.UNSPECIFIED.,.F.,.F.)
B_SPLINE_CURVE_WITH_KNOTS((3,3),(2.06502884983613E-6,0.0443073288439088),
 .UNSPECIFIED.)
CURVE()
GEOMETRIC_REPRESENTATION_ITEM()
RATIONAL_B_SPLINE_CURVE((1.00000000159591,1.00001712140953,1.00002048940709))
REPRESENTATION_ITEM('')
);
#1092=(
BOUNDED_CURVE()
B_SPLINE_CURVE(2,(#24509,#24510,#24511),.UNSPECIFIED.,.F.,.F.)
B_SPLINE_CURVE_WITH_KNOTS((3,3),(0.0392023395450886,0.10043411132165),
 .UNSPECIFIED.)
CURVE()
GEOMETRIC_REPRESENTATION_ITEM()
RATIONAL_B_SPLINE_CURVE((1.05821963517901,1.07458139657211,1.00001915745323))
REPRESENTATION_ITEM('')
);
#1093=(
BOUNDED_CURVE()
B_SPLINE_CURVE(2,(#24517,#24518,#24519),.UNSPECIFIED.,.F.,.F.)
B_SPLINE_CURVE_WITH_KNOTS((3,3),(0.0660091927116451,0.110314456526683),
 .UNSPECIFIED.)
CURVE()
GEOMETRIC_REPRESENTATION_ITEM()
RATIONAL_B_SPLINE_CURVE((1.00002048940605,1.00001712140867,1.00000000159591))
REPRESENTATION_ITEM('')
);
#1094=(
BOUNDED_CURVE()
B_SPLINE_CURVE(2,(#24540,#24541,#24542),.UNSPECIFIED.,.F.,.F.)
B_SPLINE_CURVE_WITH_KNOTS((3,3),(7.86559624689154E-6,0.061239637372801),
 .UNSPECIFIED.)
CURVE()
GEOMETRIC_REPRESENTATION_ITEM()
RATIONAL_B_SPLINE_CURVE((1.00001915745324,1.07458139657241,1.05821963517924))
REPRESENTATION_ITEM('')
);
#1095=(
BOUNDED_CURVE()
B_SPLINE_CURVE(2,(#24550,#24551,#24552),.UNSPECIFIED.,.F.,.F.)
B_SPLINE_CURVE_WITH_KNOTS((3,3),(2.0650288490547E-6,0.0443073288439657),
 .UNSPECIFIED.)
CURVE()
GEOMETRIC_REPRESENTATION_ITEM()
RATIONAL_B_SPLINE_CURVE((1.00000000159591,1.00001712141033,1.00002048940803))
REPRESENTATION_ITEM('')
);
#1096=(
BOUNDED_CURVE()
B_SPLINE_CURVE(2,(#24554,#24555,#24556),.UNSPECIFIED.,.F.,.F.)
B_SPLINE_CURVE_WITH_KNOTS((3,3),(0.0392023395450856,0.100434111321651),
 .UNSPECIFIED.)
CURVE()
GEOMETRIC_REPRESENTATION_ITEM()
RATIONAL_B_SPLINE_CURVE((1.0582196351791,1.07458139657223,1.0000191574532))
REPRESENTATION_ITEM('')
);
#1097=(
BOUNDED_CURVE()
B_SPLINE_CURVE(2,(#24562,#24563,#24564),.UNSPECIFIED.,.F.,.F.)
B_SPLINE_CURVE_WITH_KNOTS((3,3),(0.0660091927115862,0.110314456526683),
 .UNSPECIFIED.)
CURVE()
GEOMETRIC_REPRESENTATION_ITEM()
RATIONAL_B_SPLINE_CURVE((1.00002048940501,1.00001712140779,1.00000000159591))
REPRESENTATION_ITEM('')
);
#1098=(
BOUNDED_CURVE()
B_SPLINE_CURVE(2,(#24585,#24586,#24587),.UNSPECIFIED.,.F.,.F.)
B_SPLINE_CURVE_WITH_KNOTS((3,3),(7.86559623861992E-6,0.0612396373727923),
 .UNSPECIFIED.)
CURVE()
GEOMETRIC_REPRESENTATION_ITEM()
RATIONAL_B_SPLINE_CURVE((1.00001915745322,1.07458139657228,1.05821963517915))
REPRESENTATION_ITEM('')
);
#1099=(
BOUNDED_CURVE()
B_SPLINE_CURVE(2,(#24595,#24596,#24597),.UNSPECIFIED.,.F.,.F.)
B_SPLINE_CURVE_WITH_KNOTS((3,3),(2.06502884791252E-6,0.0443073288439309),
 .UNSPECIFIED.)
CURVE()
GEOMETRIC_REPRESENTATION_ITEM()
RATIONAL_B_SPLINE_CURVE((1.00000000159591,1.00001712140764,1.00002048940482))
REPRESENTATION_ITEM('')
);
#1100=(
BOUNDED_CURVE()
B_SPLINE_CURVE(2,(#24599,#24600,#24601),.UNSPECIFIED.,.F.,.F.)
B_SPLINE_CURVE_WITH_KNOTS((3,3),(0.0392023395450768,0.100434111321634),
 .UNSPECIFIED.)
CURVE()
GEOMETRIC_REPRESENTATION_ITEM()
RATIONAL_B_SPLINE_CURVE((1.05821963517911,1.07458139657224,1.00001915745319))
REPRESENTATION_ITEM('')
);
#1101=(
BOUNDED_CURVE()
B_SPLINE_CURVE(2,(#24607,#24608,#24609),.UNSPECIFIED.,.F.,.F.)
B_SPLINE_CURVE_WITH_KNOTS((3,3),(0.0660091927116233,0.11031445652668),
 .UNSPECIFIED.)
CURVE()
GEOMETRIC_REPRESENTATION_ITEM()
RATIONAL_B_SPLINE_CURVE((1.00002048941031,1.00001712141222,1.00000000159591))
REPRESENTATION_ITEM('')
);
#1102=(
BOUNDED_CURVE()
B_SPLINE_CURVE(2,(#24630,#24631,#24632),.UNSPECIFIED.,.F.,.F.)
B_SPLINE_CURVE_WITH_KNOTS((3,3),(7.8735648790627E-6,0.0613120861126728),
 .UNSPECIFIED.)
CURVE()
GEOMETRIC_REPRESENTATION_ITEM()
RATIONAL_B_SPLINE_CURVE((1.00001920106114,1.0747638688358,1.05857900734984))
REPRESENTATION_ITEM('')
);
#1103=(
BOUNDED_CURVE()
B_SPLINE_CURVE(2,(#24637,#24638,#24639),.UNSPECIFIED.,.F.,.F.)
B_SPLINE_CURVE_WITH_KNOTS((3,3),(0.0392028994779419,0.100212511691547),
 .UNSPECIFIED.)
CURVE()
GEOMETRIC_REPRESENTATION_ITEM()
RATIONAL_B_SPLINE_CURVE((1.06060654550647,1.0784249750017,1.00491903156505))
REPRESENTATION_ITEM('')
);
#1104=(
BOUNDED_CURVE()
B_SPLINE_CURVE(2,(#24658,#24659,#24660),.UNSPECIFIED.,.F.,.F.)
B_SPLINE_CURVE_WITH_KNOTS((3,3),(2.36858664140126,2.48027053188039),
 .UNSPECIFIED.)
CURVE()
GEOMETRIC_REPRESENTATION_ITEM()
RATIONAL_B_SPLINE_CURVE((1.00156925623442,1.0009208220165,1.00020774873445))
REPRESENTATION_ITEM('')
);
#1105=(
BOUNDED_CURVE()
B_SPLINE_CURVE(2,(#24994,#24995,#24996),.UNSPECIFIED.,.F.,.F.)
B_SPLINE_CURVE_WITH_KNOTS((3,3),(0.066268784781115,0.11057326983442),
 .UNSPECIFIED.)
CURVE()
GEOMETRIC_REPRESENTATION_ITEM()
RATIONAL_B_SPLINE_CURVE((1.00002057034838,1.00001716188265,1.00000000159968))
REPRESENTATION_ITEM('')
);
#1106=(
BOUNDED_CURVE()
B_SPLINE_CURVE(2,(#25003,#25004,#25005),.UNSPECIFIED.,.F.,.F.)
B_SPLINE_CURVE_WITH_KNOTS((3,3),(7.86559624521441E-6,0.0612396373727986),
 .UNSPECIFIED.)
CURVE()
GEOMETRIC_REPRESENTATION_ITEM()
RATIONAL_B_SPLINE_CURVE((1.00001915745323,1.07458139657223,1.05821963517911))
REPRESENTATION_ITEM('')
);
#1107=(
BOUNDED_CURVE()
B_SPLINE_CURVE(2,(#25010,#25011,#25012),.UNSPECIFIED.,.F.,.F.)
B_SPLINE_CURVE_WITH_KNOTS((3,3),(0.039202339545088,0.100434111321661),
 .UNSPECIFIED.)
CURVE()
GEOMETRIC_REPRESENTATION_ITEM()
RATIONAL_B_SPLINE_CURVE((1.05821963517928,1.07458139657247,1.00001915745322))
REPRESENTATION_ITEM('')
);
#1108=(
BOUNDED_CURVE()
B_SPLINE_CURVE(2,(#25030,#25031,#25032),.UNSPECIFIED.,.F.,.F.)
B_SPLINE_CURVE_WITH_KNOTS((3,3),(2.06502885058066E-6,0.0443073288438408),
 .UNSPECIFIED.)
CURVE()
GEOMETRIC_REPRESENTATION_ITEM()
RATIONAL_B_SPLINE_CURVE((1.00000000159591,1.00001712141098,1.00002048940882))
REPRESENTATION_ITEM('')
);
#1109=(
BOUNDED_CURVE()
B_SPLINE_CURVE(2,(#25036,#25037,#25038),.UNSPECIFIED.,.F.,.F.)
B_SPLINE_CURVE_WITH_KNOTS((3,3),(0.066009192711637,0.110314456526716),
 .UNSPECIFIED.)
CURVE()
GEOMETRIC_REPRESENTATION_ITEM()
RATIONAL_B_SPLINE_CURVE((1.00002048940915,1.00001712141126,1.00000000159591))
REPRESENTATION_ITEM('')
);
#1110=(
BOUNDED_CURVE()
B_SPLINE_CURVE(2,(#25045,#25046,#25047),.UNSPECIFIED.,.F.,.F.)
B_SPLINE_CURVE_WITH_KNOTS((3,3),(7.86559623619297E-6,0.06123963737278),
 .UNSPECIFIED.)
CURVE()
GEOMETRIC_REPRESENTATION_ITEM()
RATIONAL_B_SPLINE_CURVE((1.00001915745321,1.0745813965721,1.058219635179))
REPRESENTATION_ITEM('')
);
#1111=(
BOUNDED_CURVE()
B_SPLINE_CURVE(2,(#25052,#25053,#25054),.UNSPECIFIED.,.F.,.F.)
B_SPLINE_CURVE_WITH_KNOTS((3,3),(0.039202339545078,0.100434111321636),
 .UNSPECIFIED.)
CURVE()
GEOMETRIC_REPRESENTATION_ITEM()
RATIONAL_B_SPLINE_CURVE((1.05821963517909,1.07458139657222,1.0000191574532))
REPRESENTATION_ITEM('')
);
#1112=(
BOUNDED_CURVE()
B_SPLINE_CURVE(2,(#25072,#25073,#25074),.UNSPECIFIED.,.F.,.F.)
B_SPLINE_CURVE_WITH_KNOTS((3,3),(2.06502885091957E-6,0.0443073288439418),
 .UNSPECIFIED.)
CURVE()
GEOMETRIC_REPRESENTATION_ITEM()
RATIONAL_B_SPLINE_CURVE((1.00000000159591,1.00001712141366,1.00002048941202))
REPRESENTATION_ITEM('')
);
#1113=(
BOUNDED_CURVE()
B_SPLINE_CURVE(2,(#25078,#25079,#25080),.UNSPECIFIED.,.F.,.F.)
B_SPLINE_CURVE_WITH_KNOTS((3,3),(0.066009192711676,0.110314456526716),
 .UNSPECIFIED.)
CURVE()
GEOMETRIC_REPRESENTATION_ITEM()
RATIONAL_B_SPLINE_CURVE((1.00002048941196,1.0000171214136,1.00000000159591))
REPRESENTATION_ITEM('')
);
#1114=(
BOUNDED_CURVE()
B_SPLINE_CURVE(2,(#25087,#25088,#25089),.UNSPECIFIED.,.F.,.F.)
B_SPLINE_CURVE_WITH_KNOTS((3,3),(7.86559624634883E-6,0.0612396373727915),
 .UNSPECIFIED.)
CURVE()
GEOMETRIC_REPRESENTATION_ITEM()
RATIONAL_B_SPLINE_CURVE((1.00001915745324,1.07458139657221,1.05821963517909))
REPRESENTATION_ITEM('')
);
#1115=(
BOUNDED_CURVE()
B_SPLINE_CURVE(2,(#25094,#25095,#25096),.UNSPECIFIED.,.F.,.F.)
B_SPLINE_CURVE_WITH_KNOTS((3,3),(0.0392023395450874,0.100434111321651),
 .UNSPECIFIED.)
CURVE()
GEOMETRIC_REPRESENTATION_ITEM()
RATIONAL_B_SPLINE_CURVE((1.05821963517914,1.07458139657228,1.00001915745321))
REPRESENTATION_ITEM('')
);
#1116=(
BOUNDED_CURVE()
B_SPLINE_CURVE(2,(#25111,#25112,#25113),.UNSPECIFIED.,.F.,.F.)
B_SPLINE_CURVE_WITH_KNOTS((3,3),(0.0142112171257214,0.110567648737575),
 .UNSPECIFIED.)
CURVE()
GEOMETRIC_REPRESENTATION_ITEM()
RATIONAL_B_SPLINE_CURVE((1.00000961767768,1.0000374265062,1.0000001907434))
REPRESENTATION_ITEM('')
);
#1117=(
BOUNDED_CURVE()
B_SPLINE_CURVE(2,(#25124,#25125,#25126),.UNSPECIFIED.,.F.,.F.)
B_SPLINE_CURVE_WITH_KNOTS((3,3),(0.000246247416174898,0.0445514940289623),
 .UNSPECIFIED.)
CURVE()
GEOMETRIC_REPRESENTATION_ITEM()
RATIONAL_B_SPLINE_CURVE((1.00000019074344,1.00001731196687,1.00002068137031))
REPRESENTATION_ITEM('')
);
#1118=(
BOUNDED_CURVE()
B_SPLINE_CURVE(2,(#25136,#25137,#25138),.UNSPECIFIED.,.F.,.F.)
B_SPLINE_CURVE_WITH_KNOTS((3,3),(0.000246247416180695,0.0966026790274006),
 .UNSPECIFIED.)
CURVE()
GEOMETRIC_REPRESENTATION_ITEM()
RATIONAL_B_SPLINE_CURVE((1.00000019074341,1.00003742650782,1.00000961767809))
REPRESENTATION_ITEM('')
);
#1119=(
BOUNDED_CURVE()
B_SPLINE_CURVE(2,(#25144,#25145,#25146),.UNSPECIFIED.,.F.,.F.)
B_SPLINE_CURVE_WITH_KNOTS((3,3),(0.0662624021247591,0.110567648737568),
 .UNSPECIFIED.)
CURVE()
GEOMETRIC_REPRESENTATION_ITEM()
RATIONAL_B_SPLINE_CURVE((1.00002068136531,1.00001731196269,1.0000001907434))
REPRESENTATION_ITEM('')
);
#1120=(
BOUNDED_CURVE()
B_SPLINE_CURVE(2,(#25164,#25165,#25166),.UNSPECIFIED.,.F.,.F.)
B_SPLINE_CURVE_WITH_KNOTS((3,3),(7.86559624155621E-6,0.0612396373727861),
 .UNSPECIFIED.)
CURVE()
GEOMETRIC_REPRESENTATION_ITEM()
RATIONAL_B_SPLINE_CURVE((1.00001915745323,1.07458139657213,1.05821963517903))
REPRESENTATION_ITEM('')
);
#1121=(
BOUNDED_CURVE()
B_SPLINE_CURVE(2,(#25174,#25175,#25176),.UNSPECIFIED.,.F.,.F.)
B_SPLINE_CURVE_WITH_KNOTS((3,3),(2.06502885047952E-6,0.0443073288439063),
 .UNSPECIFIED.)
CURVE()
GEOMETRIC_REPRESENTATION_ITEM()
RATIONAL_B_SPLINE_CURVE((1.00000000159591,1.00001712141005,1.00002048940771))
REPRESENTATION_ITEM('')
);
#1122=(
BOUNDED_CURVE()
B_SPLINE_CURVE(2,(#25178,#25179,#25180),.UNSPECIFIED.,.F.,.F.)
B_SPLINE_CURVE_WITH_KNOTS((3,3),(0.039202339545091,0.100434111321655),
 .UNSPECIFIED.)
CURVE()
GEOMETRIC_REPRESENTATION_ITEM()
RATIONAL_B_SPLINE_CURVE((1.05821963517907,1.07458139657219,1.0000191574532))
REPRESENTATION_ITEM('')
);
#1123=(
BOUNDED_CURVE()
B_SPLINE_CURVE(2,(#25186,#25187,#25188),.UNSPECIFIED.,.F.,.F.)
B_SPLINE_CURVE_WITH_KNOTS((3,3),(0.0660091927117379,0.110314456526716),
 .UNSPECIFIED.)
CURVE()
GEOMETRIC_REPRESENTATION_ITEM()
RATIONAL_B_SPLINE_CURVE((1.00002048940992,1.0000171214119,1.00000000159591))
REPRESENTATION_ITEM('')
);
#1124=(
BOUNDED_CURVE()
B_SPLINE_CURVE(2,(#25206,#25207,#25208),.UNSPECIFIED.,.F.,.F.)
B_SPLINE_CURVE_WITH_KNOTS((3,3),(7.86559624404147E-6,0.0612396373727875),
 .UNSPECIFIED.)
CURVE()
GEOMETRIC_REPRESENTATION_ITEM()
RATIONAL_B_SPLINE_CURVE((1.00001915745323,1.07458139657229,1.05821963517915))
REPRESENTATION_ITEM('')
);
#1125=(
BOUNDED_CURVE()
B_SPLINE_CURVE(2,(#25216,#25217,#25218),.UNSPECIFIED.,.F.,.F.)
B_SPLINE_CURVE_WITH_KNOTS((3,3),(2.06502885034354E-6,0.0443073288439307),
 .UNSPECIFIED.)
CURVE()
GEOMETRIC_REPRESENTATION_ITEM()
RATIONAL_B_SPLINE_CURVE((1.00000000159591,1.00001712141048,1.00002048940822))
REPRESENTATION_ITEM('')
);
#1126=(
BOUNDED_CURVE()
B_SPLINE_CURVE(2,(#25220,#25221,#25222),.UNSPECIFIED.,.F.,.F.)
B_SPLINE_CURVE_WITH_KNOTS((3,3),(0.039202339545077,0.100434111321635),
 .UNSPECIFIED.)
CURVE()
GEOMETRIC_REPRESENTATION_ITEM()
RATIONAL_B_SPLINE_CURVE((1.05821963517913,1.07458139657227,1.00001915745318))
REPRESENTATION_ITEM('')
);
#1127=(
BOUNDED_CURVE()
B_SPLINE_CURVE(2,(#25228,#25229,#25230),.UNSPECIFIED.,.F.,.F.)
B_SPLINE_CURVE_WITH_KNOTS((3,3),(0.0660091927115155,0.110314456526713),
 .UNSPECIFIED.)
CURVE()
GEOMETRIC_REPRESENTATION_ITEM()
RATIONAL_B_SPLINE_CURVE((1.00002048939951,1.0000171214032,1.00000000159591))
REPRESENTATION_ITEM('')
);
#1128=(
BOUNDED_CURVE()
B_SPLINE_CURVE(2,(#25248,#25249,#25250),.UNSPECIFIED.,.F.,.F.)
B_SPLINE_CURVE_WITH_KNOTS((3,3),(7.8655962495386E-6,0.0612396373727939),
 .UNSPECIFIED.)
CURVE()
GEOMETRIC_REPRESENTATION_ITEM()
RATIONAL_B_SPLINE_CURVE((1.00001915745324,1.07458139657231,1.05821963517916))
REPRESENTATION_ITEM('')
);
#1129=(
BOUNDED_CURVE()
B_SPLINE_CURVE(2,(#25258,#25259,#25260),.UNSPECIFIED.,.F.,.F.)
B_SPLINE_CURVE_WITH_KNOTS((3,3),(2.06502884777574E-6,0.0443073288439337),
 .UNSPECIFIED.)
CURVE()
GEOMETRIC_REPRESENTATION_ITEM()
RATIONAL_B_SPLINE_CURVE((1.00000000159591,1.00001712140949,1.00002048940703))
REPRESENTATION_ITEM('')
);
#1130=(
BOUNDED_CURVE()
B_SPLINE_CURVE(2,(#25262,#25263,#25264),.UNSPECIFIED.,.F.,.F.)
B_SPLINE_CURVE_WITH_KNOTS((3,3),(0.0392023395450778,0.100434111321633),
 .UNSPECIFIED.)
CURVE()
GEOMETRIC_REPRESENTATION_ITEM()
RATIONAL_B_SPLINE_CURVE((1.05821963517902,1.07458139657213,1.00001915745319))
REPRESENTATION_ITEM('')
);
#1131=(
BOUNDED_CURVE()
B_SPLINE_CURVE(2,(#25270,#25271,#25272),.UNSPECIFIED.,.F.,.F.)
B_SPLINE_CURVE_WITH_KNOTS((3,3),(0.0660091927116281,0.110314456526714),
 .UNSPECIFIED.)
CURVE()
GEOMETRIC_REPRESENTATION_ITEM()
RATIONAL_B_SPLINE_CURVE((1.00002048941071,1.00001712141256,1.00000000159591))
REPRESENTATION_ITEM('')
);
#1132=(
BOUNDED_CURVE()
B_SPLINE_CURVE(2,(#25290,#25291,#25292),.UNSPECIFIED.,.F.,.F.)
B_SPLINE_CURVE_WITH_KNOTS((3,3),(7.86559623181466E-6,0.061239637372782),
 .UNSPECIFIED.)
CURVE()
GEOMETRIC_REPRESENTATION_ITEM()
RATIONAL_B_SPLINE_CURVE((1.0000191574532,1.07458139657242,1.05821963517925))
REPRESENTATION_ITEM('')
);
#1133=(
BOUNDED_CURVE()
B_SPLINE_CURVE(2,(#25300,#25301,#25302),.UNSPECIFIED.,.F.,.F.)
B_SPLINE_CURVE_WITH_KNOTS((3,3),(2.06502885033157E-6,0.0443073288437829),
 .UNSPECIFIED.)
CURVE()
GEOMETRIC_REPRESENTATION_ITEM()
RATIONAL_B_SPLINE_CURVE((1.00000000159591,1.00001712141826,1.00002048941753))
REPRESENTATION_ITEM('')
);
#1134=(
BOUNDED_CURVE()
B_SPLINE_CURVE(2,(#25304,#25305,#25306),.UNSPECIFIED.,.F.,.F.)
B_SPLINE_CURVE_WITH_KNOTS((3,3),(0.0392023395450864,0.100434111321655),
 .UNSPECIFIED.)
CURVE()
GEOMETRIC_REPRESENTATION_ITEM()
RATIONAL_B_SPLINE_CURVE((1.05821963517922,1.07458139657238,1.00001915745319))
REPRESENTATION_ITEM('')
);
#1135=(
BOUNDED_CURVE()
B_SPLINE_CURVE(2,(#25312,#25313,#25314),.UNSPECIFIED.,.F.,.F.)
B_SPLINE_CURVE_WITH_KNOTS((3,3),(0.06600919271163,0.110314456526716),
 .UNSPECIFIED.)
CURVE()
GEOMETRIC_REPRESENTATION_ITEM()
RATIONAL_B_SPLINE_CURVE((1.00002048941218,1.00001712141379,1.00000000159591))
REPRESENTATION_ITEM('')
);
#1136=(
BOUNDED_CURVE()
B_SPLINE_CURVE(2,(#25332,#25333,#25334),.UNSPECIFIED.,.F.,.F.)
B_SPLINE_CURVE_WITH_KNOTS((3,3),(7.86559623262009E-6,0.0612396373727778),
 .UNSPECIFIED.)
CURVE()
GEOMETRIC_REPRESENTATION_ITEM()
RATIONAL_B_SPLINE_CURVE((1.0000191574532,1.07458139657217,1.05821963517906))
REPRESENTATION_ITEM('')
);
#1137=(
BOUNDED_CURVE()
B_SPLINE_CURVE(2,(#25342,#25343,#25344),.UNSPECIFIED.,.F.,.F.)
B_SPLINE_CURVE_WITH_KNOTS((3,3),(2.06499351855609E-6,0.0443065724917911),
 .UNSPECIFIED.)
CURVE()
GEOMETRIC_REPRESENTATION_ITEM()
RATIONAL_B_SPLINE_CURVE((1.00000000159957,1.00001716071458,1.00002056801363))
REPRESENTATION_ITEM('')
);
#1138=(
BOUNDED_CURVE()
B_SPLINE_CURVE(2,(#25346,#25347,#25348),.UNSPECIFIED.,.F.,.F.)
B_SPLINE_CURVE_WITH_KNOTS((3,3),(0.0392023395450884,0.100434111321656),
 .UNSPECIFIED.)
CURVE()
GEOMETRIC_REPRESENTATION_ITEM()
RATIONAL_B_SPLINE_CURVE((1.05821963517918,1.07458139657233,1.00001915745319))
REPRESENTATION_ITEM('')
);
#1139=(
BOUNDED_CURVE()
B_SPLINE_CURVE(2,(#25354,#25355,#25356),.UNSPECIFIED.,.F.,.F.)
B_SPLINE_CURVE_WITH_KNOTS((3,3),(0.0142112171256352,0.110567648737535),
 .UNSPECIFIED.)
CURVE()
GEOMETRIC_REPRESENTATION_ITEM()
RATIONAL_B_SPLINE_CURVE((1.00000961767813,1.00003742650796,1.00000019074341))
REPRESENTATION_ITEM('')
);
#1140=(
BOUNDED_CURVE()
B_SPLINE_CURVE(2,(#25426,#25427,#25428),.UNSPECIFIED.,.F.,.F.)
B_SPLINE_CURVE_WITH_KNOTS((3,3),(0.0662606539244614,0.110565163369973),
 .UNSPECIFIED.)
CURVE()
GEOMETRIC_REPRESENTATION_ITEM()
RATIONAL_B_SPLINE_CURVE((1.00002056781072,1.00001716061294,1.00000000159956))
REPRESENTATION_ITEM('')
);
#1141=(
BOUNDED_CURVE()
B_SPLINE_CURVE(2,(#25435,#25436,#25437),.UNSPECIFIED.,.F.,.F.)
B_SPLINE_CURVE_WITH_KNOTS((3,3),(7.86559624220057E-6,0.0612396373727874),
 .UNSPECIFIED.)
CURVE()
GEOMETRIC_REPRESENTATION_ITEM()
RATIONAL_B_SPLINE_CURVE((1.00001915745323,1.07458139657226,1.05821963517912))
REPRESENTATION_ITEM('')
);
#1142=(
BOUNDED_CURVE()
B_SPLINE_CURVE(2,(#25442,#25443,#25444),.UNSPECIFIED.,.F.,.F.)
B_SPLINE_CURVE_WITH_KNOTS((3,3),(0.0392023395450873,0.100434111321653),
 .UNSPECIFIED.)
CURVE()
GEOMETRIC_REPRESENTATION_ITEM()
RATIONAL_B_SPLINE_CURVE((1.05821963517917,1.07458139657232,1.00001915745321))
REPRESENTATION_ITEM('')
);
#1143=(
BOUNDED_CURVE()
B_SPLINE_CURVE(2,(#25462,#25463,#25464),.UNSPECIFIED.,.F.,.F.)
B_SPLINE_CURVE_WITH_KNOTS((3,3),(2.06502885188068E-6,0.0443073288438163),
 .UNSPECIFIED.)
CURVE()
GEOMETRIC_REPRESENTATION_ITEM()
RATIONAL_B_SPLINE_CURVE((1.00000000159591,1.00001712140878,1.00002048940618))
REPRESENTATION_ITEM('')
);
#1144=(
BOUNDED_CURVE()
B_SPLINE_CURVE(2,(#25469,#25470,#25471),.UNSPECIFIED.,.F.,.F.)
B_SPLINE_CURVE_WITH_KNOTS((3,3),(0.0660091927116148,0.110314456526714),
 .UNSPECIFIED.)
CURVE()
GEOMETRIC_REPRESENTATION_ITEM()
RATIONAL_B_SPLINE_CURVE((1.00002048940315,1.00001712140625,1.00000000159591))
REPRESENTATION_ITEM('')
);
#1145=(
BOUNDED_CURVE()
B_SPLINE_CURVE(2,(#25483,#25484,#25485),.UNSPECIFIED.,.F.,.F.)
B_SPLINE_CURVE_WITH_KNOTS((3,3),(7.86559624218418E-6,0.0612396373727888),
 .UNSPECIFIED.)
CURVE()
GEOMETRIC_REPRESENTATION_ITEM()
RATIONAL_B_SPLINE_CURVE((1.00001915745323,1.07458139657228,1.05821963517914))
REPRESENTATION_ITEM('')
);
#1146=(
BOUNDED_CURVE()
B_SPLINE_CURVE(2,(#25490,#25491,#25492),.UNSPECIFIED.,.F.,.F.)
B_SPLINE_CURVE_WITH_KNOTS((3,3),(0.039202339545094,0.100434111321663),
 .UNSPECIFIED.)
CURVE()
GEOMETRIC_REPRESENTATION_ITEM()
RATIONAL_B_SPLINE_CURVE((1.05821963517907,1.07458139657219,1.00001915745321))
REPRESENTATION_ITEM('')
);
#1147=(
BOUNDED_CURVE()
B_SPLINE_CURVE(2,(#25506,#25507,#25508),.UNSPECIFIED.,.F.,.F.)
B_SPLINE_CURVE_WITH_KNOTS((3,3),(2.06502885290881E-6,0.0443073288438236),
 .UNSPECIFIED.)
CURVE()
GEOMETRIC_REPRESENTATION_ITEM()
RATIONAL_B_SPLINE_CURVE((1.00000000159591,1.0000171214084,1.00002048940573))
REPRESENTATION_ITEM('')
);
#1148=(
BOUNDED_CURVE()
B_SPLINE_CURVE(2,(#25512,#25513,#25514),.UNSPECIFIED.,.F.,.F.)
B_SPLINE_CURVE_WITH_KNOTS((3,3),(0.0660091927116525,0.110314456526715),
 .UNSPECIFIED.)
CURVE()
GEOMETRIC_REPRESENTATION_ITEM()
RATIONAL_B_SPLINE_CURVE((1.00002048941054,1.00001712141242,1.00000000159591))
REPRESENTATION_ITEM('')
);
#1149=(
BOUNDED_CURVE()
B_SPLINE_CURVE(2,(#25521,#25522,#25523),.UNSPECIFIED.,.F.,.F.)
B_SPLINE_CURVE_WITH_KNOTS((3,3),(7.86559624776651E-6,0.0612396373727933),
 .UNSPECIFIED.)
CURVE()
GEOMETRIC_REPRESENTATION_ITEM()
RATIONAL_B_SPLINE_CURVE((1.00001915745324,1.07458139657231,1.05821963517916))
REPRESENTATION_ITEM('')
);
#1150=(
BOUNDED_CURVE()
B_SPLINE_CURVE(2,(#25528,#25529,#25530),.UNSPECIFIED.,.F.,.F.)
B_SPLINE_CURVE_WITH_KNOTS((3,3),(0.0392023395450758,0.100434111321633),
 .UNSPECIFIED.)
CURVE()
GEOMETRIC_REPRESENTATION_ITEM()
RATIONAL_B_SPLINE_CURVE((1.05821963517916,1.07458139657231,1.00001915745321))
REPRESENTATION_ITEM('')
);
#1151=(
BOUNDED_CURVE()
B_SPLINE_CURVE(2,(#25548,#25549,#25550),.UNSPECIFIED.,.F.,.F.)
B_SPLINE_CURVE_WITH_KNOTS((3,3),(2.06502885179237E-6,0.0443073288439585),
 .UNSPECIFIED.)
CURVE()
GEOMETRIC_REPRESENTATION_ITEM()
RATIONAL_B_SPLINE_CURVE((1.00000000159591,1.00001712140818,1.00002048940547))
REPRESENTATION_ITEM('')
);
#1152=(
BOUNDED_CURVE()
B_SPLINE_CURVE(2,(#25554,#25555,#25556),.UNSPECIFIED.,.F.,.F.)
B_SPLINE_CURVE_WITH_KNOTS((3,3),(0.0660091927116068,0.110314456526714),
 .UNSPECIFIED.)
CURVE()
GEOMETRIC_REPRESENTATION_ITEM()
RATIONAL_B_SPLINE_CURVE((1.00002048940856,1.00001712141077,1.00000000159591))
REPRESENTATION_ITEM('')
);
#1153=(
BOUNDED_CURVE()
B_SPLINE_CURVE(2,(#25563,#25564,#25565),.UNSPECIFIED.,.F.,.F.)
B_SPLINE_CURVE_WITH_KNOTS((3,3),(7.86559623936065E-6,0.0612396373727857),
 .UNSPECIFIED.)
CURVE()
GEOMETRIC_REPRESENTATION_ITEM()
RATIONAL_B_SPLINE_CURVE((1.00001915745322,1.07458139657226,1.05821963517912))
REPRESENTATION_ITEM('')
);
#1154=(
BOUNDED_CURVE()
B_SPLINE_CURVE(2,(#25570,#25571,#25572),.UNSPECIFIED.,.F.,.F.)
B_SPLINE_CURVE_WITH_KNOTS((3,3),(0.0392023395450771,0.100434111321633),
 .UNSPECIFIED.)
CURVE()
GEOMETRIC_REPRESENTATION_ITEM()
RATIONAL_B_SPLINE_CURVE((1.05821963517909,1.07458139657222,1.00001915745321))
REPRESENTATION_ITEM('')
);
#1155=(
BOUNDED_CURVE()
B_SPLINE_CURVE(2,(#25588,#25589,#25590),.UNSPECIFIED.,.F.,.F.)
B_SPLINE_CURVE_WITH_KNOTS((3,3),(0.0142112171255719,0.110567648737547),
 .UNSPECIFIED.)
CURVE()
GEOMETRIC_REPRESENTATION_ITEM()
RATIONAL_B_SPLINE_CURVE((1.00000961768055,1.0000374265174,1.00000019074346))
REPRESENTATION_ITEM('')
);
#1156=(
BOUNDED_CURVE()
B_SPLINE_CURVE(2,(#25607,#25608,#25609),.UNSPECIFIED.,.F.,.F.)
B_SPLINE_CURVE_WITH_KNOTS((3,3),(0.000246247416175262,0.0445514940288951),
 .UNSPECIFIED.)
CURVE()
GEOMETRIC_REPRESENTATION_ITEM()
RATIONAL_B_SPLINE_CURVE((1.00000019074347,1.00001731196895,1.00002068137279))
REPRESENTATION_ITEM('')
);
#1157=(
BOUNDED_CURVE()
B_SPLINE_CURVE(2,(#25619,#25620,#25621),.UNSPECIFIED.,.F.,.F.)
B_SPLINE_CURVE_WITH_KNOTS((3,3),(0.00024624741617372,0.0966026790275413),
 .UNSPECIFIED.)
CURVE()
GEOMETRIC_REPRESENTATION_ITEM()
RATIONAL_B_SPLINE_CURVE((1.00000019074349,1.00003742652381,1.0000096176822))
REPRESENTATION_ITEM('')
);
#1158=(
BOUNDED_CURVE()
B_SPLINE_CURVE(2,(#25627,#25628,#25629),.UNSPECIFIED.,.F.,.F.)
B_SPLINE_CURVE_WITH_KNOTS((3,3),(0.0662624021246591,0.110567648737537),
 .UNSPECIFIED.)
CURVE()
GEOMETRIC_REPRESENTATION_ITEM()
RATIONAL_B_SPLINE_CURVE((1.00002068136771,1.0000173119647,1.00000019074342))
REPRESENTATION_ITEM('')
);
#1159=(
BOUNDED_CURVE()
B_SPLINE_CURVE(2,(#25647,#25648,#25649),.UNSPECIFIED.,.F.,.F.)
B_SPLINE_CURVE_WITH_KNOTS((3,3),(7.86559625117043E-6,0.0612396373728031),
 .UNSPECIFIED.)
CURVE()
GEOMETRIC_REPRESENTATION_ITEM()
RATIONAL_B_SPLINE_CURVE((1.00001915745325,1.07458139657221,1.05821963517909))
REPRESENTATION_ITEM('')
);
#1160=(
BOUNDED_CURVE()
B_SPLINE_CURVE(2,(#25657,#25658,#25659),.UNSPECIFIED.,.F.,.F.)
B_SPLINE_CURVE_WITH_KNOTS((3,3),(2.06502885156182E-6,0.0443073288437527),
 .UNSPECIFIED.)
CURVE()
GEOMETRIC_REPRESENTATION_ITEM()
RATIONAL_B_SPLINE_CURVE((1.00000000159591,1.00001712141345,1.00002048941177))
REPRESENTATION_ITEM('')
);
#1161=(
BOUNDED_CURVE()
B_SPLINE_CURVE(2,(#25661,#25662,#25663),.UNSPECIFIED.,.F.,.F.)
B_SPLINE_CURVE_WITH_KNOTS((3,3),(0.0392023395450928,0.100434111321662),
 .UNSPECIFIED.)
CURVE()
GEOMETRIC_REPRESENTATION_ITEM()
RATIONAL_B_SPLINE_CURVE((1.05821963517921,1.07458139657238,1.00001915745323))
REPRESENTATION_ITEM('')
);
#1162=(
BOUNDED_CURVE()
B_SPLINE_CURVE(2,(#25669,#25670,#25671),.UNSPECIFIED.,.F.,.F.)
B_SPLINE_CURVE_WITH_KNOTS((3,3),(0.0660091927115642,0.110314456526669),
 .UNSPECIFIED.)
CURVE()
GEOMETRIC_REPRESENTATION_ITEM()
RATIONAL_B_SPLINE_CURVE((1.00002048940194,1.00001712140523,1.00000000159591))
REPRESENTATION_ITEM('')
);
#1163=(
BOUNDED_CURVE()
B_SPLINE_CURVE(2,(#25689,#25690,#25691),.UNSPECIFIED.,.F.,.F.)
B_SPLINE_CURVE_WITH_KNOTS((3,3),(7.86559623322606E-6,0.0612396373727938),
 .UNSPECIFIED.)
CURVE()
GEOMETRIC_REPRESENTATION_ITEM()
RATIONAL_B_SPLINE_CURVE((1.0000191574532,1.07458139657236,1.05821963517921))
REPRESENTATION_ITEM('')
);
#1164=(
BOUNDED_CURVE()
B_SPLINE_CURVE(2,(#25699,#25700,#25701),.UNSPECIFIED.,.F.,.F.)
B_SPLINE_CURVE_WITH_KNOTS((3,3),(2.06502884885516E-6,0.0443073288438225),
 .UNSPECIFIED.)
CURVE()
GEOMETRIC_REPRESENTATION_ITEM()
RATIONAL_B_SPLINE_CURVE((1.00000000159591,1.00001712141336,1.00002048941166))
REPRESENTATION_ITEM('')
);
#1165=(
BOUNDED_CURVE()
B_SPLINE_CURVE(2,(#25703,#25704,#25705),.UNSPECIFIED.,.F.,.F.)
B_SPLINE_CURVE_WITH_KNOTS((3,3),(0.0392023395450786,0.100434111321634),
 .UNSPECIFIED.)
CURVE()
GEOMETRIC_REPRESENTATION_ITEM()
RATIONAL_B_SPLINE_CURVE((1.05821963517908,1.07458139657221,1.00001915745319))
REPRESENTATION_ITEM('')
);
#1166=(
BOUNDED_CURVE()
B_SPLINE_CURVE(2,(#25711,#25712,#25713),.UNSPECIFIED.,.F.,.F.)
B_SPLINE_CURVE_WITH_KNOTS((3,3),(0.0660091927118087,0.110314456526683),
 .UNSPECIFIED.)
CURVE()
GEOMETRIC_REPRESENTATION_ITEM()
RATIONAL_B_SPLINE_CURVE((1.00002048941584,1.00001712141684,1.00000000159591))
REPRESENTATION_ITEM('')
);
#1167=(
BOUNDED_CURVE()
B_SPLINE_CURVE(2,(#25731,#25732,#25733),.UNSPECIFIED.,.F.,.F.)
B_SPLINE_CURVE_WITH_KNOTS((3,3),(7.8655962357978E-6,0.061239637372792),
 .UNSPECIFIED.)
CURVE()
GEOMETRIC_REPRESENTATION_ITEM()
RATIONAL_B_SPLINE_CURVE((1.00001915745321,1.07458139657234,1.0582196351792))
REPRESENTATION_ITEM('')
);
#1168=(
BOUNDED_CURVE()
B_SPLINE_CURVE(2,(#25741,#25742,#25743),.UNSPECIFIED.,.F.,.F.)
B_SPLINE_CURVE_WITH_KNOTS((3,3),(2.06502885395743E-6,0.044307328843898),
 .UNSPECIFIED.)
CURVE()
GEOMETRIC_REPRESENTATION_ITEM()
RATIONAL_B_SPLINE_CURVE((1.00000000159591,1.00001712141084,1.00002048940865))
REPRESENTATION_ITEM('')
);
#1169=(
BOUNDED_CURVE()
B_SPLINE_CURVE(2,(#25745,#25746,#25747),.UNSPECIFIED.,.F.,.F.)
B_SPLINE_CURVE_WITH_KNOTS((3,3),(0.0392023395450774,0.100434111321634),
 .UNSPECIFIED.)
CURVE()
GEOMETRIC_REPRESENTATION_ITEM()
RATIONAL_B_SPLINE_CURVE((1.05821963517915,1.0745813965723,1.0000191574532))
REPRESENTATION_ITEM('')
);
#1170=(
BOUNDED_CURVE()
B_SPLINE_CURVE(2,(#25753,#25754,#25755),.UNSPECIFIED.,.F.,.F.)
B_SPLINE_CURVE_WITH_KNOTS((3,3),(0.0660091927117082,0.110314456526671),
 .UNSPECIFIED.)
CURVE()
GEOMETRIC_REPRESENTATION_ITEM()
RATIONAL_B_SPLINE_CURVE((1.00002048940984,1.00001712141184,1.00000000159591))
REPRESENTATION_ITEM('')
);
#1171=(
BOUNDED_CURVE()
B_SPLINE_CURVE(2,(#25773,#25774,#25775),.UNSPECIFIED.,.F.,.F.)
B_SPLINE_CURVE_WITH_KNOTS((3,3),(7.86559624864885E-6,0.0612396373728071),
 .UNSPECIFIED.)
CURVE()
GEOMETRIC_REPRESENTATION_ITEM()
RATIONAL_B_SPLINE_CURVE((1.00001915745324,1.07458139657234,1.05821963517919))
REPRESENTATION_ITEM('')
);
#1172=(
BOUNDED_CURVE()
B_SPLINE_CURVE(2,(#25783,#25784,#25785),.UNSPECIFIED.,.F.,.F.)
B_SPLINE_CURVE_WITH_KNOTS((3,3),(2.06499351570084E-6,0.0443065724918005),
 .UNSPECIFIED.)
CURVE()
GEOMETRIC_REPRESENTATION_ITEM()
RATIONAL_B_SPLINE_CURVE((1.00000000159957,1.00001716071775,1.00002056801743))
REPRESENTATION_ITEM('')
);
#1173=(
BOUNDED_CURVE()
B_SPLINE_CURVE(2,(#25787,#25788,#25789),.UNSPECIFIED.,.F.,.F.)
B_SPLINE_CURVE_WITH_KNOTS((3,3),(0.0392023395450912,0.100434111321662),
 .UNSPECIFIED.)
CURVE()
GEOMETRIC_REPRESENTATION_ITEM()
RATIONAL_B_SPLINE_CURVE((1.05821963517924,1.07458139657241,1.00001915745322))
REPRESENTATION_ITEM('')
);
#1174=(
BOUNDED_CURVE()
B_SPLINE_CURVE(2,(#25795,#25796,#25797),.UNSPECIFIED.,.F.,.F.)
B_SPLINE_CURVE_WITH_KNOTS((3,3),(0.0142112171255301,0.110567648737574),
 .UNSPECIFIED.)
CURVE()
GEOMETRIC_REPRESENTATION_ITEM()
RATIONAL_B_SPLINE_CURVE((1.00000961768267,1.00003742652563,1.0000001907435))
REPRESENTATION_ITEM('')
);
#1175=(
BOUNDED_CURVE()
B_SPLINE_CURVE(2,(#25865,#25866,#25867),.UNSPECIFIED.,.F.,.F.)
B_SPLINE_CURVE_WITH_KNOTS((3,3),(0.0662687847811601,0.110573269834452),
 .UNSPECIFIED.)
CURVE()
GEOMETRIC_REPRESENTATION_ITEM()
RATIONAL_B_SPLINE_CURVE((1.00002057034868,1.0000171618829,1.00000000159968))
REPRESENTATION_ITEM('')
);
#1176=(
BOUNDED_CURVE()
B_SPLINE_CURVE(2,(#25874,#25875,#25876),.UNSPECIFIED.,.F.,.F.)
B_SPLINE_CURVE_WITH_KNOTS((3,3),(7.86559624840906E-6,0.0612396373727937),
 .UNSPECIFIED.)
CURVE()
GEOMETRIC_REPRESENTATION_ITEM()
RATIONAL_B_SPLINE_CURVE((1.00001915745324,1.07458139657234,1.05821963517918))
REPRESENTATION_ITEM('')
);
#1177=(
BOUNDED_CURVE()
B_SPLINE_CURVE(2,(#25881,#25882,#25883),.UNSPECIFIED.,.F.,.F.)
B_SPLINE_CURVE_WITH_KNOTS((3,3),(0.0392023395450789,0.100434111321632),
 .UNSPECIFIED.)
CURVE()
GEOMETRIC_REPRESENTATION_ITEM()
RATIONAL_B_SPLINE_CURVE((1.05821963517911,1.07458139657224,1.00001915745322))
REPRESENTATION_ITEM('')
);
#1178=(
BOUNDED_CURVE()
B_SPLINE_CURVE(2,(#25901,#25902,#25903),.UNSPECIFIED.,.F.,.F.)
B_SPLINE_CURVE_WITH_KNOTS((3,3),(2.06502885157014E-6,0.0443073288439265),
 .UNSPECIFIED.)
CURVE()
GEOMETRIC_REPRESENTATION_ITEM()
RATIONAL_B_SPLINE_CURVE((1.00000000159591,1.00001712140936,1.00002048940688))
REPRESENTATION_ITEM('')
);
#1179=(
BOUNDED_CURVE()
B_SPLINE_CURVE(2,(#25907,#25908,#25909),.UNSPECIFIED.,.F.,.F.)
B_SPLINE_CURVE_WITH_KNOTS((3,3),(0.0660091927116283,0.110314456526686),
 .UNSPECIFIED.)
CURVE()
GEOMETRIC_REPRESENTATION_ITEM()
RATIONAL_B_SPLINE_CURVE((1.00002048940932,1.0000171214114,1.00000000159591))
REPRESENTATION_ITEM('')
);
#1180=(
BOUNDED_CURVE()
B_SPLINE_CURVE(2,(#25916,#25917,#25918),.UNSPECIFIED.,.F.,.F.)
B_SPLINE_CURVE_WITH_KNOTS((3,3),(7.86559624572803E-6,0.0612396373728016),
 .UNSPECIFIED.)
CURVE()
GEOMETRIC_REPRESENTATION_ITEM()
RATIONAL_B_SPLINE_CURVE((1.00001915745324,1.07458139657241,1.05821963517924))
REPRESENTATION_ITEM('')
);
#1181=(
BOUNDED_CURVE()
B_SPLINE_CURVE(2,(#25923,#25924,#25925),.UNSPECIFIED.,.F.,.F.)
B_SPLINE_CURVE_WITH_KNOTS((3,3),(0.0392023395450739,0.100434111321633),
 .UNSPECIFIED.)
CURVE()
GEOMETRIC_REPRESENTATION_ITEM()
RATIONAL_B_SPLINE_CURVE((1.05821963517925,1.07458139657243,1.00001915745321))
REPRESENTATION_ITEM('')
);
#1182=(
BOUNDED_CURVE()
B_SPLINE_CURVE(2,(#25943,#25944,#25945),.UNSPECIFIED.,.F.,.F.)
B_SPLINE_CURVE_WITH_KNOTS((3,3),(2.06502885149483E-6,0.0443073288439875),
 .UNSPECIFIED.)
CURVE()
GEOMETRIC_REPRESENTATION_ITEM()
RATIONAL_B_SPLINE_CURVE((1.00000000159591,1.00001712140408,1.00002048940056))
REPRESENTATION_ITEM('')
);
#1183=(
BOUNDED_CURVE()
B_SPLINE_CURVE(2,(#25949,#25950,#25951),.UNSPECIFIED.,.F.,.F.)
B_SPLINE_CURVE_WITH_KNOTS((3,3),(0.0660091927116748,0.110314456526719),
 .UNSPECIFIED.)
CURVE()
GEOMETRIC_REPRESENTATION_ITEM()
RATIONAL_B_SPLINE_CURVE((1.00002048940816,1.00001712141043,1.00000000159591))
REPRESENTATION_ITEM('')
);
#1184=(
BOUNDED_CURVE()
B_SPLINE_CURVE(2,(#25958,#25959,#25960),.UNSPECIFIED.,.F.,.F.)
B_SPLINE_CURVE_WITH_KNOTS((3,3),(7.86559623735724E-6,0.0612396373727826),
 .UNSPECIFIED.)
CURVE()
GEOMETRIC_REPRESENTATION_ITEM()
RATIONAL_B_SPLINE_CURVE((1.00001915745322,1.07458139657221,1.05821963517909))
REPRESENTATION_ITEM('')
);
#1185=(
BOUNDED_CURVE()
B_SPLINE_CURVE(2,(#25965,#25966,#25967),.UNSPECIFIED.,.F.,.F.)
B_SPLINE_CURVE_WITH_KNOTS((3,3),(0.03920233954508,0.100434111321635),
 .UNSPECIFIED.)
CURVE()
GEOMETRIC_REPRESENTATION_ITEM()
RATIONAL_B_SPLINE_CURVE((1.05821963517901,1.07458139657211,1.00001915745319))
REPRESENTATION_ITEM('')
);
#1186=(
BOUNDED_CURVE()
B_SPLINE_CURVE(2,(#25985,#25986,#25987),.UNSPECIFIED.,.F.,.F.)
B_SPLINE_CURVE_WITH_KNOTS((3,3),(2.06502885016307E-6,0.0443073288439128),
 .UNSPECIFIED.)
CURVE()
GEOMETRIC_REPRESENTATION_ITEM()
RATIONAL_B_SPLINE_CURVE((1.00000000159591,1.00001712140628,1.00002048940319))
REPRESENTATION_ITEM('')
);
#1187=(
BOUNDED_CURVE()
B_SPLINE_CURVE(2,(#25991,#25992,#25993),.UNSPECIFIED.,.F.,.F.)
B_SPLINE_CURVE_WITH_KNOTS((3,3),(0.0660091927116612,0.110314456526684),
 .UNSPECIFIED.)
CURVE()
GEOMETRIC_REPRESENTATION_ITEM()
RATIONAL_B_SPLINE_CURVE((1.0000204894059,1.00001712140854,1.00000000159591))
REPRESENTATION_ITEM('')
);
#1188=(
BOUNDED_CURVE()
B_SPLINE_CURVE(2,(#26000,#26001,#26002),.UNSPECIFIED.,.F.,.F.)
B_SPLINE_CURVE_WITH_KNOTS((3,3),(7.8655962337785E-6,0.0612396373727908),
 .UNSPECIFIED.)
CURVE()
GEOMETRIC_REPRESENTATION_ITEM()
RATIONAL_B_SPLINE_CURVE((1.00001915745321,1.0745813965724,1.05821963517924))
REPRESENTATION_ITEM('')
);
#1189=(
BOUNDED_CURVE()
B_SPLINE_CURVE(2,(#26007,#26008,#26009),.UNSPECIFIED.,.F.,.F.)
B_SPLINE_CURVE_WITH_KNOTS((3,3),(0.0392023395450855,0.100434111321653),
 .UNSPECIFIED.)
CURVE()
GEOMETRIC_REPRESENTATION_ITEM()
RATIONAL_B_SPLINE_CURVE((1.05821963517918,1.07458139657233,1.00001915745317))
REPRESENTATION_ITEM('')
);
#1190=(
BOUNDED_CURVE()
B_SPLINE_CURVE(2,(#26027,#26028,#26029),.UNSPECIFIED.,.F.,.F.)
B_SPLINE_CURVE_WITH_KNOTS((3,3),(2.06502884716521E-6,0.0443073288437792),
 .UNSPECIFIED.)
CURVE()
GEOMETRIC_REPRESENTATION_ITEM()
RATIONAL_B_SPLINE_CURVE((1.00000000159591,1.00001712141784,1.00002048941702))
REPRESENTATION_ITEM('')
);
#1191=(
BOUNDED_CURVE()
B_SPLINE_CURVE(2,(#26033,#26034,#26035),.UNSPECIFIED.,.F.,.F.)
B_SPLINE_CURVE_WITH_KNOTS((3,3),(0.0660091927116124,0.110314456526681),
 .UNSPECIFIED.)
CURVE()
GEOMETRIC_REPRESENTATION_ITEM()
RATIONAL_B_SPLINE_CURVE((1.00002048940556,1.00001712140826,1.00000000159591))
REPRESENTATION_ITEM('')
);
#1192=(
BOUNDED_CURVE()
B_SPLINE_CURVE(2,(#26042,#26043,#26044),.UNSPECIFIED.,.F.,.F.)
B_SPLINE_CURVE_WITH_KNOTS((3,3),(7.8655962373003E-6,0.0612396373727924),
 .UNSPECIFIED.)
CURVE()
GEOMETRIC_REPRESENTATION_ITEM()
RATIONAL_B_SPLINE_CURVE((1.00001915745321,1.07458139657233,1.05821963517918))
REPRESENTATION_ITEM('')
);
#1193=(
BOUNDED_CURVE()
B_SPLINE_CURVE(2,(#26049,#26050,#26051),.UNSPECIFIED.,.F.,.F.)
B_SPLINE_CURVE_WITH_KNOTS((3,3),(0.0392023395450769,0.100434111321635),
 .UNSPECIFIED.)
CURVE()
GEOMETRIC_REPRESENTATION_ITEM()
RATIONAL_B_SPLINE_CURVE((1.05821963517911,1.07458139657225,1.00001915745319))
REPRESENTATION_ITEM('')
);
#1194=(
BOUNDED_CURVE()
B_SPLINE_CURVE(2,(#26067,#26068,#26069),.UNSPECIFIED.,.F.,.F.)
B_SPLINE_CURVE_WITH_KNOTS((3,3),(0.0142112171257825,0.110567648737571),
 .UNSPECIFIED.)
CURVE()
GEOMETRIC_REPRESENTATION_ITEM()
RATIONAL_B_SPLINE_CURVE((1.00000961767676,1.00003742650262,1.00000019074339))
REPRESENTATION_ITEM('')
);
#1195=(
BOUNDED_CURVE()
B_SPLINE_CURVE(2,(#26086,#26087,#26088),.UNSPECIFIED.,.F.,.F.)
B_SPLINE_CURVE_WITH_KNOTS((3,3),(0.000246247416175026,0.0445514940289875),
 .UNSPECIFIED.)
CURVE()
GEOMETRIC_REPRESENTATION_ITEM()
RATIONAL_B_SPLINE_CURVE((1.0000001907434,1.00001731196304,1.00002068136573))
REPRESENTATION_ITEM('')
);
#1196=(
BOUNDED_CURVE()
B_SPLINE_CURVE(2,(#26098,#26099,#26100),.UNSPECIFIED.,.F.,.F.)
B_SPLINE_CURVE_WITH_KNOTS((3,3),(0.000246247416182682,0.0966026790274295),
 .UNSPECIFIED.)
CURVE()
GEOMETRIC_REPRESENTATION_ITEM()
RATIONAL_B_SPLINE_CURVE((1.00000019074342,1.00003742650901,1.0000096176784))
REPRESENTATION_ITEM('')
);
#1197=(
BOUNDED_CURVE()
B_SPLINE_CURVE(2,(#26106,#26107,#26108),.UNSPECIFIED.,.F.,.F.)
B_SPLINE_CURVE_WITH_KNOTS((3,3),(0.0662624021247521,0.110567648737547),
 .UNSPECIFIED.)
CURVE()
GEOMETRIC_REPRESENTATION_ITEM()
RATIONAL_B_SPLINE_CURVE((1.00002068137426,1.00001731197018,1.00000019074348))
REPRESENTATION_ITEM('')
);
#1198=(
BOUNDED_CURVE()
B_SPLINE_CURVE(2,(#26126,#26127,#26128),.UNSPECIFIED.,.F.,.F.)
B_SPLINE_CURVE_WITH_KNOTS((3,3),(7.86559623455466E-6,0.0612396373727871),
 .UNSPECIFIED.)
CURVE()
GEOMETRIC_REPRESENTATION_ITEM()
RATIONAL_B_SPLINE_CURVE((1.00001915745321,1.07458139657209,1.058219635179))
REPRESENTATION_ITEM('')
);
#1199=(
BOUNDED_CURVE()
B_SPLINE_CURVE(2,(#26136,#26137,#26138),.UNSPECIFIED.,.F.,.F.)
B_SPLINE_CURVE_WITH_KNOTS((3,3),(2.06502884828757E-6,0.0443073288439917),
 .UNSPECIFIED.)
CURVE()
GEOMETRIC_REPRESENTATION_ITEM()
RATIONAL_B_SPLINE_CURVE((1.00000000159591,1.00001712140454,1.00002048940111))
REPRESENTATION_ITEM('')
);
#1200=(
BOUNDED_CURVE()
B_SPLINE_CURVE(2,(#26140,#26141,#26142),.UNSPECIFIED.,.F.,.F.)
B_SPLINE_CURVE_WITH_KNOTS((3,3),(0.0392023395450789,0.100434111321635),
 .UNSPECIFIED.)
CURVE()
GEOMETRIC_REPRESENTATION_ITEM()
RATIONAL_B_SPLINE_CURVE((1.05821963517905,1.07458139657217,1.0000191574532))
REPRESENTATION_ITEM('')
);
#1201=(
BOUNDED_CURVE()
B_SPLINE_CURVE(2,(#26148,#26149,#26150),.UNSPECIFIED.,.F.,.F.)
B_SPLINE_CURVE_WITH_KNOTS((3,3),(0.0660091927117031,0.110314456526714),
 .UNSPECIFIED.)
CURVE()
GEOMETRIC_REPRESENTATION_ITEM()
RATIONAL_B_SPLINE_CURVE((1.00002048941073,1.00001712141258,1.00000000159591))
REPRESENTATION_ITEM('')
);
#1202=(
BOUNDED_CURVE()
B_SPLINE_CURVE(2,(#26168,#26169,#26170),.UNSPECIFIED.,.F.,.F.)
B_SPLINE_CURVE_WITH_KNOTS((3,3),(7.8655962436939E-6,0.0612396373727877),
 .UNSPECIFIED.)
CURVE()
GEOMETRIC_REPRESENTATION_ITEM()
RATIONAL_B_SPLINE_CURVE((1.00001915745323,1.07458139657225,1.05821963517912))
REPRESENTATION_ITEM('')
);
#1203=(
BOUNDED_CURVE()
B_SPLINE_CURVE(2,(#26178,#26179,#26180),.UNSPECIFIED.,.F.,.F.)
B_SPLINE_CURVE_WITH_KNOTS((3,3),(2.06502885453414E-6,0.0443073288439499),
 .UNSPECIFIED.)
CURVE()
GEOMETRIC_REPRESENTATION_ITEM()
RATIONAL_B_SPLINE_CURVE((1.00000000159591,1.00001712140702,1.00002048940408))
REPRESENTATION_ITEM('')
);
#1204=(
BOUNDED_CURVE()
B_SPLINE_CURVE(2,(#26182,#26183,#26184),.UNSPECIFIED.,.F.,.F.)
B_SPLINE_CURVE_WITH_KNOTS((3,3),(0.0392023395450765,0.100434111321633),
 .UNSPECIFIED.)
CURVE()
GEOMETRIC_REPRESENTATION_ITEM()
RATIONAL_B_SPLINE_CURVE((1.0582196351791,1.07458139657223,1.00001915745321))
REPRESENTATION_ITEM('')
);
#1205=(
BOUNDED_CURVE()
B_SPLINE_CURVE(2,(#26190,#26191,#26192),.UNSPECIFIED.,.F.,.F.)
B_SPLINE_CURVE_WITH_KNOTS((3,3),(0.0660091927116513,0.110314456526682),
 .UNSPECIFIED.)
CURVE()
GEOMETRIC_REPRESENTATION_ITEM()
RATIONAL_B_SPLINE_CURVE((1.00002048940269,1.00001712140586,1.00000000159591))
REPRESENTATION_ITEM('')
);
#1206=(
BOUNDED_CURVE()
B_SPLINE_CURVE(2,(#26210,#26211,#26212),.UNSPECIFIED.,.F.,.F.)
B_SPLINE_CURVE_WITH_KNOTS((3,3),(7.86559624777047E-6,0.0612396373728002),
 .UNSPECIFIED.)
CURVE()
GEOMETRIC_REPRESENTATION_ITEM()
RATIONAL_B_SPLINE_CURVE((1.00001915745324,1.0745813965723,1.05821963517915))
REPRESENTATION_ITEM('')
);
#1207=(
BOUNDED_CURVE()
B_SPLINE_CURVE(2,(#26220,#26221,#26222),.UNSPECIFIED.,.F.,.F.)
B_SPLINE_CURVE_WITH_KNOTS((3,3),(2.06499351625639E-6,0.0443065724919249),
 .UNSPECIFIED.)
CURVE()
GEOMETRIC_REPRESENTATION_ITEM()
RATIONAL_B_SPLINE_CURVE((1.00000000159957,1.00001716071701,1.00002056801654))
REPRESENTATION_ITEM('')
);
#1208=(
BOUNDED_CURVE()
B_SPLINE_CURVE(2,(#26224,#26225,#26226),.UNSPECIFIED.,.F.,.F.)
B_SPLINE_CURVE_WITH_KNOTS((3,3),(0.0392023395450864,0.100434111321651),
 .UNSPECIFIED.)
CURVE()
GEOMETRIC_REPRESENTATION_ITEM()
RATIONAL_B_SPLINE_CURVE((1.05821963517911,1.07458139657224,1.0000191574532))
REPRESENTATION_ITEM('')
);
#1209=(
BOUNDED_CURVE()
B_SPLINE_CURVE(2,(#26232,#26233,#26234),.UNSPECIFIED.,.F.,.F.)
B_SPLINE_CURVE_WITH_KNOTS((3,3),(0.0142112171256077,0.110567648737539),
 .UNSPECIFIED.)
CURVE()
GEOMETRIC_REPRESENTATION_ITEM()
RATIONAL_B_SPLINE_CURVE((1.00000961767965,1.00003742651388,1.00000019074344))
REPRESENTATION_ITEM('')
);
#1210=(
BOUNDED_CURVE()
B_SPLINE_CURVE(2,(#26304,#26305,#26306),.UNSPECIFIED.,.F.,.F.)
B_SPLINE_CURVE_WITH_KNOTS((3,3),(0.0662606539245541,0.110565163369947),
 .UNSPECIFIED.)
CURVE()
GEOMETRIC_REPRESENTATION_ITEM()
RATIONAL_B_SPLINE_CURVE((1.00002056780968,1.00001716061207,1.00000000159956))
REPRESENTATION_ITEM('')
);
#1211=(
BOUNDED_CURVE()
B_SPLINE_CURVE(2,(#26313,#26314,#26315),.UNSPECIFIED.,.F.,.F.)
B_SPLINE_CURVE_WITH_KNOTS((3,3),(7.86559623941073E-6,0.0612396373727952),
 .UNSPECIFIED.)
CURVE()
GEOMETRIC_REPRESENTATION_ITEM()
RATIONAL_B_SPLINE_CURVE((1.00001915745322,1.07458139657236,1.0582196351792))
REPRESENTATION_ITEM('')
);
#1212=(
BOUNDED_CURVE()
B_SPLINE_CURVE(2,(#26320,#26321,#26322),.UNSPECIFIED.,.F.,.F.)
B_SPLINE_CURVE_WITH_KNOTS((3,3),(0.0392023395450859,0.100434111321652),
 .UNSPECIFIED.)
CURVE()
GEOMETRIC_REPRESENTATION_ITEM()
RATIONAL_B_SPLINE_CURVE((1.05821963517913,1.07458139657226,1.0000191574532))
REPRESENTATION_ITEM('')
);
#1213=(
BOUNDED_CURVE()
B_SPLINE_CURVE(2,(#26340,#26341,#26342),.UNSPECIFIED.,.F.,.F.)
B_SPLINE_CURVE_WITH_KNOTS((3,3),(2.06502885201139E-6,0.0443073288438582),
 .UNSPECIFIED.)
CURVE()
GEOMETRIC_REPRESENTATION_ITEM()
RATIONAL_B_SPLINE_CURVE((1.00000000159591,1.00001712141177,1.00002048940977))
REPRESENTATION_ITEM('')
);
#1214=(
BOUNDED_CURVE()
B_SPLINE_CURVE(2,(#26347,#26348,#26349),.UNSPECIFIED.,.F.,.F.)
B_SPLINE_CURVE_WITH_KNOTS((3,3),(0.0660091927115239,0.110314456526711),
 .UNSPECIFIED.)
CURVE()
GEOMETRIC_REPRESENTATION_ITEM()
RATIONAL_B_SPLINE_CURVE((1.00002048939877,1.00001712140258,1.00000000159591))
REPRESENTATION_ITEM('')
);
#1215=(
BOUNDED_CURVE()
B_SPLINE_CURVE(2,(#26361,#26362,#26363),.UNSPECIFIED.,.F.,.F.)
B_SPLINE_CURVE_WITH_KNOTS((3,3),(7.86559624532228E-6,0.0612396373727895),
 .UNSPECIFIED.)
CURVE()
GEOMETRIC_REPRESENTATION_ITEM()
RATIONAL_B_SPLINE_CURVE((1.00001915745323,1.07458139657214,1.05821963517903))
REPRESENTATION_ITEM('')
);
#1216=(
BOUNDED_CURVE()
B_SPLINE_CURVE(2,(#26368,#26369,#26370),.UNSPECIFIED.,.F.,.F.)
B_SPLINE_CURVE_WITH_KNOTS((3,3),(0.0392023395450881,0.100434111321656),
 .UNSPECIFIED.)
CURVE()
GEOMETRIC_REPRESENTATION_ITEM()
RATIONAL_B_SPLINE_CURVE((1.05821963517912,1.07458139657226,1.00001915745319))
REPRESENTATION_ITEM('')
);
#1217=(
BOUNDED_CURVE()
B_SPLINE_CURVE(2,(#26384,#26385,#26386),.UNSPECIFIED.,.F.,.F.)
B_SPLINE_CURVE_WITH_KNOTS((3,3),(2.06502884911628E-6,0.0443073288438737),
 .UNSPECIFIED.)
CURVE()
GEOMETRIC_REPRESENTATION_ITEM()
RATIONAL_B_SPLINE_CURVE((1.00000000159591,1.00001712140897,1.00002048940641))
REPRESENTATION_ITEM('')
);
#1218=(
BOUNDED_CURVE()
B_SPLINE_CURVE(2,(#26390,#26391,#26392),.UNSPECIFIED.,.F.,.F.)
B_SPLINE_CURVE_WITH_KNOTS((3,3),(0.0660091927116664,0.110314456526713),
 .UNSPECIFIED.)
CURVE()
GEOMETRIC_REPRESENTATION_ITEM()
RATIONAL_B_SPLINE_CURVE((1.0000204894019,1.0000171214052,1.00000000159591))
REPRESENTATION_ITEM('')
);
#1219=(
BOUNDED_CURVE()
B_SPLINE_CURVE(2,(#26399,#26400,#26401),.UNSPECIFIED.,.F.,.F.)
B_SPLINE_CURVE_WITH_KNOTS((3,3),(7.86559624159626E-6,0.0612396373727846),
 .UNSPECIFIED.)
CURVE()
GEOMETRIC_REPRESENTATION_ITEM()
RATIONAL_B_SPLINE_CURVE((1.00001915745323,1.07458139657216,1.05821963517905))
REPRESENTATION_ITEM('')
);
#1220=(
BOUNDED_CURVE()
B_SPLINE_CURVE(2,(#26406,#26407,#26408),.UNSPECIFIED.,.F.,.F.)
B_SPLINE_CURVE_WITH_KNOTS((3,3),(0.0392023395450783,0.100434111321637),
 .UNSPECIFIED.)
CURVE()
GEOMETRIC_REPRESENTATION_ITEM()
RATIONAL_B_SPLINE_CURVE((1.05821963517912,1.07458139657226,1.00001915745319))
REPRESENTATION_ITEM('')
);
#1221=(
BOUNDED_CURVE()
B_SPLINE_CURVE(2,(#26426,#26427,#26428),.UNSPECIFIED.,.F.,.F.)
B_SPLINE_CURVE_WITH_KNOTS((3,3),(2.06502885183502E-6,0.0443073288439655),
 .UNSPECIFIED.)
CURVE()
GEOMETRIC_REPRESENTATION_ITEM()
RATIONAL_B_SPLINE_CURVE((1.00000000159591,1.00001712140387,1.00002048940031))
REPRESENTATION_ITEM('')
);
#1222=(
BOUNDED_CURVE()
B_SPLINE_CURVE(2,(#26432,#26433,#26434),.UNSPECIFIED.,.F.,.F.)
B_SPLINE_CURVE_WITH_KNOTS((3,3),(0.0660091927116195,0.110314456526666),
 .UNSPECIFIED.)
CURVE()
GEOMETRIC_REPRESENTATION_ITEM()
RATIONAL_B_SPLINE_CURVE((1.00002048940356,1.00001712140659,1.00000000159591))
REPRESENTATION_ITEM('')
);
#1223=(
BOUNDED_CURVE()
B_SPLINE_CURVE(2,(#26441,#26442,#26443),.UNSPECIFIED.,.F.,.F.)
B_SPLINE_CURVE_WITH_KNOTS((3,3),(7.8655962358422E-6,0.0612396373727976),
 .UNSPECIFIED.)
CURVE()
GEOMETRIC_REPRESENTATION_ITEM()
RATIONAL_B_SPLINE_CURVE((1.00001915745321,1.07458139657234,1.05821963517919))
REPRESENTATION_ITEM('')
);
#1224=(
BOUNDED_CURVE()
B_SPLINE_CURVE(2,(#26448,#26449,#26450),.UNSPECIFIED.,.F.,.F.)
B_SPLINE_CURVE_WITH_KNOTS((3,3),(0.0392023395450768,0.100434111321634),
 .UNSPECIFIED.)
CURVE()
GEOMETRIC_REPRESENTATION_ITEM()
RATIONAL_B_SPLINE_CURVE((1.0582196351792,1.07458139657236,1.00001915745321))
REPRESENTATION_ITEM('')
);
#1225=(
BOUNDED_CURVE()
B_SPLINE_CURVE(2,(#26468,#26469,#26470),.UNSPECIFIED.,.F.,.F.)
B_SPLINE_CURVE_WITH_KNOTS((3,3),(2.06502884978542E-6,0.044307328843927),
 .UNSPECIFIED.)
CURVE()
GEOMETRIC_REPRESENTATION_ITEM()
RATIONAL_B_SPLINE_CURVE((1.00000000159591,1.00001712141206,1.00002048941012))
REPRESENTATION_ITEM('')
);
#1226=(
BOUNDED_CURVE()
B_SPLINE_CURVE(2,(#26474,#26475,#26476),.UNSPECIFIED.,.F.,.F.)
B_SPLINE_CURVE_WITH_KNOTS((3,3),(0.0660091927117639,0.110314456526716),
 .UNSPECIFIED.)
CURVE()
GEOMETRIC_REPRESENTATION_ITEM()
RATIONAL_B_SPLINE_CURVE((1.00002048941328,1.00001712141471,1.00000000159591))
REPRESENTATION_ITEM('')
);
#1227=(
BOUNDED_CURVE()
B_SPLINE_CURVE(2,(#26483,#26484,#26485),.UNSPECIFIED.,.F.,.F.)
B_SPLINE_CURVE_WITH_KNOTS((3,3),(7.86559624401459E-6,0.061239637372789),
 .UNSPECIFIED.)
CURVE()
GEOMETRIC_REPRESENTATION_ITEM()
RATIONAL_B_SPLINE_CURVE((1.00001915745323,1.07458139657231,1.05821963517916))
REPRESENTATION_ITEM('')
);
#1228=(
BOUNDED_CURVE()
B_SPLINE_CURVE(2,(#26490,#26491,#26492),.UNSPECIFIED.,.F.,.F.)
B_SPLINE_CURVE_WITH_KNOTS((3,3),(0.0392023395450879,0.100434111321656),
 .UNSPECIFIED.)
CURVE()
GEOMETRIC_REPRESENTATION_ITEM()
RATIONAL_B_SPLINE_CURVE((1.05821963517917,1.07458139657232,1.00001915745319))
REPRESENTATION_ITEM('')
);
#1229=(
BOUNDED_CURVE()
B_SPLINE_CURVE(2,(#26510,#26511,#26512),.UNSPECIFIED.,.F.,.F.)
B_SPLINE_CURVE_WITH_KNOTS((3,3),(2.06502884833352E-6,0.044307328843929),
 .UNSPECIFIED.)
CURVE()
GEOMETRIC_REPRESENTATION_ITEM()
RATIONAL_B_SPLINE_CURVE((1.00000000159591,1.00001712141061,1.00002048940837))
REPRESENTATION_ITEM('')
);
#1230=(
BOUNDED_CURVE()
B_SPLINE_CURVE(2,(#26516,#26517,#26518),.UNSPECIFIED.,.F.,.F.)
B_SPLINE_CURVE_WITH_KNOTS((3,3),(0.0660091927116832,0.110314456526714),
 .UNSPECIFIED.)
CURVE()
GEOMETRIC_REPRESENTATION_ITEM()
RATIONAL_B_SPLINE_CURVE((1.00002048940784,1.00001712141016,1.00000000159591))
REPRESENTATION_ITEM('')
);
#1231=(
BOUNDED_CURVE()
B_SPLINE_CURVE(2,(#26525,#26526,#26527),.UNSPECIFIED.,.F.,.F.)
B_SPLINE_CURVE_WITH_KNOTS((3,3),(7.86559624514939E-6,0.0612396373727892),
 .UNSPECIFIED.)
CURVE()
GEOMETRIC_REPRESENTATION_ITEM()
RATIONAL_B_SPLINE_CURVE((1.00001915745323,1.07458139657222,1.05821963517909))
REPRESENTATION_ITEM('')
);
#1232=(
BOUNDED_CURVE()
B_SPLINE_CURVE(2,(#26532,#26533,#26534),.UNSPECIFIED.,.F.,.F.)
B_SPLINE_CURVE_WITH_KNOTS((3,3),(0.0392023395450942,0.100434111321667),
 .UNSPECIFIED.)
CURVE()
GEOMETRIC_REPRESENTATION_ITEM()
RATIONAL_B_SPLINE_CURVE((1.05821963517916,1.0745813965723,1.00001915745317))
REPRESENTATION_ITEM('')
);
#1233=(
BOUNDED_CURVE()
B_SPLINE_CURVE(2,(#26550,#26551,#26552),.UNSPECIFIED.,.F.,.F.)
B_SPLINE_CURVE_WITH_KNOTS((3,3),(0.0142193842176284,0.11057581462524),
 .UNSPECIFIED.)
CURVE()
GEOMETRIC_REPRESENTATION_ITEM()
RATIONAL_B_SPLINE_CURVE((1.00000962398904,1.00003743271758,1.00000019685764))
REPRESENTATION_ITEM('')
);
#1234=(
BOUNDED_CURVE()
B_SPLINE_CURVE(2,(#26569,#26570,#26571),.UNSPECIFIED.,.F.,.F.)
B_SPLINE_CURVE_WITH_KNOTS((3,3),(0.000254122058504862,0.0445593681152428),
 .UNSPECIFIED.)
CURVE()
GEOMETRIC_REPRESENTATION_ITEM()
RATIONAL_B_SPLINE_CURVE((1.00000019685769,1.0000173181266,1.00002068757546))
REPRESENTATION_ITEM('')
);
#1235=(
BOUNDED_CURVE()
B_SPLINE_CURVE(2,(#26581,#26582,#26583),.UNSPECIFIED.,.F.,.F.)
B_SPLINE_CURVE_WITH_KNOTS((3,3),(0.000246247416175252,0.0966026790274265),
 .UNSPECIFIED.)
CURVE()
GEOMETRIC_REPRESENTATION_ITEM()
RATIONAL_B_SPLINE_CURVE((1.00000019074343,1.00003742651156,1.00000961767906))
REPRESENTATION_ITEM('')
);
#1236=(
BOUNDED_CURVE()
B_SPLINE_CURVE(2,(#26589,#26590,#26591),.UNSPECIFIED.,.F.,.F.)
B_SPLINE_CURVE_WITH_KNOTS((3,3),(0.0662624021247102,0.11056764873757),
 .UNSPECIFIED.)
CURVE()
GEOMETRIC_REPRESENTATION_ITEM()
RATIONAL_B_SPLINE_CURVE((1.00002068136862,1.00001731196546,1.00000019074343))
REPRESENTATION_ITEM('')
);
#1237=(
BOUNDED_CURVE()
B_SPLINE_CURVE(2,(#26609,#26610,#26611),.UNSPECIFIED.,.F.,.F.)
B_SPLINE_CURVE_WITH_KNOTS((3,3),(7.86559623933804E-6,0.0612396373727864),
 .UNSPECIFIED.)
CURVE()
GEOMETRIC_REPRESENTATION_ITEM()
RATIONAL_B_SPLINE_CURVE((1.00001915745322,1.07458139657227,1.05821963517913))
REPRESENTATION_ITEM('')
);
#1238=(
BOUNDED_CURVE()
B_SPLINE_CURVE(2,(#26619,#26620,#26621),.UNSPECIFIED.,.F.,.F.)
B_SPLINE_CURVE_WITH_KNOTS((3,3),(2.06502885193672E-6,0.0443073288438289),
 .UNSPECIFIED.)
CURVE()
GEOMETRIC_REPRESENTATION_ITEM()
RATIONAL_B_SPLINE_CURVE((1.00000000159591,1.00001712141026,1.00002048940795))
REPRESENTATION_ITEM('')
);
#1239=(
BOUNDED_CURVE()
B_SPLINE_CURVE(2,(#26623,#26624,#26625),.UNSPECIFIED.,.F.,.F.)
B_SPLINE_CURVE_WITH_KNOTS((3,3),(0.0392023395450853,0.10043411132165),
 .UNSPECIFIED.)
CURVE()
GEOMETRIC_REPRESENTATION_ITEM()
RATIONAL_B_SPLINE_CURVE((1.05821963517918,1.07458139657234,1.00001915745322))
REPRESENTATION_ITEM('')
);
#1240=(
BOUNDED_CURVE()
B_SPLINE_CURVE(2,(#26631,#26632,#26633),.UNSPECIFIED.,.F.,.F.)
B_SPLINE_CURVE_WITH_KNOTS((3,3),(0.0660091927116699,0.110314456526683),
 .UNSPECIFIED.)
CURVE()
GEOMETRIC_REPRESENTATION_ITEM()
RATIONAL_B_SPLINE_CURVE((1.00002048940987,1.00001712141186,1.00000000159591))
REPRESENTATION_ITEM('')
);
#1241=(
BOUNDED_CURVE()
B_SPLINE_CURVE(2,(#26651,#26652,#26653),.UNSPECIFIED.,.F.,.F.)
B_SPLINE_CURVE_WITH_KNOTS((3,3),(7.86559624078655E-6,0.061239637372796),
 .UNSPECIFIED.)
CURVE()
GEOMETRIC_REPRESENTATION_ITEM()
RATIONAL_B_SPLINE_CURVE((1.00001915745322,1.07458139657237,1.05821963517922))
REPRESENTATION_ITEM('')
);
#1242=(
BOUNDED_CURVE()
B_SPLINE_CURVE(2,(#26661,#26662,#26663),.UNSPECIFIED.,.F.,.F.)
B_SPLINE_CURVE_WITH_KNOTS((3,3),(2.06499351893339E-6,0.0443065724918821),
 .UNSPECIFIED.)
CURVE()
GEOMETRIC_REPRESENTATION_ITEM()
RATIONAL_B_SPLINE_CURVE((1.00000000159957,1.0000171607139,1.00002056801282))
REPRESENTATION_ITEM('')
);
#1243=(
BOUNDED_CURVE()
B_SPLINE_CURVE(2,(#26665,#26666,#26667),.UNSPECIFIED.,.F.,.F.)
B_SPLINE_CURVE_WITH_KNOTS((3,3),(0.0392023395450775,0.100434111321634),
 .UNSPECIFIED.)
CURVE()
GEOMETRIC_REPRESENTATION_ITEM()
RATIONAL_B_SPLINE_CURVE((1.05821963517913,1.07458139657227,1.0000191574532))
REPRESENTATION_ITEM('')
);
#1244=(
BOUNDED_CURVE()
B_SPLINE_CURVE(2,(#26673,#26674,#26675),.UNSPECIFIED.,.F.,.F.)
B_SPLINE_CURVE_WITH_KNOTS((3,3),(0.0142112171257224,0.11056764873754),
 .UNSPECIFIED.)
CURVE()
GEOMETRIC_REPRESENTATION_ITEM()
RATIONAL_B_SPLINE_CURVE((1.00000961767654,1.00003742650177,1.00000019074338))
REPRESENTATION_ITEM('')
);
#1245=(
BOUNDED_CURVE()
B_SPLINE_CURVE(2,(#26743,#26744,#26745),.UNSPECIFIED.,.F.,.F.)
B_SPLINE_CURVE_WITH_KNOTS((3,3),(0.0662687847811842,0.110573269834456),
 .UNSPECIFIED.)
CURVE()
GEOMETRIC_REPRESENTATION_ITEM()
RATIONAL_B_SPLINE_CURVE((1.00002057034848,1.00001716188273,1.00000000159968))
REPRESENTATION_ITEM('')
);
#1246=(
BOUNDED_CURVE()
B_SPLINE_CURVE(2,(#26752,#26753,#26754),.UNSPECIFIED.,.F.,.F.)
B_SPLINE_CURVE_WITH_KNOTS((3,3),(7.86559623619297E-6,0.06123963737278),
 .UNSPECIFIED.)
CURVE()
GEOMETRIC_REPRESENTATION_ITEM()
RATIONAL_B_SPLINE_CURVE((1.00001915745321,1.0745813965721,1.058219635179))
REPRESENTATION_ITEM('')
);
#1247=(
BOUNDED_CURVE()
B_SPLINE_CURVE(2,(#26759,#26760,#26761),.UNSPECIFIED.,.F.,.F.)
B_SPLINE_CURVE_WITH_KNOTS((3,3),(0.039202339545078,0.100434111321636),
 .UNSPECIFIED.)
CURVE()
GEOMETRIC_REPRESENTATION_ITEM()
RATIONAL_B_SPLINE_CURVE((1.05821963517909,1.07458139657222,1.0000191574532))
REPRESENTATION_ITEM('')
);
#1248=(
BOUNDED_CURVE()
B_SPLINE_CURVE(2,(#26779,#26780,#26781),.UNSPECIFIED.,.F.,.F.)
B_SPLINE_CURVE_WITH_KNOTS((3,3),(2.06502885056018E-6,0.0443073288440188),
 .UNSPECIFIED.)
CURVE()
GEOMETRIC_REPRESENTATION_ITEM()
RATIONAL_B_SPLINE_CURVE((1.00000000159591,1.00001712140584,1.00002048940267))
REPRESENTATION_ITEM('')
);
#1249=(
BOUNDED_CURVE()
B_SPLINE_CURVE(2,(#26785,#26786,#26787),.UNSPECIFIED.,.F.,.F.)
B_SPLINE_CURVE_WITH_KNOTS((3,3),(0.0660091927117243,0.110314456526684),
 .UNSPECIFIED.)
CURVE()
GEOMETRIC_REPRESENTATION_ITEM()
RATIONAL_B_SPLINE_CURVE((1.00002048940642,1.00001712140897,1.00000000159591))
REPRESENTATION_ITEM('')
);
#1250=(
BOUNDED_CURVE()
B_SPLINE_CURVE(2,(#26794,#26795,#26796),.UNSPECIFIED.,.F.,.F.)
B_SPLINE_CURVE_WITH_KNOTS((3,3),(7.86559624052001E-6,0.0612396373727947),
 .UNSPECIFIED.)
CURVE()
GEOMETRIC_REPRESENTATION_ITEM()
RATIONAL_B_SPLINE_CURVE((1.00001915745322,1.0745813965723,1.05821963517916))
REPRESENTATION_ITEM('')
);
#1251=(
BOUNDED_CURVE()
B_SPLINE_CURVE(2,(#26801,#26802,#26803),.UNSPECIFIED.,.F.,.F.)
B_SPLINE_CURVE_WITH_KNOTS((3,3),(0.0392023395450857,0.100434111321653),
 .UNSPECIFIED.)
CURVE()
GEOMETRIC_REPRESENTATION_ITEM()
RATIONAL_B_SPLINE_CURVE((1.05821963517924,1.0745813965724,1.0000191574532))
REPRESENTATION_ITEM('')
);
#1252=(
BOUNDED_CURVE()
B_SPLINE_CURVE(2,(#26821,#26822,#26823),.UNSPECIFIED.,.F.,.F.)
B_SPLINE_CURVE_WITH_KNOTS((3,3),(2.0650288503503E-6,0.0443073288439064),
 .UNSPECIFIED.)
CURVE()
GEOMETRIC_REPRESENTATION_ITEM()
RATIONAL_B_SPLINE_CURVE((1.00000000159591,1.00001712140843,1.00002048940577))
REPRESENTATION_ITEM('')
);
#1253=(
BOUNDED_CURVE()
B_SPLINE_CURVE(2,(#26827,#26828,#26829),.UNSPECIFIED.,.F.,.F.)
B_SPLINE_CURVE_WITH_KNOTS((3,3),(0.0660091927115479,0.110314456526717),
 .UNSPECIFIED.)
CURVE()
GEOMETRIC_REPRESENTATION_ITEM()
RATIONAL_B_SPLINE_CURVE((1.00002048940187,1.00001712140517,1.00000000159591))
REPRESENTATION_ITEM('')
);
#1254=(
BOUNDED_CURVE()
B_SPLINE_CURVE(2,(#26836,#26837,#26838),.UNSPECIFIED.,.F.,.F.)
B_SPLINE_CURVE_WITH_KNOTS((3,3),(7.86559623675799E-6,0.0612396373727838),
 .UNSPECIFIED.)
CURVE()
GEOMETRIC_REPRESENTATION_ITEM()
RATIONAL_B_SPLINE_CURVE((1.00001915745321,1.07458139657228,1.05821963517914))
REPRESENTATION_ITEM('')
);
#1255=(
BOUNDED_CURVE()
B_SPLINE_CURVE(2,(#26843,#26844,#26845),.UNSPECIFIED.,.F.,.F.)
B_SPLINE_CURVE_WITH_KNOTS((3,3),(0.0392023395450765,0.100434111321632),
 .UNSPECIFIED.)
CURVE()
GEOMETRIC_REPRESENTATION_ITEM()
RATIONAL_B_SPLINE_CURVE((1.05821963517912,1.07458139657226,1.00001915745321))
REPRESENTATION_ITEM('')
);
#1256=(
BOUNDED_CURVE()
B_SPLINE_CURVE(2,(#26863,#26864,#26865),.UNSPECIFIED.,.F.,.F.)
B_SPLINE_CURVE_WITH_KNOTS((3,3),(2.06502885377429E-6,0.0443073288438915),
 .UNSPECIFIED.)
CURVE()
GEOMETRIC_REPRESENTATION_ITEM()
RATIONAL_B_SPLINE_CURVE((1.00000000159591,1.00001712141336,1.00002048941167))
REPRESENTATION_ITEM('')
);
#1257=(
BOUNDED_CURVE()
B_SPLINE_CURVE(2,(#26869,#26870,#26871),.UNSPECIFIED.,.F.,.F.)
B_SPLINE_CURVE_WITH_KNOTS((3,3),(0.0660091927116458,0.110314456526714),
 .UNSPECIFIED.)
CURVE()
GEOMETRIC_REPRESENTATION_ITEM()
RATIONAL_B_SPLINE_CURVE((1.000020489408,1.0000171214103,1.00000000159591))
REPRESENTATION_ITEM('')
);
#1258=(
BOUNDED_CURVE()
B_SPLINE_CURVE(2,(#26878,#26879,#26880),.UNSPECIFIED.,.F.,.F.)
B_SPLINE_CURVE_WITH_KNOTS((3,3),(7.86559625794864E-6,0.0612396373728014),
 .UNSPECIFIED.)
CURVE()
GEOMETRIC_REPRESENTATION_ITEM()
RATIONAL_B_SPLINE_CURVE((1.00001915745327,1.07458139657237,1.0582196351792))
REPRESENTATION_ITEM('')
);
#1259=(
BOUNDED_CURVE()
B_SPLINE_CURVE(2,(#26885,#26886,#26887),.UNSPECIFIED.,.F.,.F.)
B_SPLINE_CURVE_WITH_KNOTS((3,3),(0.0392023395450741,0.100434111321631),
 .UNSPECIFIED.)
CURVE()
GEOMETRIC_REPRESENTATION_ITEM()
RATIONAL_B_SPLINE_CURVE((1.05821963517911,1.07458139657226,1.00001915745322))
REPRESENTATION_ITEM('')
);
#1260=(
BOUNDED_CURVE()
B_SPLINE_CURVE(2,(#26905,#26906,#26907),.UNSPECIFIED.,.F.,.F.)
B_SPLINE_CURVE_WITH_KNOTS((3,3),(2.0650288534097E-6,0.0443073288438614),
 .UNSPECIFIED.)
CURVE()
GEOMETRIC_REPRESENTATION_ITEM()
RATIONAL_B_SPLINE_CURVE((1.00000000159591,1.00001712141325,1.00002048941153))
REPRESENTATION_ITEM('')
);
#1261=(
BOUNDED_CURVE()
B_SPLINE_CURVE(2,(#26911,#26912,#26913),.UNSPECIFIED.,.F.,.F.)
B_SPLINE_CURVE_WITH_KNOTS((3,3),(0.0660091927116462,0.110314456526715),
 .UNSPECIFIED.)
CURVE()
GEOMETRIC_REPRESENTATION_ITEM()
RATIONAL_B_SPLINE_CURVE((1.00002048940619,1.00001712140878,1.00000000159591))
REPRESENTATION_ITEM('')
);
#1262=(
BOUNDED_CURVE()
B_SPLINE_CURVE(2,(#26920,#26921,#26922),.UNSPECIFIED.,.F.,.F.)
B_SPLINE_CURVE_WITH_KNOTS((3,3),(7.86559624534418E-6,0.0612396373727898),
 .UNSPECIFIED.)
CURVE()
GEOMETRIC_REPRESENTATION_ITEM()
RATIONAL_B_SPLINE_CURVE((1.00001915745323,1.07458139657225,1.05821963517912))
REPRESENTATION_ITEM('')
);
#1263=(
BOUNDED_CURVE()
B_SPLINE_CURVE(2,(#26927,#26928,#26929),.UNSPECIFIED.,.F.,.F.)
B_SPLINE_CURVE_WITH_KNOTS((3,3),(0.039202339545079,0.100434111321632),
 .UNSPECIFIED.)
CURVE()
GEOMETRIC_REPRESENTATION_ITEM()
RATIONAL_B_SPLINE_CURVE((1.05821963517908,1.0745813965722,1.00001915745321))
REPRESENTATION_ITEM('')
);
#1264=(
BOUNDED_CURVE()
B_SPLINE_CURVE(2,(#26947,#26948,#26949),.UNSPECIFIED.,.F.,.F.)
B_SPLINE_CURVE_WITH_KNOTS((3,3),(2.06502885096946E-6,0.0443073288439515),
 .UNSPECIFIED.)
CURVE()
GEOMETRIC_REPRESENTATION_ITEM()
RATIONAL_B_SPLINE_CURVE((1.00000000159591,1.00001712140919,1.00002048940668))
REPRESENTATION_ITEM('')
);
#1265=(
BOUNDED_CURVE()
B_SPLINE_CURVE(2,(#26953,#26954,#26955),.UNSPECIFIED.,.F.,.F.)
B_SPLINE_CURVE_WITH_KNOTS((3,3),(0.0660091927116946,0.110314456526713),
 .UNSPECIFIED.)
CURVE()
GEOMETRIC_REPRESENTATION_ITEM()
RATIONAL_B_SPLINE_CURVE((1.00002048940625,1.00001712140884,1.00000000159591))
REPRESENTATION_ITEM('')
);
#1266=(
BOUNDED_CURVE()
B_SPLINE_CURVE(2,(#26962,#26963,#26964),.UNSPECIFIED.,.F.,.F.)
B_SPLINE_CURVE_WITH_KNOTS((3,3),(7.86559624800839E-6,0.0612396373727904),
 .UNSPECIFIED.)
CURVE()
GEOMETRIC_REPRESENTATION_ITEM()
RATIONAL_B_SPLINE_CURVE((1.00001915745324,1.07458139657215,1.05821963517904))
REPRESENTATION_ITEM('')
);
#1267=(
BOUNDED_CURVE()
B_SPLINE_CURVE(2,(#26969,#26970,#26971),.UNSPECIFIED.,.F.,.F.)
B_SPLINE_CURVE_WITH_KNOTS((3,3),(0.0392023395450754,0.100434111321632),
 .UNSPECIFIED.)
CURVE()
GEOMETRIC_REPRESENTATION_ITEM()
RATIONAL_B_SPLINE_CURVE((1.05821963517914,1.07458139657228,1.00001915745321))
REPRESENTATION_ITEM('')
);
#1268=(
BOUNDED_CURVE()
B_SPLINE_CURVE(2,(#26989,#26990,#26991),.UNSPECIFIED.,.F.,.F.)
B_SPLINE_CURVE_WITH_KNOTS((3,3),(2.065028853533E-6,0.0443073288439286),
 .UNSPECIFIED.)
CURVE()
GEOMETRIC_REPRESENTATION_ITEM()
RATIONAL_B_SPLINE_CURVE((1.00000000159591,1.00001712140699,1.00002048940404))
REPRESENTATION_ITEM('')
);
#1269=(
BOUNDED_CURVE()
B_SPLINE_CURVE(2,(#26995,#26996,#26997),.UNSPECIFIED.,.F.,.F.)
B_SPLINE_CURVE_WITH_KNOTS((3,3),(0.0660091927117083,0.110314456526682),
 .UNSPECIFIED.)
CURVE()
GEOMETRIC_REPRESENTATION_ITEM()
RATIONAL_B_SPLINE_CURVE((1.00002048940433,1.00001712140723,1.00000000159591))
REPRESENTATION_ITEM('')
);
#1270=(
BOUNDED_CURVE()
B_SPLINE_CURVE(2,(#27004,#27005,#27006),.UNSPECIFIED.,.F.,.F.)
B_SPLINE_CURVE_WITH_KNOTS((3,3),(7.86559624267222E-6,0.0612396373727971),
 .UNSPECIFIED.)
CURVE()
GEOMETRIC_REPRESENTATION_ITEM()
RATIONAL_B_SPLINE_CURVE((1.00001915745323,1.07458139657241,1.05821963517925))
REPRESENTATION_ITEM('')
);
#1271=(
BOUNDED_CURVE()
B_SPLINE_CURVE(2,(#27011,#27012,#27013),.UNSPECIFIED.,.F.,.F.)
B_SPLINE_CURVE_WITH_KNOTS((3,3),(0.0392023395450862,0.100434111321654),
 .UNSPECIFIED.)
CURVE()
GEOMETRIC_REPRESENTATION_ITEM()
RATIONAL_B_SPLINE_CURVE((1.05821963517913,1.07458139657226,1.0000191574532))
REPRESENTATION_ITEM('')
);
#1272=(
BOUNDED_CURVE()
B_SPLINE_CURVE(2,(#27029,#27030,#27031),.UNSPECIFIED.,.F.,.F.)
B_SPLINE_CURVE_WITH_KNOTS((3,3),(0.0142112171255263,0.110567648737579),
 .UNSPECIFIED.)
CURVE()
GEOMETRIC_REPRESENTATION_ITEM()
RATIONAL_B_SPLINE_CURVE((1.00000961768216,1.00003742652363,1.00000019074349))
REPRESENTATION_ITEM('')
);
#1273=(
BOUNDED_CURVE()
B_SPLINE_CURVE(2,(#27048,#27049,#27050),.UNSPECIFIED.,.F.,.F.)
B_SPLINE_CURVE_WITH_KNOTS((3,3),(0.000246247416178109,0.0445514940289694),
 .UNSPECIFIED.)
CURVE()
GEOMETRIC_REPRESENTATION_ITEM()
RATIONAL_B_SPLINE_CURVE((1.0000001907434,1.00001731196283,1.00002068136548))
REPRESENTATION_ITEM('')
);
#1274=(
BOUNDED_CURVE()
B_SPLINE_CURVE(2,(#27060,#27061,#27062),.UNSPECIFIED.,.F.,.F.)
B_SPLINE_CURVE_WITH_KNOTS((3,3),(0.000246247416177958,0.0966026790273509),
 .UNSPECIFIED.)
CURVE()
GEOMETRIC_REPRESENTATION_ITEM()
RATIONAL_B_SPLINE_CURVE((1.00000019074342,1.00003742650884,1.00000961767836))
REPRESENTATION_ITEM('')
);
#1275=(
BOUNDED_CURVE()
B_SPLINE_CURVE(2,(#27068,#27069,#27070),.UNSPECIFIED.,.F.,.F.)
B_SPLINE_CURVE_WITH_KNOTS((3,3),(0.0662624021247137,0.110567648737539),
 .UNSPECIFIED.)
CURVE()
GEOMETRIC_REPRESENTATION_ITEM()
RATIONAL_B_SPLINE_CURVE((1.00002068136864,1.00001731196548,1.00000019074343))
REPRESENTATION_ITEM('')
);
#1276=(
BOUNDED_CURVE()
B_SPLINE_CURVE(2,(#27088,#27089,#27090),.UNSPECIFIED.,.F.,.F.)
B_SPLINE_CURVE_WITH_KNOTS((3,3),(7.86559624408066E-6,0.0612396373727953),
 .UNSPECIFIED.)
CURVE()
GEOMETRIC_REPRESENTATION_ITEM()
RATIONAL_B_SPLINE_CURVE((1.00001915745323,1.07458139657215,1.05821963517905))
REPRESENTATION_ITEM('')
);
#1277=(
BOUNDED_CURVE()
B_SPLINE_CURVE(2,(#27098,#27099,#27100),.UNSPECIFIED.,.F.,.F.)
B_SPLINE_CURVE_WITH_KNOTS((3,3),(2.06499351984749E-6,0.0443065724919119),
 .UNSPECIFIED.)
CURVE()
GEOMETRIC_REPRESENTATION_ITEM()
RATIONAL_B_SPLINE_CURVE((1.00000000159957,1.00001716071212,1.00002056801068))
REPRESENTATION_ITEM('')
);
#1278=(
BOUNDED_CURVE()
B_SPLINE_CURVE(2,(#27102,#27103,#27104),.UNSPECIFIED.,.F.,.F.)
B_SPLINE_CURVE_WITH_KNOTS((3,3),(0.039202339545086,0.100434111321651),
 .UNSPECIFIED.)
CURVE()
GEOMETRIC_REPRESENTATION_ITEM()
RATIONAL_B_SPLINE_CURVE((1.05821963517915,1.0745813965723,1.00001915745321))
REPRESENTATION_ITEM('')
);
#1279=(
BOUNDED_CURVE()
B_SPLINE_CURVE(2,(#27110,#27111,#27112),.UNSPECIFIED.,.F.,.F.)
B_SPLINE_CURVE_WITH_KNOTS((3,3),(0.0142112171256635,0.110567648737569),
 .UNSPECIFIED.)
CURVE()
GEOMETRIC_REPRESENTATION_ITEM()
RATIONAL_B_SPLINE_CURVE((1.00000961767905,1.00003742651155,1.00000019074343))
REPRESENTATION_ITEM('')
);
#1280=(
BOUNDED_CURVE()
B_SPLINE_CURVE(2,(#27182,#27183,#27184),.UNSPECIFIED.,.F.,.F.)
B_SPLINE_CURVE_WITH_KNOTS((3,3),(0.0662606539244983,0.110565163369973),
 .UNSPECIFIED.)
CURVE()
GEOMETRIC_REPRESENTATION_ITEM()
RATIONAL_B_SPLINE_CURVE((1.00002056781132,1.00001716061344,1.00000000159956))
REPRESENTATION_ITEM('')
);
#1281=(
BOUNDED_CURVE()
B_SPLINE_CURVE(2,(#27191,#27192,#27193),.UNSPECIFIED.,.F.,.F.)
B_SPLINE_CURVE_WITH_KNOTS((3,3),(7.86559624013797E-6,0.0612396373727866),
 .UNSPECIFIED.)
CURVE()
GEOMETRIC_REPRESENTATION_ITEM()
RATIONAL_B_SPLINE_CURVE((1.00001915745322,1.07458139657224,1.05821963517911))
REPRESENTATION_ITEM('')
);
#1282=(
BOUNDED_CURVE()
B_SPLINE_CURVE(2,(#27198,#27199,#27200),.UNSPECIFIED.,.F.,.F.)
B_SPLINE_CURVE_WITH_KNOTS((3,3),(0.0392023395450931,0.100434111321664),
 .UNSPECIFIED.)
CURVE()
GEOMETRIC_REPRESENTATION_ITEM()
RATIONAL_B_SPLINE_CURVE((1.05821963517915,1.07458139657229,1.0000191574532))
REPRESENTATION_ITEM('')
);
#1283=(
BOUNDED_CURVE()
B_SPLINE_CURVE(2,(#27218,#27219,#27220),.UNSPECIFIED.,.F.,.F.)
B_SPLINE_CURVE_WITH_KNOTS((3,3),(2.06502885237961E-6,0.0443073288438955),
 .UNSPECIFIED.)
CURVE()
GEOMETRIC_REPRESENTATION_ITEM()
RATIONAL_B_SPLINE_CURVE((1.00000000159591,1.00001712140489,1.00002048940153))
REPRESENTATION_ITEM('')
);
#1284=(
BOUNDED_CURVE()
B_SPLINE_CURVE(2,(#27224,#27225,#27226),.UNSPECIFIED.,.F.,.F.)
B_SPLINE_CURVE_WITH_KNOTS((3,3),(0.0660091927116133,0.110314456526713),
 .UNSPECIFIED.)
CURVE()
GEOMETRIC_REPRESENTATION_ITEM()
RATIONAL_B_SPLINE_CURVE((1.00002048940597,1.0000171214086,1.00000000159591))
REPRESENTATION_ITEM('')
);
#1285=(
BOUNDED_CURVE()
B_SPLINE_CURVE(2,(#27233,#27234,#27235),.UNSPECIFIED.,.F.,.F.)
B_SPLINE_CURVE_WITH_KNOTS((3,3),(7.86559624719566E-6,0.0612396373727914),
 .UNSPECIFIED.)
CURVE()
GEOMETRIC_REPRESENTATION_ITEM()
RATIONAL_B_SPLINE_CURVE((1.00001915745324,1.07458139657227,1.05821963517913))
REPRESENTATION_ITEM('')
);
#1286=(
BOUNDED_CURVE()
B_SPLINE_CURVE(2,(#27240,#27241,#27242),.UNSPECIFIED.,.F.,.F.)
B_SPLINE_CURVE_WITH_KNOTS((3,3),(0.0392023395450766,0.100434111321633),
 .UNSPECIFIED.)
CURVE()
GEOMETRIC_REPRESENTATION_ITEM()
RATIONAL_B_SPLINE_CURVE((1.05821963517913,1.07458139657227,1.0000191574532))
REPRESENTATION_ITEM('')
);
#1287=(
BOUNDED_CURVE()
B_SPLINE_CURVE(2,(#27260,#27261,#27262),.UNSPECIFIED.,.F.,.F.)
B_SPLINE_CURVE_WITH_KNOTS((3,3),(2.0650288492734E-6,0.0443073288439416),
 .UNSPECIFIED.)
CURVE()
GEOMETRIC_REPRESENTATION_ITEM()
RATIONAL_B_SPLINE_CURVE((1.00000000159591,1.00001712140949,1.00002048940704))
REPRESENTATION_ITEM('')
);
#1288=(
BOUNDED_CURVE()
B_SPLINE_CURVE(2,(#27266,#27267,#27268),.UNSPECIFIED.,.F.,.F.)
B_SPLINE_CURVE_WITH_KNOTS((3,3),(0.06600919271168,0.110314456526681),
 .UNSPECIFIED.)
CURVE()
GEOMETRIC_REPRESENTATION_ITEM()
RATIONAL_B_SPLINE_CURVE((1.00002048940869,1.00001712141088,1.00000000159591))
REPRESENTATION_ITEM('')
);
#1289=(
BOUNDED_CURVE()
B_SPLINE_CURVE(2,(#27275,#27276,#27277),.UNSPECIFIED.,.F.,.F.)
B_SPLINE_CURVE_WITH_KNOTS((3,3),(7.86559623979792E-6,0.0612396373727948),
 .UNSPECIFIED.)
CURVE()
GEOMETRIC_REPRESENTATION_ITEM()
RATIONAL_B_SPLINE_CURVE((1.00001915745322,1.0745813965724,1.05821963517924))
REPRESENTATION_ITEM('')
);
#1290=(
BOUNDED_CURVE()
B_SPLINE_CURVE(2,(#27282,#27283,#27284),.UNSPECIFIED.,.F.,.F.)
B_SPLINE_CURVE_WITH_KNOTS((3,3),(0.0392023395450884,0.100434111321653),
 .UNSPECIFIED.)
CURVE()
GEOMETRIC_REPRESENTATION_ITEM()
RATIONAL_B_SPLINE_CURVE((1.05821963517909,1.07458139657222,1.00001915745319))
REPRESENTATION_ITEM('')
);
#1291=(
BOUNDED_CURVE()
B_SPLINE_CURVE(2,(#27302,#27303,#27304),.UNSPECIFIED.,.F.,.F.)
B_SPLINE_CURVE_WITH_KNOTS((3,3),(2.06502884853687E-6,0.0443073288438766),
 .UNSPECIFIED.)
CURVE()
GEOMETRIC_REPRESENTATION_ITEM()
RATIONAL_B_SPLINE_CURVE((1.00000000159591,1.00001712141175,1.00002048940974))
REPRESENTATION_ITEM('')
);
#1292=(
BOUNDED_CURVE()
B_SPLINE_CURVE(2,(#27308,#27309,#27310),.UNSPECIFIED.,.F.,.F.)
B_SPLINE_CURVE_WITH_KNOTS((3,3),(0.0660091927116071,0.110314456526712),
 .UNSPECIFIED.)
CURVE()
GEOMETRIC_REPRESENTATION_ITEM()
RATIONAL_B_SPLINE_CURVE((1.00002048940052,1.00001712140405,1.00000000159591))
REPRESENTATION_ITEM('')
);
#1293=(
BOUNDED_CURVE()
B_SPLINE_CURVE(2,(#27317,#27318,#27319),.UNSPECIFIED.,.F.,.F.)
B_SPLINE_CURVE_WITH_KNOTS((3,3),(7.86559623158078E-6,0.0612396373727783),
 .UNSPECIFIED.)
CURVE()
GEOMETRIC_REPRESENTATION_ITEM()
RATIONAL_B_SPLINE_CURVE((1.0000191574532,1.07458139657216,1.05821963517905))
REPRESENTATION_ITEM('')
);
#1294=(
BOUNDED_CURVE()
B_SPLINE_CURVE(2,(#27324,#27325,#27326),.UNSPECIFIED.,.F.,.F.)
B_SPLINE_CURVE_WITH_KNOTS((3,3),(0.039202339545081,0.100434111321637),
 .UNSPECIFIED.)
CURVE()
GEOMETRIC_REPRESENTATION_ITEM()
RATIONAL_B_SPLINE_CURVE((1.05821963517899,1.07458139657208,1.00001915745317))
REPRESENTATION_ITEM('')
);
#1295=(
BOUNDED_CURVE()
B_SPLINE_CURVE(2,(#27344,#27345,#27346),.UNSPECIFIED.,.F.,.F.)
B_SPLINE_CURVE_WITH_KNOTS((3,3),(2.06502885037694E-6,0.0443073288438504),
 .UNSPECIFIED.)
CURVE()
GEOMETRIC_REPRESENTATION_ITEM()
RATIONAL_B_SPLINE_CURVE((1.00000000159591,1.00001712141043,1.00002048940816))
REPRESENTATION_ITEM('')
);
#1296=(
BOUNDED_CURVE()
B_SPLINE_CURVE(2,(#27350,#27351,#27352),.UNSPECIFIED.,.F.,.F.)
B_SPLINE_CURVE_WITH_KNOTS((3,3),(0.0660091927116714,0.110314456526714),
 .UNSPECIFIED.)
CURVE()
GEOMETRIC_REPRESENTATION_ITEM()
RATIONAL_B_SPLINE_CURVE((1.00002048940854,1.00001712141075,1.00000000159591))
REPRESENTATION_ITEM('')
);
#1297=(
BOUNDED_CURVE()
B_SPLINE_CURVE(2,(#27359,#27360,#27361),.UNSPECIFIED.,.F.,.F.)
B_SPLINE_CURVE_WITH_KNOTS((3,3),(7.86559624227606E-6,0.0612396373727856),
 .UNSPECIFIED.)
CURVE()
GEOMETRIC_REPRESENTATION_ITEM()
RATIONAL_B_SPLINE_CURVE((1.00001915745323,1.07458139657213,1.05821963517903))
REPRESENTATION_ITEM('')
);
#1298=(
BOUNDED_CURVE()
B_SPLINE_CURVE(2,(#27366,#27367,#27368),.UNSPECIFIED.,.F.,.F.)
B_SPLINE_CURVE_WITH_KNOTS((3,3),(0.0392023395450793,0.100434111321634),
 .UNSPECIFIED.)
CURVE()
GEOMETRIC_REPRESENTATION_ITEM()
RATIONAL_B_SPLINE_CURVE((1.0582196351791,1.07458139657223,1.00001915745319))
REPRESENTATION_ITEM('')
);
#1299=(
BOUNDED_CURVE()
B_SPLINE_CURVE(2,(#27386,#27387,#27388),.UNSPECIFIED.,.F.,.F.)
B_SPLINE_CURVE_WITH_KNOTS((3,3),(2.06502885144773E-6,0.044307328843974),
 .UNSPECIFIED.)
CURVE()
GEOMETRIC_REPRESENTATION_ITEM()
RATIONAL_B_SPLINE_CURVE((1.00000000159591,1.00001712140841,1.00002048940574))
REPRESENTATION_ITEM('')
);
#1300=(
BOUNDED_CURVE()
B_SPLINE_CURVE(2,(#27392,#27393,#27394),.UNSPECIFIED.,.F.,.F.)
B_SPLINE_CURVE_WITH_KNOTS((3,3),(0.0660091927116272,0.110314456526716),
 .UNSPECIFIED.)
CURVE()
GEOMETRIC_REPRESENTATION_ITEM()
RATIONAL_B_SPLINE_CURVE((1.00002048940471,1.00001712140755,1.00000000159591))
REPRESENTATION_ITEM('')
);
#1301=(
BOUNDED_CURVE()
B_SPLINE_CURVE(2,(#27401,#27402,#27403),.UNSPECIFIED.,.F.,.F.)
B_SPLINE_CURVE_WITH_KNOTS((3,3),(7.86559623316717E-6,0.0612396373727784),
 .UNSPECIFIED.)
CURVE()
GEOMETRIC_REPRESENTATION_ITEM()
RATIONAL_B_SPLINE_CURVE((1.0000191574532,1.07458139657221,1.05821963517909))
REPRESENTATION_ITEM('')
);
#1302=(
BOUNDED_CURVE()
B_SPLINE_CURVE(2,(#27408,#27409,#27410),.UNSPECIFIED.,.F.,.F.)
B_SPLINE_CURVE_WITH_KNOTS((3,3),(0.0392023395450884,0.100434111321648),
 .UNSPECIFIED.)
CURVE()
GEOMETRIC_REPRESENTATION_ITEM()
RATIONAL_B_SPLINE_CURVE((1.05821963517895,1.07458139657204,1.00001915745322))
REPRESENTATION_ITEM('')
);
#1303=(
BOUNDED_CURVE()
B_SPLINE_CURVE(2,(#27428,#27429,#27430),.UNSPECIFIED.,.F.,.F.)
B_SPLINE_CURVE_WITH_KNOTS((3,3),(2.06502884894631E-6,0.0443073288438279),
 .UNSPECIFIED.)
CURVE()
GEOMETRIC_REPRESENTATION_ITEM()
RATIONAL_B_SPLINE_CURVE((1.00000000159591,1.00001712141452,1.00002048941305))
REPRESENTATION_ITEM('')
);
#1304=(
BOUNDED_CURVE()
B_SPLINE_CURVE(2,(#27434,#27435,#27436),.UNSPECIFIED.,.F.,.F.)
B_SPLINE_CURVE_WITH_KNOTS((3,3),(0.0660091927115484,0.110314456526686),
 .UNSPECIFIED.)
CURVE()
GEOMETRIC_REPRESENTATION_ITEM()
RATIONAL_B_SPLINE_CURVE((1.00002048939942,1.00001712140313,1.00000000159591))
REPRESENTATION_ITEM('')
);
#1305=(
BOUNDED_CURVE()
B_SPLINE_CURVE(2,(#27443,#27444,#27445),.UNSPECIFIED.,.F.,.F.)
B_SPLINE_CURVE_WITH_KNOTS((3,3),(7.86559624503439E-6,0.0612396373727955),
 .UNSPECIFIED.)
CURVE()
GEOMETRIC_REPRESENTATION_ITEM()
RATIONAL_B_SPLINE_CURVE((1.00001915745323,1.07458139657222,1.0582196351791))
REPRESENTATION_ITEM('')
);
#1306=(
BOUNDED_CURVE()
B_SPLINE_CURVE(2,(#27450,#27451,#27452),.UNSPECIFIED.,.F.,.F.)
B_SPLINE_CURVE_WITH_KNOTS((3,3),(0.0392023395450828,0.100434111321649),
 .UNSPECIFIED.)
CURVE()
GEOMETRIC_REPRESENTATION_ITEM()
RATIONAL_B_SPLINE_CURVE((1.05821963517927,1.07458139657245,1.00001915745322))
REPRESENTATION_ITEM('')
);
#1307=(
BOUNDED_CURVE()
B_SPLINE_CURVE(2,(#27470,#27471,#27472),.UNSPECIFIED.,.F.,.F.)
B_SPLINE_CURVE_WITH_KNOTS((3,3),(2.06502884806617E-6,0.044307328843884),
 .UNSPECIFIED.)
CURVE()
GEOMETRIC_REPRESENTATION_ITEM()
RATIONAL_B_SPLINE_CURVE((1.00000000159591,1.00001712140915,1.00002048940663))
REPRESENTATION_ITEM('')
);
#1308=(
BOUNDED_CURVE()
B_SPLINE_CURVE(2,(#27476,#27477,#27478),.UNSPECIFIED.,.F.,.F.)
B_SPLINE_CURVE_WITH_KNOTS((3,3),(0.0660091927117217,0.110314456526714),
 .UNSPECIFIED.)
CURVE()
GEOMETRIC_REPRESENTATION_ITEM()
RATIONAL_B_SPLINE_CURVE((1.00002048940948,1.00001712141153,1.00000000159591))
REPRESENTATION_ITEM('')
);
#1309=(
BOUNDED_CURVE()
B_SPLINE_CURVE(2,(#27485,#27486,#27487),.UNSPECIFIED.,.F.,.F.)
B_SPLINE_CURVE_WITH_KNOTS((3,3),(7.86559623218909E-6,0.0612396373727783),
 .UNSPECIFIED.)
CURVE()
GEOMETRIC_REPRESENTATION_ITEM()
RATIONAL_B_SPLINE_CURVE((1.0000191574532,1.07458139657225,1.05821963517912))
REPRESENTATION_ITEM('')
);
#1310=(
BOUNDED_CURVE()
B_SPLINE_CURVE(2,(#27492,#27493,#27494),.UNSPECIFIED.,.F.,.F.)
B_SPLINE_CURVE_WITH_KNOTS((3,3),(0.0392023395450802,0.100434111321634),
 .UNSPECIFIED.)
CURVE()
GEOMETRIC_REPRESENTATION_ITEM()
RATIONAL_B_SPLINE_CURVE((1.05821963517902,1.07458139657212,1.0000191574532))
REPRESENTATION_ITEM('')
);
#1311=(
BOUNDED_CURVE()
B_SPLINE_CURVE(2,(#27510,#27511,#27512),.UNSPECIFIED.,.F.,.F.)
B_SPLINE_CURVE_WITH_KNOTS((3,3),(0.0142112171256889,0.110567648737577),
 .UNSPECIFIED.)
CURVE()
GEOMETRIC_REPRESENTATION_ITEM()
RATIONAL_B_SPLINE_CURVE((1.00000961767866,1.00003742651004,1.00000019074342))
REPRESENTATION_ITEM('')
);
#1312=(
BOUNDED_CURVE()
B_SPLINE_CURVE(2,(#27529,#27530,#27531),.UNSPECIFIED.,.F.,.F.)
B_SPLINE_CURVE_WITH_KNOTS((3,3),(0.000246247416171589,0.0445514940288941),
 .UNSPECIFIED.)
CURVE()
GEOMETRIC_REPRESENTATION_ITEM()
RATIONAL_B_SPLINE_CURVE((1.00000019074345,1.00001731196734,1.00002068137086))
REPRESENTATION_ITEM('')
);
#1313=(
BOUNDED_CURVE()
B_SPLINE_CURVE(2,(#27541,#27542,#27543),.UNSPECIFIED.,.F.,.F.)
B_SPLINE_CURVE_WITH_KNOTS((3,3),(0.000246247416178378,0.0966026790274705),
 .UNSPECIFIED.)
CURVE()
GEOMETRIC_REPRESENTATION_ITEM()
RATIONAL_B_SPLINE_CURVE((1.00000019074344,1.00003742651365,1.00000961767959))
REPRESENTATION_ITEM('')
);
#1314=(
BOUNDED_CURVE()
B_SPLINE_CURVE(2,(#27549,#27550,#27551),.UNSPECIFIED.,.F.,.F.)
B_SPLINE_CURVE_WITH_KNOTS((3,3),(0.0142112171255851,0.11056764873757),
 .UNSPECIFIED.)
CURVE()
GEOMETRIC_REPRESENTATION_ITEM()
RATIONAL_B_SPLINE_CURVE((1.00000961768111,1.00003742651954,1.00000019074347))
REPRESENTATION_ITEM('')
);
#1315=(
BOUNDED_CURVE()
B_SPLINE_CURVE(2,(#27624,#27625,#27626),.UNSPECIFIED.,.F.,.F.)
B_SPLINE_CURVE_WITH_KNOTS((3,3),(0.000496318296887013,0.0448015472108987),
 .UNSPECIFIED.)
CURVE()
GEOMETRIC_REPRESENTATION_ITEM()
RATIONAL_B_SPLINE_CURVE((1.00000038535058,1.00001750801892,1.00002087886772))
REPRESENTATION_ITEM('')
);
#1316=(
BOUNDED_CURVE()
B_SPLINE_CURVE(2,(#27632,#27633,#27634),.UNSPECIFIED.,.F.,.F.)
B_SPLINE_CURVE_WITH_KNOTS((3,3),(0.0665217606070769,0.110826989520968),
 .UNSPECIFIED.)
CURVE()
GEOMETRIC_REPRESENTATION_ITEM()
RATIONAL_B_SPLINE_CURVE((1.0000208788742,1.00001750802436,1.0000003853507))
REPRESENTATION_ITEM('')
);
#1317=(
BOUNDED_CURVE()
B_SPLINE_CURVE(2,(#27648,#27649,#27650),.UNSPECIFIED.,.F.,.F.)
B_SPLINE_CURVE_WITH_KNOTS((3,3),(7.86559624534712E-6,0.061239637372799),
 .UNSPECIFIED.)
CURVE()
GEOMETRIC_REPRESENTATION_ITEM()
RATIONAL_B_SPLINE_CURVE((1.00001915745323,1.07458139657233,1.05821963517918))
REPRESENTATION_ITEM('')
);
#1318=(
BOUNDED_CURVE()
B_SPLINE_CURVE(2,(#27658,#27659,#27660),.UNSPECIFIED.,.F.,.F.)
B_SPLINE_CURVE_WITH_KNOTS((3,3),(2.06502884745806E-6,0.0443073288438634),
 .UNSPECIFIED.)
CURVE()
GEOMETRIC_REPRESENTATION_ITEM()
RATIONAL_B_SPLINE_CURVE((1.00000000159591,1.00001712141092,1.00002048940875))
REPRESENTATION_ITEM('')
);
#1319=(
BOUNDED_CURVE()
B_SPLINE_CURVE(2,(#27662,#27663,#27664),.UNSPECIFIED.,.F.,.F.)
B_SPLINE_CURVE_WITH_KNOTS((3,3),(0.0392023395450795,0.100434111321635),
 .UNSPECIFIED.)
CURVE()
GEOMETRIC_REPRESENTATION_ITEM()
RATIONAL_B_SPLINE_CURVE((1.05821963517901,1.07458139657211,1.00001915745319))
REPRESENTATION_ITEM('')
);
#1320=(
BOUNDED_CURVE()
B_SPLINE_CURVE(2,(#27670,#27671,#27672),.UNSPECIFIED.,.F.,.F.)
B_SPLINE_CURVE_WITH_KNOTS((3,3),(0.0660091927116517,0.110314456526715),
 .UNSPECIFIED.)
CURVE()
GEOMETRIC_REPRESENTATION_ITEM()
RATIONAL_B_SPLINE_CURVE((1.00002048940891,1.00001712141106,1.00000000159591))
REPRESENTATION_ITEM('')
);
#1321=(
BOUNDED_CURVE()
B_SPLINE_CURVE(2,(#27690,#27691,#27692),.UNSPECIFIED.,.F.,.F.)
B_SPLINE_CURVE_WITH_KNOTS((3,3),(7.86559623604086E-6,0.0612396373727819),
 .UNSPECIFIED.)
CURVE()
GEOMETRIC_REPRESENTATION_ITEM()
RATIONAL_B_SPLINE_CURVE((1.00001915745321,1.07458139657227,1.05821963517914))
REPRESENTATION_ITEM('')
);
#1322=(
BOUNDED_CURVE()
B_SPLINE_CURVE(2,(#27700,#27701,#27702),.UNSPECIFIED.,.F.,.F.)
B_SPLINE_CURVE_WITH_KNOTS((3,3),(2.06502884700055E-6,0.0443073288438819),
 .UNSPECIFIED.)
CURVE()
GEOMETRIC_REPRESENTATION_ITEM()
RATIONAL_B_SPLINE_CURVE((1.00000000159591,1.00001712140918,1.00002048940666))
REPRESENTATION_ITEM('')
);
#1323=(
BOUNDED_CURVE()
B_SPLINE_CURVE(2,(#27704,#27705,#27706),.UNSPECIFIED.,.F.,.F.)
B_SPLINE_CURVE_WITH_KNOTS((3,3),(0.0392023395450774,0.100434111321637),
 .UNSPECIFIED.)
CURVE()
GEOMETRIC_REPRESENTATION_ITEM()
RATIONAL_B_SPLINE_CURVE((1.05821963517918,1.07458139657232,1.00001915745317))
REPRESENTATION_ITEM('')
);
#1324=(
BOUNDED_CURVE()
B_SPLINE_CURVE(2,(#27712,#27713,#27714),.UNSPECIFIED.,.F.,.F.)
B_SPLINE_CURVE_WITH_KNOTS((3,3),(0.0660091927116316,0.110314456526682),
 .UNSPECIFIED.)
CURVE()
GEOMETRIC_REPRESENTATION_ITEM()
RATIONAL_B_SPLINE_CURVE((1.00002048940402,1.00001712140697,1.00000000159591))
REPRESENTATION_ITEM('')
);
#1325=(
BOUNDED_CURVE()
B_SPLINE_CURVE(2,(#27732,#27733,#27734),.UNSPECIFIED.,.F.,.F.)
B_SPLINE_CURVE_WITH_KNOTS((3,3),(7.86559623940256E-6,0.0612396373727946),
 .UNSPECIFIED.)
CURVE()
GEOMETRIC_REPRESENTATION_ITEM()
RATIONAL_B_SPLINE_CURVE((1.00001915745322,1.0745813965724,1.05821963517923))
REPRESENTATION_ITEM('')
);
#1326=(
BOUNDED_CURVE()
B_SPLINE_CURVE(2,(#27742,#27743,#27744),.UNSPECIFIED.,.F.,.F.)
B_SPLINE_CURVE_WITH_KNOTS((3,3),(2.06502884915366E-6,0.0443073288438936),
 .UNSPECIFIED.)
CURVE()
GEOMETRIC_REPRESENTATION_ITEM()
RATIONAL_B_SPLINE_CURVE((1.00000000159591,1.00001712141024,1.00002048940794))
REPRESENTATION_ITEM('')
);
#1327=(
BOUNDED_CURVE()
B_SPLINE_CURVE(2,(#27746,#27747,#27748),.UNSPECIFIED.,.F.,.F.)
B_SPLINE_CURVE_WITH_KNOTS((3,3),(0.0392023395450764,0.100434111321633),
 .UNSPECIFIED.)
CURVE()
GEOMETRIC_REPRESENTATION_ITEM()
RATIONAL_B_SPLINE_CURVE((1.05821963517915,1.07458139657229,1.00001915745319))
REPRESENTATION_ITEM('')
);
#1328=(
BOUNDED_CURVE()
B_SPLINE_CURVE(2,(#27754,#27755,#27756),.UNSPECIFIED.,.F.,.F.)
B_SPLINE_CURVE_WITH_KNOTS((3,3),(0.0660091927116924,0.110314456526717),
 .UNSPECIFIED.)
CURVE()
GEOMETRIC_REPRESENTATION_ITEM()
RATIONAL_B_SPLINE_CURVE((1.00002048940367,1.00001712140668,1.00000000159591))
REPRESENTATION_ITEM('')
);
#1329=(
BOUNDED_CURVE()
B_SPLINE_CURVE(2,(#27774,#27775,#27776),.UNSPECIFIED.,.F.,.F.)
B_SPLINE_CURVE_WITH_KNOTS((3,3),(7.86559623680102E-6,0.0612396373727785),
 .UNSPECIFIED.)
CURVE()
GEOMETRIC_REPRESENTATION_ITEM()
RATIONAL_B_SPLINE_CURVE((1.00001915745321,1.074581396572,1.05821963517893))
REPRESENTATION_ITEM('')
);
#1330=(
BOUNDED_CURVE()
B_SPLINE_CURVE(2,(#27784,#27785,#27786),.UNSPECIFIED.,.F.,.F.)
B_SPLINE_CURVE_WITH_KNOTS((3,3),(2.06502885214286E-6,0.0443073288438507),
 .UNSPECIFIED.)
CURVE()
GEOMETRIC_REPRESENTATION_ITEM()
RATIONAL_B_SPLINE_CURVE((1.00000000159591,1.00001712141213,1.0000204894102))
REPRESENTATION_ITEM('')
);
#1331=(
BOUNDED_CURVE()
B_SPLINE_CURVE(2,(#27788,#27789,#27790),.UNSPECIFIED.,.F.,.F.)
B_SPLINE_CURVE_WITH_KNOTS((3,3),(0.0392023395450757,0.100434111321633),
 .UNSPECIFIED.)
CURVE()
GEOMETRIC_REPRESENTATION_ITEM()
RATIONAL_B_SPLINE_CURVE((1.05821963517913,1.07458139657228,1.0000191574532))
REPRESENTATION_ITEM('')
);
#1332=(
BOUNDED_CURVE()
B_SPLINE_CURVE(2,(#27796,#27797,#27798),.UNSPECIFIED.,.F.,.F.)
B_SPLINE_CURVE_WITH_KNOTS((3,3),(0.0660091927116415,0.110314456526713),
 .UNSPECIFIED.)
CURVE()
GEOMETRIC_REPRESENTATION_ITEM()
RATIONAL_B_SPLINE_CURVE((1.00002048940584,1.00001712140849,1.00000000159591))
REPRESENTATION_ITEM('')
);
#1333=(
BOUNDED_CURVE()
B_SPLINE_CURVE(2,(#27816,#27817,#27818),.UNSPECIFIED.,.F.,.F.)
B_SPLINE_CURVE_WITH_KNOTS((3,3),(7.86559624497379E-6,0.0612396373727874),
 .UNSPECIFIED.)
CURVE()
GEOMETRIC_REPRESENTATION_ITEM()
RATIONAL_B_SPLINE_CURVE((1.00001915745323,1.07458139657225,1.05821963517912))
REPRESENTATION_ITEM('')
);
#1334=(
BOUNDED_CURVE()
B_SPLINE_CURVE(2,(#27826,#27827,#27828),.UNSPECIFIED.,.F.,.F.)
B_SPLINE_CURVE_WITH_KNOTS((3,3),(2.06502884959385E-6,0.0443073288439219),
 .UNSPECIFIED.)
CURVE()
GEOMETRIC_REPRESENTATION_ITEM()
RATIONAL_B_SPLINE_CURVE((1.00000000159591,1.00001712140764,1.00002048940482))
REPRESENTATION_ITEM('')
);
#1335=(
BOUNDED_CURVE()
B_SPLINE_CURVE(2,(#27830,#27831,#27832),.UNSPECIFIED.,.F.,.F.)
B_SPLINE_CURVE_WITH_KNOTS((3,3),(0.0392023395450757,0.100434111321633),
 .UNSPECIFIED.)
CURVE()
GEOMETRIC_REPRESENTATION_ITEM()
RATIONAL_B_SPLINE_CURVE((1.05821963517915,1.0745813965723,1.00001915745321))
REPRESENTATION_ITEM('')
);
#1336=(
BOUNDED_CURVE()
B_SPLINE_CURVE(2,(#27838,#27839,#27840),.UNSPECIFIED.,.F.,.F.)
B_SPLINE_CURVE_WITH_KNOTS((3,3),(0.0660091927117066,0.110314456526683),
 .UNSPECIFIED.)
CURVE()
GEOMETRIC_REPRESENTATION_ITEM()
RATIONAL_B_SPLINE_CURVE((1.00002048940495,1.00001712140775,1.00000000159591))
REPRESENTATION_ITEM('')
);
#1337=(
BOUNDED_CURVE()
B_SPLINE_CURVE(2,(#27858,#27859,#27860),.UNSPECIFIED.,.F.,.F.)
B_SPLINE_CURVE_WITH_KNOTS((3,3),(7.86559625117044E-6,0.0612396373728031),
 .UNSPECIFIED.)
CURVE()
GEOMETRIC_REPRESENTATION_ITEM()
RATIONAL_B_SPLINE_CURVE((1.00001915745325,1.07458139657221,1.05821963517909))
REPRESENTATION_ITEM('')
);
#1338=(
BOUNDED_CURVE()
B_SPLINE_CURVE(2,(#27868,#27869,#27870),.UNSPECIFIED.,.F.,.F.)
B_SPLINE_CURVE_WITH_KNOTS((3,3),(2.06502885431328E-6,0.0443073288438909),
 .UNSPECIFIED.)
CURVE()
GEOMETRIC_REPRESENTATION_ITEM()
RATIONAL_B_SPLINE_CURVE((1.00000000159591,1.00001712140729,1.0000204894044))
REPRESENTATION_ITEM('')
);
#1339=(
BOUNDED_CURVE()
B_SPLINE_CURVE(2,(#27872,#27873,#27874),.UNSPECIFIED.,.F.,.F.)
B_SPLINE_CURVE_WITH_KNOTS((3,3),(0.0392023395450745,0.100434111321634),
 .UNSPECIFIED.)
CURVE()
GEOMETRIC_REPRESENTATION_ITEM()
RATIONAL_B_SPLINE_CURVE((1.05821963517924,1.07458139657242,1.00001915745323))
REPRESENTATION_ITEM('')
);
#1340=(
BOUNDED_CURVE()
B_SPLINE_CURVE(2,(#27880,#27881,#27882),.UNSPECIFIED.,.F.,.F.)
B_SPLINE_CURVE_WITH_KNOTS((3,3),(0.0660091927116867,0.110314456526718),
 .UNSPECIFIED.)
CURVE()
GEOMETRIC_REPRESENTATION_ITEM()
RATIONAL_B_SPLINE_CURVE((1.00002048940563,1.00001712140832,1.00000000159591))
REPRESENTATION_ITEM('')
);
#1341=(
BOUNDED_CURVE()
B_SPLINE_CURVE(2,(#27900,#27901,#27902),.UNSPECIFIED.,.F.,.F.)
B_SPLINE_CURVE_WITH_KNOTS((3,3),(7.86559624197589E-6,0.0612396373727868),
 .UNSPECIFIED.)
CURVE()
GEOMETRIC_REPRESENTATION_ITEM()
RATIONAL_B_SPLINE_CURVE((1.00001915745323,1.07458139657218,1.05821963517906))
REPRESENTATION_ITEM('')
);
#1342=(
BOUNDED_CURVE()
B_SPLINE_CURVE(2,(#27910,#27911,#27912),.UNSPECIFIED.,.F.,.F.)
B_SPLINE_CURVE_WITH_KNOTS((3,3),(2.06502884662093E-6,0.0443073288437533),
 .UNSPECIFIED.)
CURVE()
GEOMETRIC_REPRESENTATION_ITEM()
RATIONAL_B_SPLINE_CURVE((1.00000000159591,1.0000171214157,1.00002048941447))
REPRESENTATION_ITEM('')
);
#1343=(
BOUNDED_CURVE()
B_SPLINE_CURVE(2,(#27914,#27915,#27916),.UNSPECIFIED.,.F.,.F.)
B_SPLINE_CURVE_WITH_KNOTS((3,3),(0.0392023395450786,0.100434111321633),
 .UNSPECIFIED.)
CURVE()
GEOMETRIC_REPRESENTATION_ITEM()
RATIONAL_B_SPLINE_CURVE((1.05821963517905,1.07458139657217,1.00001915745321))
REPRESENTATION_ITEM('')
);
#1344=(
BOUNDED_CURVE()
B_SPLINE_CURVE(2,(#27922,#27923,#27924),.UNSPECIFIED.,.F.,.F.)
B_SPLINE_CURVE_WITH_KNOTS((3,3),(0.0660091927117032,0.110314456526714),
 .UNSPECIFIED.)
CURVE()
GEOMETRIC_REPRESENTATION_ITEM()
RATIONAL_B_SPLINE_CURVE((1.0000204894113,1.00001712141305,1.00000000159591))
REPRESENTATION_ITEM('')
);
#1345=(
BOUNDED_CURVE()
B_SPLINE_CURVE(2,(#27942,#27943,#27944),.UNSPECIFIED.,.F.,.F.)
B_SPLINE_CURVE_WITH_KNOTS((3,3),(7.86559625570308E-6,0.0612396373727984),
 .UNSPECIFIED.)
CURVE()
GEOMETRIC_REPRESENTATION_ITEM()
RATIONAL_B_SPLINE_CURVE((1.00001915745326,1.07458139657228,1.05821963517913))
REPRESENTATION_ITEM('')
);
#1346=(
BOUNDED_CURVE()
B_SPLINE_CURVE(2,(#27952,#27953,#27954),.UNSPECIFIED.,.F.,.F.)
B_SPLINE_CURVE_WITH_KNOTS((3,3),(2.06502885013862E-6,0.0443073288438289),
 .UNSPECIFIED.)
CURVE()
GEOMETRIC_REPRESENTATION_ITEM()
RATIONAL_B_SPLINE_CURVE((1.00000000159591,1.00001712141,1.00002048940764))
REPRESENTATION_ITEM('')
);
#1347=(
BOUNDED_CURVE()
B_SPLINE_CURVE(2,(#27956,#27957,#27958),.UNSPECIFIED.,.F.,.F.)
B_SPLINE_CURVE_WITH_KNOTS((3,3),(0.0392023395450752,0.100434111321631),
 .UNSPECIFIED.)
CURVE()
GEOMETRIC_REPRESENTATION_ITEM()
RATIONAL_B_SPLINE_CURVE((1.05821963517917,1.07458139657232,1.00001915745323))
REPRESENTATION_ITEM('')
);
#1348=(
BOUNDED_CURVE()
B_SPLINE_CURVE(2,(#27964,#27965,#27966),.UNSPECIFIED.,.F.,.F.)
B_SPLINE_CURVE_WITH_KNOTS((3,3),(0.0660091927116231,0.110314456526669),
 .UNSPECIFIED.)
CURVE()
GEOMETRIC_REPRESENTATION_ITEM()
RATIONAL_B_SPLINE_CURVE((1.00002048940694,1.00001712140941,1.00000000159591))
REPRESENTATION_ITEM('')
);
#1349=(
BOUNDED_CURVE()
B_SPLINE_CURVE(2,(#27983,#27984,#27985),.UNSPECIFIED.,.F.,.F.)
B_SPLINE_CURVE_WITH_KNOTS((3,3),(0.0392023395450754,0.100434111321632),
 .UNSPECIFIED.)
CURVE()
GEOMETRIC_REPRESENTATION_ITEM()
RATIONAL_B_SPLINE_CURVE((1.05821963517916,1.07458139657231,1.00001915745321))
REPRESENTATION_ITEM('')
);
#1350=(
BOUNDED_CURVE()
B_SPLINE_CURVE(2,(#27994,#27995,#27996),.UNSPECIFIED.,.F.,.F.)
B_SPLINE_CURVE_WITH_KNOTS((3,3),(7.86559624287504E-6,0.0612396373728),
 .UNSPECIFIED.)
CURVE()
GEOMETRIC_REPRESENTATION_ITEM()
RATIONAL_B_SPLINE_CURVE((1.00001915745323,1.07458139657225,1.05821963517912))
REPRESENTATION_ITEM('')
);
#1443=FACE_BOUND('',#3408,.T.);
#1444=FACE_BOUND('',#3855,.T.);
#1445=FACE_BOUND('',#3859,.T.);
#1446=FACE_BOUND('',#3860,.T.);
#1447=FACE_BOUND('',#3861,.T.);
#1448=FACE_BOUND('',#3862,.T.);
#1449=FACE_BOUND('',#3863,.T.);
#1450=FACE_BOUND('',#3864,.T.);
#1451=FACE_BOUND('',#3989,.T.);
#1452=FACE_BOUND('',#3990,.T.);
#1453=FACE_BOUND('',#3991,.T.);
#1454=FACE_BOUND('',#3992,.T.);
#1455=FACE_BOUND('',#3993,.T.);
#1456=FACE_BOUND('',#3994,.T.);
#1457=FACE_BOUND('',#3995,.T.);
#1458=FACE_BOUND('',#3996,.T.);
#1459=FACE_BOUND('',#3997,.T.);
#1460=FACE_BOUND('',#3998,.T.);
#1461=FACE_BOUND('',#3999,.T.);
#1501=CIRCLE('',#17326,53.5);
#1502=CIRCLE('',#17327,53.5);
#1503=CIRCLE('',#17329,53.);
#1504=CIRCLE('',#17332,53.5);
#1505=CIRCLE('',#17333,53.5);
#1506=CIRCLE('',#17335,53.);
#1507=CIRCLE('',#17338,0.700000000000003);
#1508=CIRCLE('',#17339,0.700000000000003);
#1509=CIRCLE('',#17342,0.700000000000003);
#1510=CIRCLE('',#17343,1.2);
#1511=CIRCLE('',#17345,0.700000000000003);
#1512=CIRCLE('',#17348,0.700000000000003);
#1513=CIRCLE('',#17349,0.700000000000003);
#1514=CIRCLE('',#17351,1.2);
#1515=CIRCLE('',#17354,0.700000000000003);
#1516=CIRCLE('',#17355,1.2);
#1517=CIRCLE('',#17357,0.700000000000003);
#1518=CIRCLE('',#17362,0.700000000000003);
#1519=CIRCLE('',#17363,0.700000000000003);
#1520=CIRCLE('',#17365,53.5);
#1521=CIRCLE('',#17366,53.);
#1522=CIRCLE('',#17369,53.5);
#1523=CIRCLE('',#17370,53.5);
#1524=CIRCLE('',#17372,53.);
#1525=CIRCLE('',#17375,53.5);
#1526=CIRCLE('',#17376,53.);
#1527=CIRCLE('',#17378,53.5);
#1528=CIRCLE('',#17382,53.5);
#1529=CIRCLE('',#17383,53.);
#1530=CIRCLE('',#17385,53.5);
#1531=CIRCLE('',#17389,53.5);
#1532=CIRCLE('',#17390,53.);
#1533=CIRCLE('',#17392,53.5);
#1534=CIRCLE('',#17396,53.5);
#1535=CIRCLE('',#17397,53.);
#1536=CIRCLE('',#17399,53.5);
#1537=CIRCLE('',#17403,53.5);
#1538=CIRCLE('',#17404,53.);
#1539=CIRCLE('',#17406,53.5);
#1540=CIRCLE('',#17410,53.5);
#1541=CIRCLE('',#17411,53.);
#1542=CIRCLE('',#17413,53.5);
#1543=CIRCLE('',#17417,53.5);
#1544=CIRCLE('',#17418,53.);
#1545=CIRCLE('',#17420,53.5);
#1546=CIRCLE('',#17424,53.5);
#1547=CIRCLE('',#17425,53.);
#1548=CIRCLE('',#17427,53.5);
#1549=CIRCLE('',#17430,0.700000000000003);
#1550=CIRCLE('',#17431,1.2);
#1551=CIRCLE('',#17433,53.);
#1552=CIRCLE('',#17434,53.5);
#1553=CIRCLE('',#17436,53.);
#1554=CIRCLE('',#17437,53.5);
#1555=CIRCLE('',#17439,53.5);
#1556=CIRCLE('',#17440,53.);
#1557=CIRCLE('',#17442,0.700000000000003);
#1558=CIRCLE('',#17443,53.);
#1559=CIRCLE('',#17444,0.700000000000003);
#1560=CIRCLE('',#17445,53.);
#1561=CIRCLE('',#17446,0.700000000000003);
#1562=CIRCLE('',#17447,53.);
#1563=CIRCLE('',#17448,0.700000000000003);
#1564=CIRCLE('',#17449,53.);
#1565=CIRCLE('',#17450,0.700000000000003);
#1566=CIRCLE('',#17451,53.);
#1567=CIRCLE('',#17452,0.700000000000003);
#1568=CIRCLE('',#17453,53.);
#1569=CIRCLE('',#17454,0.700000000000003);
#1570=CIRCLE('',#17455,1.2);
#1571=CIRCLE('',#17456,1.2);
#1572=CIRCLE('',#17457,1.2);
#1573=CIRCLE('',#17458,1.2);
#1574=CIRCLE('',#17459,1.2);
#1575=CIRCLE('',#17460,1.2);
#1576=CIRCLE('',#17461,1.2);
#1577=CIRCLE('',#17462,1.2);
#1578=CIRCLE('',#17463,53.);
#1579=CIRCLE('',#17464,1.2);
#1580=CIRCLE('',#17465,53.);
#1581=CIRCLE('',#17466,1.2);
#1582=CIRCLE('',#17467,53.);
#1583=CIRCLE('',#17468,1.2);
#1584=CIRCLE('',#17469,53.);
#1585=CIRCLE('',#17470,1.2);
#1586=CIRCLE('',#17471,53.);
#1587=CIRCLE('',#17472,1.20000000000001);
#1588=CIRCLE('',#17473,53.);
#1589=CIRCLE('',#17474,1.2);
#1590=CIRCLE('',#17475,53.);
#1591=CIRCLE('',#17476,1.2);
#1592=CIRCLE('',#17477,53.);
#1593=CIRCLE('',#17478,1.2);
#1594=CIRCLE('',#17479,53.);
#1595=CIRCLE('',#17480,1.2);
#1596=CIRCLE('',#17481,0.700000000000003);
#1597=CIRCLE('',#17482,53.);
#1598=CIRCLE('',#17483,0.700000000000003);
#1599=CIRCLE('',#17484,53.);
#1600=CIRCLE('',#17485,1.2);
#1601=CIRCLE('',#17486,53.);
#1602=CIRCLE('',#17487,1.2);
#1603=CIRCLE('',#17488,53.);
#1604=CIRCLE('',#17489,1.2);
#1605=CIRCLE('',#17490,53.);
#1606=CIRCLE('',#17491,1.2);
#1607=CIRCLE('',#17492,53.);
#1608=CIRCLE('',#17493,1.20000000000001);
#1609=CIRCLE('',#17494,53.);
#1610=CIRCLE('',#17495,1.2);
#1611=CIRCLE('',#17496,53.);
#1612=CIRCLE('',#17497,1.2);
#1613=CIRCLE('',#17498,53.);
#1614=CIRCLE('',#17499,1.2);
#1615=CIRCLE('',#17500,53.);
#1616=CIRCLE('',#17501,0.700000000000003);
#1617=CIRCLE('',#17502,53.);
#1618=CIRCLE('',#17503,1.2);
#1619=CIRCLE('',#17504,53.);
#1620=CIRCLE('',#17505,0.700000000000003);
#1621=CIRCLE('',#17506,53.);
#1622=CIRCLE('',#17507,1.2);
#1623=CIRCLE('',#17508,53.);
#1624=CIRCLE('',#17509,1.2);
#1625=CIRCLE('',#17510,53.);
#1626=CIRCLE('',#17511,1.2);
#1627=CIRCLE('',#17512,53.);
#1628=CIRCLE('',#17513,1.2);
#1629=CIRCLE('',#17514,53.);
#1630=CIRCLE('',#17515,1.2);
#1631=CIRCLE('',#17516,53.);
#1632=CIRCLE('',#17517,1.2);
#1633=CIRCLE('',#17518,53.);
#1634=CIRCLE('',#17519,1.2);
#1635=CIRCLE('',#17520,53.);
#1636=CIRCLE('',#17521,0.700000000000003);
#1637=CIRCLE('',#17522,53.);
#1638=CIRCLE('',#17523,1.2);
#1639=CIRCLE('',#17524,53.);
#1640=CIRCLE('',#17525,1.2);
#1641=CIRCLE('',#17526,53.);
#1642=CIRCLE('',#17527,0.700000000000003);
#1643=CIRCLE('',#17528,53.);
#1644=CIRCLE('',#17529,1.2);
#1645=CIRCLE('',#17530,53.);
#1646=CIRCLE('',#17531,1.2);
#1647=CIRCLE('',#17532,53.);
#1648=CIRCLE('',#17533,1.2);
#1649=CIRCLE('',#17534,53.);
#1650=CIRCLE('',#17535,1.2);
#1651=CIRCLE('',#17536,53.);
#1652=CIRCLE('',#17537,1.2);
#1653=CIRCLE('',#17538,53.);
#1654=CIRCLE('',#17539,1.2);
#1655=CIRCLE('',#17540,53.);
#1656=CIRCLE('',#17541,0.700000000000003);
#1657=CIRCLE('',#17542,53.);
#1658=CIRCLE('',#17543,1.2);
#1659=CIRCLE('',#17544,53.);
#1660=CIRCLE('',#17545,1.20000000000001);
#1661=CIRCLE('',#17546,53.);
#1662=CIRCLE('',#17547,1.2);
#1663=CIRCLE('',#17548,53.);
#1664=CIRCLE('',#17549,0.700000000000003);
#1665=CIRCLE('',#17550,53.);
#1666=CIRCLE('',#17551,1.2);
#1667=CIRCLE('',#17552,53.);
#1668=CIRCLE('',#17553,1.2);
#1669=CIRCLE('',#17554,53.);
#1670=CIRCLE('',#17555,1.2);
#1671=CIRCLE('',#17556,53.);
#1672=CIRCLE('',#17557,1.2);
#1673=CIRCLE('',#17558,53.);
#1674=CIRCLE('',#17559,1.2);
#1675=CIRCLE('',#17560,53.);
#1676=CIRCLE('',#17561,0.700000000000003);
#1677=CIRCLE('',#17562,53.);
#1678=CIRCLE('',#17563,1.2);
#1679=CIRCLE('',#17564,53.);
#1680=CIRCLE('',#17565,1.2);
#1681=CIRCLE('',#17566,53.);
#1682=CIRCLE('',#17567,1.2);
#1683=CIRCLE('',#17568,53.);
#1684=CIRCLE('',#17569,1.2);
#1685=CIRCLE('',#17570,53.);
#1686=CIRCLE('',#17571,0.700000000000003);
#1687=CIRCLE('',#17572,53.);
#1688=CIRCLE('',#17573,1.20000000000001);
#1689=CIRCLE('',#17574,53.);
#1690=CIRCLE('',#17575,1.2);
#1691=CIRCLE('',#17576,53.);
#1692=CIRCLE('',#17577,1.2);
#1693=CIRCLE('',#17578,53.);
#1694=CIRCLE('',#17579,1.2);
#1695=CIRCLE('',#17580,53.);
#1696=CIRCLE('',#17581,0.700000000000003);
#1697=CIRCLE('',#17582,53.);
#1698=CIRCLE('',#17583,1.20000000000001);
#1699=CIRCLE('',#17584,53.);
#1700=CIRCLE('',#17585,1.2);
#1701=CIRCLE('',#17586,53.);
#1702=CIRCLE('',#17587,1.2);
#1703=CIRCLE('',#17588,53.);
#1704=CIRCLE('',#17589,1.2);
#1705=CIRCLE('',#17590,53.);
#1706=CIRCLE('',#17591,1.2);
#1707=CIRCLE('',#17592,53.);
#1708=CIRCLE('',#17593,0.700000000000003);
#1709=CIRCLE('',#17594,53.);
#1710=CIRCLE('',#17595,1.2);
#1711=CIRCLE('',#17596,53.);
#1712=CIRCLE('',#17597,1.2);
#1713=CIRCLE('',#17598,53.);
#1714=CIRCLE('',#17599,1.20000000000001);
#1715=CIRCLE('',#17600,53.);
#1716=CIRCLE('',#17601,50.);
#1717=CIRCLE('',#17603,0.700000000000003);
#1718=CIRCLE('',#17607,0.700000000000003);
#1719=CIRCLE('',#17609,0.700000000000003);
#1720=CIRCLE('',#17613,0.700000000000003);
#1721=CIRCLE('',#17615,0.700000000000003);
#1722=CIRCLE('',#17619,0.700000000000003);
#1723=CIRCLE('',#17621,0.700000000000003);
#1724=CIRCLE('',#17624,53.5);
#1725=CIRCLE('',#17625,53.5);
#1726=CIRCLE('',#17630,53.5);
#1727=CIRCLE('',#17632,53.5);
#1728=CIRCLE('',#17636,53.5);
#1729=CIRCLE('',#17638,53.5);
#1730=CIRCLE('',#17642,53.5);
#1731=CIRCLE('',#17644,53.5);
#1732=CIRCLE('',#17648,53.5);
#1733=CIRCLE('',#17650,53.5);
#1734=CIRCLE('',#17654,53.5);
#1735=CIRCLE('',#17656,53.5);
#1736=CIRCLE('',#17660,53.5);
#1737=CIRCLE('',#17662,53.5);
#1738=CIRCLE('',#17665,53.5);
#1739=CIRCLE('',#17667,53.5);
#1740=CIRCLE('',#17669,53.5);
#1741=CIRCLE('',#17671,53.5);
#1742=CIRCLE('',#17673,53.5);
#1743=CIRCLE('',#17675,53.5);
#1744=CIRCLE('',#17678,0.700000000000003);
#1745=CIRCLE('',#17680,0.700000000000003);
#1746=CIRCLE('',#17682,0.700000000000003);
#1747=CIRCLE('',#17684,0.700000000000003);
#1748=CIRCLE('',#17686,0.700000000000003);
#1749=CIRCLE('',#17688,0.700000000000003);
#1750=CIRCLE('',#17690,0.700000000000003);
#1751=CIRCLE('',#17692,0.700000000000003);
#1752=CIRCLE('',#17694,0.700000000000003);
#1753=CIRCLE('',#17696,0.700000000000003);
#1754=CIRCLE('',#17698,0.700000000000003);
#1755=CIRCLE('',#17701,0.700000000000003);
#1756=CIRCLE('',#17703,0.700000000000003);
#1757=CIRCLE('',#17706,53.5);
#1758=CIRCLE('',#17709,0.700000000000003);
#1759=CIRCLE('',#17711,0.700000000000003);
#1760=CIRCLE('',#17715,0.700000000000003);
#1761=CIRCLE('',#17717,0.700000000000003);
#1762=CIRCLE('',#17721,0.700000000000003);
#1763=CIRCLE('',#17723,0.700000000000003);
#1764=CIRCLE('',#17726,53.5);
#1765=CIRCLE('',#17727,53.5);
#1766=CIRCLE('',#17732,53.5);
#1767=CIRCLE('',#17734,53.5);
#1768=CIRCLE('',#17738,53.5);
#1769=CIRCLE('',#17740,53.5);
#1770=CIRCLE('',#17744,53.5);
#1771=CIRCLE('',#17746,53.5);
#1772=CIRCLE('',#17750,53.5);
#1773=CIRCLE('',#17752,53.5);
#1774=CIRCLE('',#17756,53.5);
#1775=CIRCLE('',#17758,53.5);
#1776=CIRCLE('',#17761,53.5);
#1777=CIRCLE('',#17763,53.5);
#1778=CIRCLE('',#17765,53.5);
#1779=CIRCLE('',#17767,53.5);
#1780=CIRCLE('',#17769,53.5);
#1781=CIRCLE('',#17771,53.5);
#1782=CIRCLE('',#17773,53.5);
#1783=CIRCLE('',#17776,0.700000000000003);
#1784=CIRCLE('',#17778,0.700000000000003);
#1785=CIRCLE('',#17780,0.700000000000003);
#1786=CIRCLE('',#17782,0.700000000000003);
#1787=CIRCLE('',#17784,0.700000000000003);
#1788=CIRCLE('',#17786,0.700000000000003);
#1789=CIRCLE('',#17788,0.700000000000003);
#1790=CIRCLE('',#17790,0.700000000000003);
#1791=CIRCLE('',#17792,0.700000000000003);
#1792=CIRCLE('',#17795,0.700000000000003);
#1793=CIRCLE('',#17797,0.700000000000003);
#1794=CIRCLE('',#17801,0.700000000000003);
#1795=CIRCLE('',#17803,0.700000000000003);
#1796=CIRCLE('',#17807,0.700000000000003);
#1797=CIRCLE('',#17809,0.700000000000003);
#1798=CIRCLE('',#17813,0.700000000000003);
#1799=CIRCLE('',#17815,0.700000000000003);
#1800=CIRCLE('',#17819,0.700000000000003);
#1801=CIRCLE('',#17821,0.700000000000003);
#1802=CIRCLE('',#17824,53.5);
#1803=CIRCLE('',#17825,53.5);
#1804=CIRCLE('',#17830,53.5);
#1805=CIRCLE('',#17832,53.5);
#1806=CIRCLE('',#17836,53.5);
#1807=CIRCLE('',#17838,53.5);
#1808=CIRCLE('',#17842,53.5);
#1809=CIRCLE('',#17844,53.5);
#1810=CIRCLE('',#17848,53.5);
#1811=CIRCLE('',#17850,53.5);
#1812=CIRCLE('',#17853,53.5);
#1813=CIRCLE('',#17855,53.5);
#1814=CIRCLE('',#17857,53.5);
#1815=CIRCLE('',#17859,53.5);
#1816=CIRCLE('',#17861,53.5);
#1817=CIRCLE('',#17863,53.5);
#1818=CIRCLE('',#17865,53.5);
#1819=CIRCLE('',#17867,53.5);
#1820=CIRCLE('',#17869,53.5);
#1821=CIRCLE('',#17871,53.5);
#1822=CIRCLE('',#17874,0.700000000000003);
#1823=CIRCLE('',#17876,0.700000000000003);
#1824=CIRCLE('',#17878,0.700000000000003);
#1825=CIRCLE('',#17880,0.700000000000003);
#1826=CIRCLE('',#17882,0.700000000000003);
#1827=CIRCLE('',#17884,0.700000000000003);
#1828=CIRCLE('',#17886,0.700000000000003);
#1829=CIRCLE('',#17889,0.700000000000003);
#1830=CIRCLE('',#17891,0.700000000000003);
#1831=CIRCLE('',#17894,53.5);
#1832=CIRCLE('',#17897,0.700000000000003);
#1833=CIRCLE('',#17899,0.700000000000003);
#1834=CIRCLE('',#17903,0.700000000000003);
#1835=CIRCLE('',#17905,0.700000000000003);
#1836=CIRCLE('',#17909,0.700000000000003);
#1837=CIRCLE('',#17911,0.700000000000003);
#1838=CIRCLE('',#17915,0.700000000000003);
#1839=CIRCLE('',#17917,0.700000000000003);
#1840=CIRCLE('',#17921,0.700000000000003);
#1841=CIRCLE('',#17923,0.700000000000003);
#1842=CIRCLE('',#17926,53.5);
#1843=CIRCLE('',#17927,53.5);
#1844=CIRCLE('',#17932,53.5);
#1845=CIRCLE('',#17934,53.5);
#1846=CIRCLE('',#17938,53.5);
#1847=CIRCLE('',#17940,53.5);
#1848=CIRCLE('',#17944,53.5);
#1849=CIRCLE('',#17946,53.5);
#1850=CIRCLE('',#17949,53.5);
#1851=CIRCLE('',#17951,53.5);
#1852=CIRCLE('',#17953,53.5);
#1853=CIRCLE('',#17955,53.5);
#1854=CIRCLE('',#17957,53.5);
#1855=CIRCLE('',#17959,53.5);
#1856=CIRCLE('',#17961,53.5);
#1857=CIRCLE('',#17963,53.5);
#1858=CIRCLE('',#17965,53.5);
#1859=CIRCLE('',#17967,53.5);
#1860=CIRCLE('',#17969,53.5);
#1861=CIRCLE('',#17972,0.700000000000003);
#1862=CIRCLE('',#17974,0.700000000000003);
#1863=CIRCLE('',#17976,0.700000000000003);
#1864=CIRCLE('',#17978,0.700000000000003);
#1865=CIRCLE('',#17980,0.700000000000003);
#1866=CIRCLE('',#17983,0.700000000000003);
#1867=CIRCLE('',#17985,0.700000000000003);
#1868=CIRCLE('',#17989,0.700000000000003);
#1869=CIRCLE('',#17991,0.700000000000003);
#1870=CIRCLE('',#17995,0.700000000000003);
#1871=CIRCLE('',#17997,0.700000000000003);
#1872=CIRCLE('',#18001,0.700000000000003);
#1873=CIRCLE('',#18003,0.700000000000003);
#1874=CIRCLE('',#18007,0.700000000000003);
#1875=CIRCLE('',#18009,0.700000000000003);
#1876=CIRCLE('',#18013,0.700000000000003);
#1877=CIRCLE('',#18015,0.700000000000003);
#1878=CIRCLE('',#18019,0.700000000000003);
#1879=CIRCLE('',#18021,0.700000000000003);
#1880=CIRCLE('',#18024,53.5);
#1881=CIRCLE('',#18025,53.5);
#1882=CIRCLE('',#18030,53.5);
#1883=CIRCLE('',#18032,53.5);
#1884=CIRCLE('',#18036,53.5);
#1885=CIRCLE('',#18038,53.5);
#1886=CIRCLE('',#18041,53.5);
#1887=CIRCLE('',#18043,53.5);
#1888=CIRCLE('',#18045,53.5);
#1889=CIRCLE('',#18047,53.5);
#1890=CIRCLE('',#18049,53.5);
#1891=CIRCLE('',#18051,53.5);
#1892=CIRCLE('',#18053,53.5);
#1893=CIRCLE('',#18055,53.5);
#1894=CIRCLE('',#18057,53.5);
#1895=CIRCLE('',#18059,53.5);
#1896=CIRCLE('',#18061,53.5);
#1897=CIRCLE('',#18063,53.5);
#1898=CIRCLE('',#18065,53.5);
#1899=CIRCLE('',#18067,53.5);
#1900=CIRCLE('',#18070,0.700000000000003);
#1901=CIRCLE('',#18072,0.700000000000003);
#1902=CIRCLE('',#18074,0.700000000000003);
#1903=CIRCLE('',#18077,0.700000000000003);
#1904=CIRCLE('',#18079,0.700000000000003);
#1905=CIRCLE('',#18083,0.700000000000003);
#1906=CIRCLE('',#18085,0.700000000000003);
#1907=CIRCLE('',#18089,0.700000000000003);
#1908=CIRCLE('',#18091,0.700000000000003);
#1909=CIRCLE('',#18095,0.700000000000003);
#1910=CIRCLE('',#18097,0.700000000000003);
#1911=CIRCLE('',#18101,0.700000000000003);
#1912=CIRCLE('',#18103,0.700000000000003);
#1913=CIRCLE('',#18107,0.700000000000003);
#1914=CIRCLE('',#18109,0.700000000000003);
#1915=CIRCLE('',#18113,0.700000000000003);
#1916=CIRCLE('',#18115,0.700000000000003);
#1917=CIRCLE('',#18119,0.700000000000003);
#1918=CIRCLE('',#18121,0.700000000000003);
#1919=CIRCLE('',#18124,53.5);
#1920=CIRCLE('',#18125,53.5);
#1921=CIRCLE('',#18130,53.5);
#1922=CIRCLE('',#18132,53.5);
#1923=CIRCLE('',#18135,53.5);
#1924=CIRCLE('',#18137,53.5);
#1925=CIRCLE('',#18139,53.5);
#1926=CIRCLE('',#18141,53.5);
#1927=CIRCLE('',#18143,53.5);
#1928=CIRCLE('',#18145,53.5);
#1929=CIRCLE('',#18147,53.5);
#1930=CIRCLE('',#18149,53.5);
#1931=CIRCLE('',#18151,53.5);
#1932=CIRCLE('',#18153,53.5);
#1933=CIRCLE('',#18155,53.5);
#1934=CIRCLE('',#18157,53.5);
#1935=CIRCLE('',#18159,53.5);
#1936=CIRCLE('',#18161,53.5);
#1937=CIRCLE('',#18163,53.5);
#1938=CIRCLE('',#18165,53.5);
#1939=CIRCLE('',#18168,0.700000000000003);
#1940=CIRCLE('',#18171,53.5);
#1941=CIRCLE('',#18173,53.5);
#1942=CIRCLE('',#18177,53.5);
#1943=CIRCLE('',#18179,53.5);
#1944=CIRCLE('',#18183,53.5);
#1945=CIRCLE('',#18185,53.5);
#1946=CIRCLE('',#18189,53.5);
#1947=CIRCLE('',#18191,53.5);
#1948=CIRCLE('',#18195,53.5);
#1949=CIRCLE('',#18197,53.5);
#1950=CIRCLE('',#18201,53.5);
#1951=CIRCLE('',#18203,53.5);
#1952=CIRCLE('',#18207,53.5);
#1953=CIRCLE('',#18209,53.5);
#1954=CIRCLE('',#18213,53.5);
#1955=CIRCLE('',#18215,53.5);
#1956=CIRCLE('',#18219,53.5);
#1957=CIRCLE('',#18221,53.5);
#1958=CIRCLE('',#18224,0.700000000000003);
#1959=CIRCLE('',#18225,0.700000000000003);
#1960=CIRCLE('',#18229,0.700000000000003);
#1961=CIRCLE('',#18231,0.700000000000003);
#1962=CIRCLE('',#18233,0.700000000000003);
#1963=CIRCLE('',#18235,0.700000000000003);
#1964=CIRCLE('',#18237,0.700000000000003);
#1965=CIRCLE('',#18239,0.700000000000003);
#1966=CIRCLE('',#18241,0.700000000000003);
#1967=CIRCLE('',#18243,0.700000000000003);
#1968=CIRCLE('',#18245,0.700000000000003);
#1969=CIRCLE('',#18247,0.700000000000003);
#1970=CIRCLE('',#18249,0.700000000000003);
#1971=CIRCLE('',#18251,0.700000000000003);
#1972=CIRCLE('',#18253,0.700000000000003);
#1973=CIRCLE('',#18255,0.700000000000003);
#1974=CIRCLE('',#18257,0.700000000000003);
#1975=CIRCLE('',#18259,0.700000000000003);
#1976=CIRCLE('',#18261,49.5);
#1977=CIRCLE('',#18263,49.5);
#1978=CIRCLE('',#18266,0.700000000000003);
#1979=CIRCLE('',#18268,0.700000000000003);
#1980=CIRCLE('',#18270,0.700000000000003);
#1981=CIRCLE('',#18272,0.700000000000003);
#1982=CIRCLE('',#18274,0.700000000000003);
#1983=CIRCLE('',#18276,0.700000000000003);
#1984=CIRCLE('',#18278,0.700000000000003);
#1985=CIRCLE('',#18280,0.700000000000003);
#1986=CIRCLE('',#18282,0.700000000000003);
#1987=CIRCLE('',#18284,0.700000000000003);
#1988=CIRCLE('',#18286,0.700000000000003);
#1989=CIRCLE('',#18288,0.700000000000003);
#1990=CIRCLE('',#18290,0.700000000000003);
#1991=CIRCLE('',#18292,0.700000000000003);
#1992=CIRCLE('',#18294,0.700000000000003);
#1993=CIRCLE('',#18296,0.700000000000003);
#1994=CIRCLE('',#18298,0.700000000000003);
#1995=CIRCLE('',#18301,0.700000000000003);
#1996=CIRCLE('',#18304,53.5);
#1997=CIRCLE('',#18307,0.700000000000003);
#1998=CIRCLE('',#18310,53.5);
#1999=CIRCLE('',#18313,0.700000000000003);
#2000=CIRCLE('',#18316,53.5);
#2001=CIRCLE('',#18319,0.700000000000003);
#2002=CIRCLE('',#18322,53.5);
#2003=CIRCLE('',#18325,0.700000000000003);
#2004=CIRCLE('',#18328,53.5);
#2005=CIRCLE('',#18331,0.700000000000003);
#2006=CIRCLE('',#18334,53.5);
#2007=CIRCLE('',#18337,53.0535533905933);
#2008=CIRCLE('',#18338,52.2);
#2009=CIRCLE('',#18340,51.1);
#2010=CIRCLE('',#18342,53.5);
#2011=CIRCLE('',#18343,53.5);
#2012=CIRCLE('',#18344,53.5);
#2013=CIRCLE('',#18345,53.5);
#2014=CIRCLE('',#18346,53.5);
#2015=CIRCLE('',#18347,53.5);
#2016=CIRCLE('',#18348,53.5);
#2017=CIRCLE('',#18349,53.5);
#2018=CIRCLE('',#18350,53.5);
#2019=CIRCLE('',#18351,53.5);
#2020=CIRCLE('',#18352,53.5);
#2021=CIRCLE('',#18353,53.5);
#2022=CIRCLE('',#18354,53.5);
#2023=CIRCLE('',#18355,53.5);
#2024=CIRCLE('',#18356,53.5);
#2025=CIRCLE('',#18357,53.5);
#2026=CIRCLE('',#18358,53.5);
#2027=CIRCLE('',#18359,53.5);
#2028=CIRCLE('',#18360,53.5);
#2029=CIRCLE('',#18361,53.5);
#2030=CIRCLE('',#18362,53.5);
#2031=CIRCLE('',#18363,53.5);
#2032=CIRCLE('',#18364,53.5);
#2033=CIRCLE('',#18365,53.5);
#2034=CIRCLE('',#18366,53.5);
#2035=CIRCLE('',#18367,53.5);
#2036=CIRCLE('',#18368,53.5);
#2037=CIRCLE('',#18369,53.5);
#2038=CIRCLE('',#18370,53.5);
#2039=CIRCLE('',#18371,53.5);
#2040=CIRCLE('',#18372,53.5);
#2041=CIRCLE('',#18373,53.5);
#2042=CIRCLE('',#18374,53.5);
#2043=CIRCLE('',#18375,53.5);
#2044=CIRCLE('',#18376,53.5);
#2045=CIRCLE('',#18377,53.5);
#2046=CIRCLE('',#18378,53.5);
#2047=CIRCLE('',#18379,53.5);
#2048=CIRCLE('',#18380,53.5);
#2049=CIRCLE('',#18381,53.5);
#2050=CIRCLE('',#18382,53.5);
#2051=CIRCLE('',#18383,53.5);
#2052=CIRCLE('',#18384,53.5);
#2053=CIRCLE('',#18385,53.5);
#2054=CIRCLE('',#18386,53.5);
#2055=CIRCLE('',#18387,53.5);
#2056=CIRCLE('',#18388,53.5);
#2057=CIRCLE('',#18389,53.5);
#2058=CIRCLE('',#18390,53.5);
#2059=CIRCLE('',#18391,53.5);
#2060=CIRCLE('',#18392,53.5);
#2061=CIRCLE('',#18393,53.5);
#2062=CIRCLE('',#18394,53.5);
#2063=CIRCLE('',#18395,53.5);
#2064=CIRCLE('',#18396,53.5);
#2065=CIRCLE('',#18397,53.5);
#2066=CIRCLE('',#18398,53.5);
#2067=CIRCLE('',#18399,53.5);
#2068=CIRCLE('',#18400,53.5);
#2069=CIRCLE('',#18401,53.5);
#2070=CIRCLE('',#18402,53.5);
#2071=CIRCLE('',#18403,53.5);
#2072=CIRCLE('',#18404,53.5);
#2073=CIRCLE('',#18405,53.5);
#2074=CIRCLE('',#18406,53.5);
#2075=CIRCLE('',#18407,53.5);
#2076=CIRCLE('',#18408,53.5);
#2077=CIRCLE('',#18409,53.5);
#2078=CIRCLE('',#18410,53.5);
#2079=CIRCLE('',#18411,53.5);
#2080=CIRCLE('',#18412,53.5);
#2081=CIRCLE('',#18413,53.5);
#2082=CIRCLE('',#18414,53.5);
#2083=CIRCLE('',#18415,53.5);
#2084=CIRCLE('',#18416,53.5);
#2085=CIRCLE('',#18417,53.5);
#2086=CIRCLE('',#18418,53.5);
#2087=CIRCLE('',#18419,53.5);
#2088=CIRCLE('',#18420,53.5);
#2089=CIRCLE('',#18421,53.5);
#2090=CIRCLE('',#18422,53.5);
#2091=CIRCLE('',#18423,53.5);
#2092=CIRCLE('',#18424,53.5);
#2093=CIRCLE('',#18425,53.5);
#2094=CIRCLE('',#18426,53.5);
#2095=CIRCLE('',#18427,53.5);
#2096=CIRCLE('',#18428,53.5);
#2097=CIRCLE('',#18429,53.5);
#2098=CIRCLE('',#18430,53.5);
#2099=CIRCLE('',#18431,53.5);
#2100=CIRCLE('',#18432,53.5);
#2101=CIRCLE('',#18433,53.5);
#2102=CIRCLE('',#18434,53.5);
#2103=CIRCLE('',#18435,53.5);
#2104=CIRCLE('',#18436,53.5);
#2105=CIRCLE('',#18437,53.5);
#2106=CIRCLE('',#18438,53.5);
#2107=CIRCLE('',#18439,53.5);
#2108=CIRCLE('',#18440,53.5);
#2109=CIRCLE('',#18441,53.5);
#2110=CIRCLE('',#18442,53.5);
#2111=CIRCLE('',#18444,12.9);
#2112=CIRCLE('',#18445,12.5);
#2113=CIRCLE('',#18447,50.5);
#2114=CIRCLE('',#18448,12.9);
#2115=CIRCLE('',#18449,12.9);
#2116=CIRCLE('',#18450,5.025);
#2117=CIRCLE('',#18451,12.9);
#2118=CIRCLE('',#18452,12.9);
#2119=CIRCLE('',#18454,12.5);
#2120=CIRCLE('',#18456,12.5);
#2121=CIRCLE('',#18458,12.5);
#2122=CIRCLE('',#18460,12.5);
#2123=CIRCLE('',#18462,12.5);
#2124=CIRCLE('',#18464,12.5);
#2125=CIRCLE('',#18466,12.5);
#2126=CIRCLE('',#18468,12.5);
#2127=CIRCLE('',#18470,12.5);
#2128=CIRCLE('',#18472,50.5);
#2129=CIRCLE('',#18491,0.700000000000003);
#2130=CIRCLE('',#18503,0.700000000000003);
#2131=CIRCLE('',#18515,0.700000000000003);
#2132=CIRCLE('',#18557,0.700000000000003);
#2133=CIRCLE('',#18569,0.700000000000003);
#2134=CIRCLE('',#18581,0.700000000000003);
#2135=CIRCLE('',#18587,1.5);
#2136=CIRCLE('',#18589,1.5);
#2137=CIRCLE('',#18591,1.5);
#2138=CIRCLE('',#18593,1.5);
#2139=CIRCLE('',#18595,1.5);
#2140=CIRCLE('',#18597,5.025);
#2352=FACE_OUTER_BOUND('',#3346,.T.);
#2353=FACE_OUTER_BOUND('',#3347,.T.);
#2354=FACE_OUTER_BOUND('',#3348,.T.);
#2355=FACE_OUTER_BOUND('',#3349,.T.);
#2356=FACE_OUTER_BOUND('',#3350,.T.);
#2357=FACE_OUTER_BOUND('',#3351,.T.);
#2358=FACE_OUTER_BOUND('',#3352,.T.);
#2359=FACE_OUTER_BOUND('',#3353,.T.);
#2360=FACE_OUTER_BOUND('',#3354,.T.);
#2361=FACE_OUTER_BOUND('',#3355,.T.);
#2362=FACE_OUTER_BOUND('',#3356,.T.);
#2363=FACE_OUTER_BOUND('',#3357,.T.);
#2364=FACE_OUTER_BOUND('',#3358,.T.);
#2365=FACE_OUTER_BOUND('',#3359,.T.);
#2366=FACE_OUTER_BOUND('',#3360,.T.);
#2367=FACE_OUTER_BOUND('',#3361,.T.);
#2368=FACE_OUTER_BOUND('',#3362,.T.);
#2369=FACE_OUTER_BOUND('',#3363,.T.);
#2370=FACE_OUTER_BOUND('',#3364,.T.);
#2371=FACE_OUTER_BOUND('',#3365,.T.);
#2372=FACE_OUTER_BOUND('',#3366,.T.);
#2373=FACE_OUTER_BOUND('',#3367,.T.);
#2374=FACE_OUTER_BOUND('',#3368,.T.);
#2375=FACE_OUTER_BOUND('',#3369,.T.);
#2376=FACE_OUTER_BOUND('',#3370,.T.);
#2377=FACE_OUTER_BOUND('',#3371,.T.);
#2378=FACE_OUTER_BOUND('',#3372,.T.);
#2379=FACE_OUTER_BOUND('',#3373,.T.);
#2380=FACE_OUTER_BOUND('',#3374,.T.);
#2381=FACE_OUTER_BOUND('',#3375,.T.);
#2382=FACE_OUTER_BOUND('',#3376,.T.);
#2383=FACE_OUTER_BOUND('',#3377,.T.);
#2384=FACE_OUTER_BOUND('',#3378,.T.);
#2385=FACE_OUTER_BOUND('',#3379,.T.);
#2386=FACE_OUTER_BOUND('',#3380,.T.);
#2387=FACE_OUTER_BOUND('',#3381,.T.);
#2388=FACE_OUTER_BOUND('',#3382,.T.);
#2389=FACE_OUTER_BOUND('',#3383,.T.);
#2390=FACE_OUTER_BOUND('',#3384,.T.);
#2391=FACE_OUTER_BOUND('',#3385,.T.);
#2392=FACE_OUTER_BOUND('',#3386,.T.);
#2393=FACE_OUTER_BOUND('',#3387,.T.);
#2394=FACE_OUTER_BOUND('',#3388,.T.);
#2395=FACE_OUTER_BOUND('',#3389,.T.);
#2396=FACE_OUTER_BOUND('',#3390,.T.);
#2397=FACE_OUTER_BOUND('',#3391,.T.);
#2398=FACE_OUTER_BOUND('',#3392,.T.);
#2399=FACE_OUTER_BOUND('',#3393,.T.);
#2400=FACE_OUTER_BOUND('',#3394,.T.);
#2401=FACE_OUTER_BOUND('',#3395,.T.);
#2402=FACE_OUTER_BOUND('',#3396,.T.);
#2403=FACE_OUTER_BOUND('',#3397,.T.);
#2404=FACE_OUTER_BOUND('',#3398,.T.);
#2405=FACE_OUTER_BOUND('',#3399,.T.);
#2406=FACE_OUTER_BOUND('',#3400,.T.);
#2407=FACE_OUTER_BOUND('',#3401,.T.);
#2408=FACE_OUTER_BOUND('',#3402,.T.);
#2409=FACE_OUTER_BOUND('',#3403,.T.);
#2410=FACE_OUTER_BOUND('',#3404,.T.);
#2411=FACE_OUTER_BOUND('',#3405,.T.);
#2412=FACE_OUTER_BOUND('',#3406,.T.);
#2413=FACE_OUTER_BOUND('',#3407,.T.);
#2414=FACE_OUTER_BOUND('',#3409,.T.);
#2415=FACE_OUTER_BOUND('',#3410,.T.);
#2416=FACE_OUTER_BOUND('',#3411,.T.);
#2417=FACE_OUTER_BOUND('',#3412,.T.);
#2418=FACE_OUTER_BOUND('',#3413,.T.);
#2419=FACE_OUTER_BOUND('',#3414,.T.);
#2420=FACE_OUTER_BOUND('',#3415,.T.);
#2421=FACE_OUTER_BOUND('',#3416,.T.);
#2422=FACE_OUTER_BOUND('',#3417,.T.);
#2423=FACE_OUTER_BOUND('',#3418,.T.);
#2424=FACE_OUTER_BOUND('',#3419,.T.);
#2425=FACE_OUTER_BOUND('',#3420,.T.);
#2426=FACE_OUTER_BOUND('',#3421,.T.);
#2427=FACE_OUTER_BOUND('',#3422,.T.);
#2428=FACE_OUTER_BOUND('',#3423,.T.);
#2429=FACE_OUTER_BOUND('',#3424,.T.);
#2430=FACE_OUTER_BOUND('',#3425,.T.);
#2431=FACE_OUTER_BOUND('',#3426,.T.);
#2432=FACE_OUTER_BOUND('',#3427,.T.);
#2433=FACE_OUTER_BOUND('',#3428,.T.);
#2434=FACE_OUTER_BOUND('',#3429,.T.);
#2435=FACE_OUTER_BOUND('',#3430,.T.);
#2436=FACE_OUTER_BOUND('',#3431,.T.);
#2437=FACE_OUTER_BOUND('',#3432,.T.);
#2438=FACE_OUTER_BOUND('',#3433,.T.);
#2439=FACE_OUTER_BOUND('',#3434,.T.);
#2440=FACE_OUTER_BOUND('',#3435,.T.);
#2441=FACE_OUTER_BOUND('',#3436,.T.);
#2442=FACE_OUTER_BOUND('',#3437,.T.);
#2443=FACE_OUTER_BOUND('',#3438,.T.);
#2444=FACE_OUTER_BOUND('',#3439,.T.);
#2445=FACE_OUTER_BOUND('',#3440,.T.);
#2446=FACE_OUTER_BOUND('',#3441,.T.);
#2447=FACE_OUTER_BOUND('',#3442,.T.);
#2448=FACE_OUTER_BOUND('',#3443,.T.);
#2449=FACE_OUTER_BOUND('',#3444,.T.);
#2450=FACE_OUTER_BOUND('',#3445,.T.);
#2451=FACE_OUTER_BOUND('',#3446,.T.);
#2452=FACE_OUTER_BOUND('',#3447,.T.);
#2453=FACE_OUTER_BOUND('',#3448,.T.);
#2454=FACE_OUTER_BOUND('',#3449,.T.);
#2455=FACE_OUTER_BOUND('',#3450,.T.);
#2456=FACE_OUTER_BOUND('',#3451,.T.);
#2457=FACE_OUTER_BOUND('',#3452,.T.);
#2458=FACE_OUTER_BOUND('',#3453,.T.);
#2459=FACE_OUTER_BOUND('',#3454,.T.);
#2460=FACE_OUTER_BOUND('',#3455,.T.);
#2461=FACE_OUTER_BOUND('',#3456,.T.);
#2462=FACE_OUTER_BOUND('',#3457,.T.);
#2463=FACE_OUTER_BOUND('',#3458,.T.);
#2464=FACE_OUTER_BOUND('',#3459,.T.);
#2465=FACE_OUTER_BOUND('',#3460,.T.);
#2466=FACE_OUTER_BOUND('',#3461,.T.);
#2467=FACE_OUTER_BOUND('',#3462,.T.);
#2468=FACE_OUTER_BOUND('',#3463,.T.);
#2469=FACE_OUTER_BOUND('',#3464,.T.);
#2470=FACE_OUTER_BOUND('',#3465,.T.);
#2471=FACE_OUTER_BOUND('',#3466,.T.);
#2472=FACE_OUTER_BOUND('',#3467,.T.);
#2473=FACE_OUTER_BOUND('',#3468,.T.);
#2474=FACE_OUTER_BOUND('',#3469,.T.);
#2475=FACE_OUTER_BOUND('',#3470,.T.);
#2476=FACE_OUTER_BOUND('',#3471,.T.);
#2477=FACE_OUTER_BOUND('',#3472,.T.);
#2478=FACE_OUTER_BOUND('',#3473,.T.);
#2479=FACE_OUTER_BOUND('',#3474,.T.);
#2480=FACE_OUTER_BOUND('',#3475,.T.);
#2481=FACE_OUTER_BOUND('',#3476,.T.);
#2482=FACE_OUTER_BOUND('',#3477,.T.);
#2483=FACE_OUTER_BOUND('',#3478,.T.);
#2484=FACE_OUTER_BOUND('',#3479,.T.);
#2485=FACE_OUTER_BOUND('',#3480,.T.);
#2486=FACE_OUTER_BOUND('',#3481,.T.);
#2487=FACE_OUTER_BOUND('',#3482,.T.);
#2488=FACE_OUTER_BOUND('',#3483,.T.);
#2489=FACE_OUTER_BOUND('',#3484,.T.);
#2490=FACE_OUTER_BOUND('',#3485,.T.);
#2491=FACE_OUTER_BOUND('',#3486,.T.);
#2492=FACE_OUTER_BOUND('',#3487,.T.);
#2493=FACE_OUTER_BOUND('',#3488,.T.);
#2494=FACE_OUTER_BOUND('',#3489,.T.);
#2495=FACE_OUTER_BOUND('',#3490,.T.);
#2496=FACE_OUTER_BOUND('',#3491,.T.);
#2497=FACE_OUTER_BOUND('',#3492,.T.);
#2498=FACE_OUTER_BOUND('',#3493,.T.);
#2499=FACE_OUTER_BOUND('',#3494,.T.);
#2500=FACE_OUTER_BOUND('',#3495,.T.);
#2501=FACE_OUTER_BOUND('',#3496,.T.);
#2502=FACE_OUTER_BOUND('',#3497,.T.);
#2503=FACE_OUTER_BOUND('',#3498,.T.);
#2504=FACE_OUTER_BOUND('',#3499,.T.);
#2505=FACE_OUTER_BOUND('',#3500,.T.);
#2506=FACE_OUTER_BOUND('',#3501,.T.);
#2507=FACE_OUTER_BOUND('',#3502,.T.);
#2508=FACE_OUTER_BOUND('',#3503,.T.);
#2509=FACE_OUTER_BOUND('',#3504,.T.);
#2510=FACE_OUTER_BOUND('',#3505,.T.);
#2511=FACE_OUTER_BOUND('',#3506,.T.);
#2512=FACE_OUTER_BOUND('',#3507,.T.);
#2513=FACE_OUTER_BOUND('',#3508,.T.);
#2514=FACE_OUTER_BOUND('',#3509,.T.);
#2515=FACE_OUTER_BOUND('',#3510,.T.);
#2516=FACE_OUTER_BOUND('',#3511,.T.);
#2517=FACE_OUTER_BOUND('',#3512,.T.);
#2518=FACE_OUTER_BOUND('',#3513,.T.);
#2519=FACE_OUTER_BOUND('',#3514,.T.);
#2520=FACE_OUTER_BOUND('',#3515,.T.);
#2521=FACE_OUTER_BOUND('',#3516,.T.);
#2522=FACE_OUTER_BOUND('',#3517,.T.);
#2523=FACE_OUTER_BOUND('',#3518,.T.);
#2524=FACE_OUTER_BOUND('',#3519,.T.);
#2525=FACE_OUTER_BOUND('',#3520,.T.);
#2526=FACE_OUTER_BOUND('',#3521,.T.);
#2527=FACE_OUTER_BOUND('',#3522,.T.);
#2528=FACE_OUTER_BOUND('',#3523,.T.);
#2529=FACE_OUTER_BOUND('',#3524,.T.);
#2530=FACE_OUTER_BOUND('',#3525,.T.);
#2531=FACE_OUTER_BOUND('',#3526,.T.);
#2532=FACE_OUTER_BOUND('',#3527,.T.);
#2533=FACE_OUTER_BOUND('',#3528,.T.);
#2534=FACE_OUTER_BOUND('',#3529,.T.);
#2535=FACE_OUTER_BOUND('',#3530,.T.);
#2536=FACE_OUTER_BOUND('',#3531,.T.);
#2537=FACE_OUTER_BOUND('',#3532,.T.);
#2538=FACE_OUTER_BOUND('',#3533,.T.);
#2539=FACE_OUTER_BOUND('',#3534,.T.);
#2540=FACE_OUTER_BOUND('',#3535,.T.);
#2541=FACE_OUTER_BOUND('',#3536,.T.);
#2542=FACE_OUTER_BOUND('',#3537,.T.);
#2543=FACE_OUTER_BOUND('',#3538,.T.);
#2544=FACE_OUTER_BOUND('',#3539,.T.);
#2545=FACE_OUTER_BOUND('',#3540,.T.);
#2546=FACE_OUTER_BOUND('',#3541,.T.);
#2547=FACE_OUTER_BOUND('',#3542,.T.);
#2548=FACE_OUTER_BOUND('',#3543,.T.);
#2549=FACE_OUTER_BOUND('',#3544,.T.);
#2550=FACE_OUTER_BOUND('',#3545,.T.);
#2551=FACE_OUTER_BOUND('',#3546,.T.);
#2552=FACE_OUTER_BOUND('',#3547,.T.);
#2553=FACE_OUTER_BOUND('',#3548,.T.);
#2554=FACE_OUTER_BOUND('',#3549,.T.);
#2555=FACE_OUTER_BOUND('',#3550,.T.);
#2556=FACE_OUTER_BOUND('',#3551,.T.);
#2557=FACE_OUTER_BOUND('',#3552,.T.);
#2558=FACE_OUTER_BOUND('',#3553,.T.);
#2559=FACE_OUTER_BOUND('',#3554,.T.);
#2560=FACE_OUTER_BOUND('',#3555,.T.);
#2561=FACE_OUTER_BOUND('',#3556,.T.);
#2562=FACE_OUTER_BOUND('',#3557,.T.);
#2563=FACE_OUTER_BOUND('',#3558,.T.);
#2564=FACE_OUTER_BOUND('',#3559,.T.);
#2565=FACE_OUTER_BOUND('',#3560,.T.);
#2566=FACE_OUTER_BOUND('',#3561,.T.);
#2567=FACE_OUTER_BOUND('',#3562,.T.);
#2568=FACE_OUTER_BOUND('',#3563,.T.);
#2569=FACE_OUTER_BOUND('',#3564,.T.);
#2570=FACE_OUTER_BOUND('',#3565,.T.);
#2571=FACE_OUTER_BOUND('',#3566,.T.);
#2572=FACE_OUTER_BOUND('',#3567,.T.);
#2573=FACE_OUTER_BOUND('',#3568,.T.);
#2574=FACE_OUTER_BOUND('',#3569,.T.);
#2575=FACE_OUTER_BOUND('',#3570,.T.);
#2576=FACE_OUTER_BOUND('',#3571,.T.);
#2577=FACE_OUTER_BOUND('',#3572,.T.);
#2578=FACE_OUTER_BOUND('',#3573,.T.);
#2579=FACE_OUTER_BOUND('',#3574,.T.);
#2580=FACE_OUTER_BOUND('',#3575,.T.);
#2581=FACE_OUTER_BOUND('',#3576,.T.);
#2582=FACE_OUTER_BOUND('',#3577,.T.);
#2583=FACE_OUTER_BOUND('',#3578,.T.);
#2584=FACE_OUTER_BOUND('',#3579,.T.);
#2585=FACE_OUTER_BOUND('',#3580,.T.);
#2586=FACE_OUTER_BOUND('',#3581,.T.);
#2587=FACE_OUTER_BOUND('',#3582,.T.);
#2588=FACE_OUTER_BOUND('',#3583,.T.);
#2589=FACE_OUTER_BOUND('',#3584,.T.);
#2590=FACE_OUTER_BOUND('',#3585,.T.);
#2591=FACE_OUTER_BOUND('',#3586,.T.);
#2592=FACE_OUTER_BOUND('',#3587,.T.);
#2593=FACE_OUTER_BOUND('',#3588,.T.);
#2594=FACE_OUTER_BOUND('',#3589,.T.);
#2595=FACE_OUTER_BOUND('',#3590,.T.);
#2596=FACE_OUTER_BOUND('',#3591,.T.);
#2597=FACE_OUTER_BOUND('',#3592,.T.);
#2598=FACE_OUTER_BOUND('',#3593,.T.);
#2599=FACE_OUTER_BOUND('',#3594,.T.);
#2600=FACE_OUTER_BOUND('',#3595,.T.);
#2601=FACE_OUTER_BOUND('',#3596,.T.);
#2602=FACE_OUTER_BOUND('',#3597,.T.);
#2603=FACE_OUTER_BOUND('',#3598,.T.);
#2604=FACE_OUTER_BOUND('',#3599,.T.);
#2605=FACE_OUTER_BOUND('',#3600,.T.);
#2606=FACE_OUTER_BOUND('',#3601,.T.);
#2607=FACE_OUTER_BOUND('',#3602,.T.);
#2608=FACE_OUTER_BOUND('',#3603,.T.);
#2609=FACE_OUTER_BOUND('',#3604,.T.);
#2610=FACE_OUTER_BOUND('',#3605,.T.);
#2611=FACE_OUTER_BOUND('',#3606,.T.);
#2612=FACE_OUTER_BOUND('',#3607,.T.);
#2613=FACE_OUTER_BOUND('',#3608,.T.);
#2614=FACE_OUTER_BOUND('',#3609,.T.);
#2615=FACE_OUTER_BOUND('',#3610,.T.);
#2616=FACE_OUTER_BOUND('',#3611,.T.);
#2617=FACE_OUTER_BOUND('',#3612,.T.);
#2618=FACE_OUTER_BOUND('',#3613,.T.);
#2619=FACE_OUTER_BOUND('',#3614,.T.);
#2620=FACE_OUTER_BOUND('',#3615,.T.);
#2621=FACE_OUTER_BOUND('',#3616,.T.);
#2622=FACE_OUTER_BOUND('',#3617,.T.);
#2623=FACE_OUTER_BOUND('',#3618,.T.);
#2624=FACE_OUTER_BOUND('',#3619,.T.);
#2625=FACE_OUTER_BOUND('',#3620,.T.);
#2626=FACE_OUTER_BOUND('',#3621,.T.);
#2627=FACE_OUTER_BOUND('',#3622,.T.);
#2628=FACE_OUTER_BOUND('',#3623,.T.);
#2629=FACE_OUTER_BOUND('',#3624,.T.);
#2630=FACE_OUTER_BOUND('',#3625,.T.);
#2631=FACE_OUTER_BOUND('',#3626,.T.);
#2632=FACE_OUTER_BOUND('',#3627,.T.);
#2633=FACE_OUTER_BOUND('',#3628,.T.);
#2634=FACE_OUTER_BOUND('',#3629,.T.);
#2635=FACE_OUTER_BOUND('',#3630,.T.);
#2636=FACE_OUTER_BOUND('',#3631,.T.);
#2637=FACE_OUTER_BOUND('',#3632,.T.);
#2638=FACE_OUTER_BOUND('',#3633,.T.);
#2639=FACE_OUTER_BOUND('',#3634,.T.);
#2640=FACE_OUTER_BOUND('',#3635,.T.);
#2641=FACE_OUTER_BOUND('',#3636,.T.);
#2642=FACE_OUTER_BOUND('',#3637,.T.);
#2643=FACE_OUTER_BOUND('',#3638,.T.);
#2644=FACE_OUTER_BOUND('',#3639,.T.);
#2645=FACE_OUTER_BOUND('',#3640,.T.);
#2646=FACE_OUTER_BOUND('',#3641,.T.);
#2647=FACE_OUTER_BOUND('',#3642,.T.);
#2648=FACE_OUTER_BOUND('',#3643,.T.);
#2649=FACE_OUTER_BOUND('',#3644,.T.);
#2650=FACE_OUTER_BOUND('',#3645,.T.);
#2651=FACE_OUTER_BOUND('',#3646,.T.);
#2652=FACE_OUTER_BOUND('',#3647,.T.);
#2653=FACE_OUTER_BOUND('',#3648,.T.);
#2654=FACE_OUTER_BOUND('',#3649,.T.);
#2655=FACE_OUTER_BOUND('',#3650,.T.);
#2656=FACE_OUTER_BOUND('',#3651,.T.);
#2657=FACE_OUTER_BOUND('',#3652,.T.);
#2658=FACE_OUTER_BOUND('',#3653,.T.);
#2659=FACE_OUTER_BOUND('',#3654,.T.);
#2660=FACE_OUTER_BOUND('',#3655,.T.);
#2661=FACE_OUTER_BOUND('',#3656,.T.);
#2662=FACE_OUTER_BOUND('',#3657,.T.);
#2663=FACE_OUTER_BOUND('',#3658,.T.);
#2664=FACE_OUTER_BOUND('',#3659,.T.);
#2665=FACE_OUTER_BOUND('',#3660,.T.);
#2666=FACE_OUTER_BOUND('',#3661,.T.);
#2667=FACE_OUTER_BOUND('',#3662,.T.);
#2668=FACE_OUTER_BOUND('',#3663,.T.);
#2669=FACE_OUTER_BOUND('',#3664,.T.);
#2670=FACE_OUTER_BOUND('',#3665,.T.);
#2671=FACE_OUTER_BOUND('',#3666,.T.);
#2672=FACE_OUTER_BOUND('',#3667,.T.);
#2673=FACE_OUTER_BOUND('',#3668,.T.);
#2674=FACE_OUTER_BOUND('',#3669,.T.);
#2675=FACE_OUTER_BOUND('',#3670,.T.);
#2676=FACE_OUTER_BOUND('',#3671,.T.);
#2677=FACE_OUTER_BOUND('',#3672,.T.);
#2678=FACE_OUTER_BOUND('',#3673,.T.);
#2679=FACE_OUTER_BOUND('',#3674,.T.);
#2680=FACE_OUTER_BOUND('',#3675,.T.);
#2681=FACE_OUTER_BOUND('',#3676,.T.);
#2682=FACE_OUTER_BOUND('',#3677,.T.);
#2683=FACE_OUTER_BOUND('',#3678,.T.);
#2684=FACE_OUTER_BOUND('',#3679,.T.);
#2685=FACE_OUTER_BOUND('',#3680,.T.);
#2686=FACE_OUTER_BOUND('',#3681,.T.);
#2687=FACE_OUTER_BOUND('',#3682,.T.);
#2688=FACE_OUTER_BOUND('',#3683,.T.);
#2689=FACE_OUTER_BOUND('',#3684,.T.);
#2690=FACE_OUTER_BOUND('',#3685,.T.);
#2691=FACE_OUTER_BOUND('',#3686,.T.);
#2692=FACE_OUTER_BOUND('',#3687,.T.);
#2693=FACE_OUTER_BOUND('',#3688,.T.);
#2694=FACE_OUTER_BOUND('',#3689,.T.);
#2695=FACE_OUTER_BOUND('',#3690,.T.);
#2696=FACE_OUTER_BOUND('',#3691,.T.);
#2697=FACE_OUTER_BOUND('',#3692,.T.);
#2698=FACE_OUTER_BOUND('',#3693,.T.);
#2699=FACE_OUTER_BOUND('',#3694,.T.);
#2700=FACE_OUTER_BOUND('',#3695,.T.);
#2701=FACE_OUTER_BOUND('',#3696,.T.);
#2702=FACE_OUTER_BOUND('',#3697,.T.);
#2703=FACE_OUTER_BOUND('',#3698,.T.);
#2704=FACE_OUTER_BOUND('',#3699,.T.);
#2705=FACE_OUTER_BOUND('',#3700,.T.);
#2706=FACE_OUTER_BOUND('',#3701,.T.);
#2707=FACE_OUTER_BOUND('',#3702,.T.);
#2708=FACE_OUTER_BOUND('',#3703,.T.);
#2709=FACE_OUTER_BOUND('',#3704,.T.);
#2710=FACE_OUTER_BOUND('',#3705,.T.);
#2711=FACE_OUTER_BOUND('',#3706,.T.);
#2712=FACE_OUTER_BOUND('',#3707,.T.);
#2713=FACE_OUTER_BOUND('',#3708,.T.);
#2714=FACE_OUTER_BOUND('',#3709,.T.);
#2715=FACE_OUTER_BOUND('',#3710,.T.);
#2716=FACE_OUTER_BOUND('',#3711,.T.);
#2717=FACE_OUTER_BOUND('',#3712,.T.);
#2718=FACE_OUTER_BOUND('',#3713,.T.);
#2719=FACE_OUTER_BOUND('',#3714,.T.);
#2720=FACE_OUTER_BOUND('',#3715,.T.);
#2721=FACE_OUTER_BOUND('',#3716,.T.);
#2722=FACE_OUTER_BOUND('',#3717,.T.);
#2723=FACE_OUTER_BOUND('',#3718,.T.);
#2724=FACE_OUTER_BOUND('',#3719,.T.);
#2725=FACE_OUTER_BOUND('',#3720,.T.);
#2726=FACE_OUTER_BOUND('',#3721,.T.);
#2727=FACE_OUTER_BOUND('',#3722,.T.);
#2728=FACE_OUTER_BOUND('',#3723,.T.);
#2729=FACE_OUTER_BOUND('',#3724,.T.);
#2730=FACE_OUTER_BOUND('',#3725,.T.);
#2731=FACE_OUTER_BOUND('',#3726,.T.);
#2732=FACE_OUTER_BOUND('',#3727,.T.);
#2733=FACE_OUTER_BOUND('',#3728,.T.);
#2734=FACE_OUTER_BOUND('',#3729,.T.);
#2735=FACE_OUTER_BOUND('',#3730,.T.);
#2736=FACE_OUTER_BOUND('',#3731,.T.);
#2737=FACE_OUTER_BOUND('',#3732,.T.);
#2738=FACE_OUTER_BOUND('',#3733,.T.);
#2739=FACE_OUTER_BOUND('',#3734,.T.);
#2740=FACE_OUTER_BOUND('',#3735,.T.);
#2741=FACE_OUTER_BOUND('',#3736,.T.);
#2742=FACE_OUTER_BOUND('',#3737,.T.);
#2743=FACE_OUTER_BOUND('',#3738,.T.);
#2744=FACE_OUTER_BOUND('',#3739,.T.);
#2745=FACE_OUTER_BOUND('',#3740,.T.);
#2746=FACE_OUTER_BOUND('',#3741,.T.);
#2747=FACE_OUTER_BOUND('',#3742,.T.);
#2748=FACE_OUTER_BOUND('',#3743,.T.);
#2749=FACE_OUTER_BOUND('',#3744,.T.);
#2750=FACE_OUTER_BOUND('',#3745,.T.);
#2751=FACE_OUTER_BOUND('',#3746,.T.);
#2752=FACE_OUTER_BOUND('',#3747,.T.);
#2753=FACE_OUTER_BOUND('',#3748,.T.);
#2754=FACE_OUTER_BOUND('',#3749,.T.);
#2755=FACE_OUTER_BOUND('',#3750,.T.);
#2756=FACE_OUTER_BOUND('',#3751,.T.);
#2757=FACE_OUTER_BOUND('',#3752,.T.);
#2758=FACE_OUTER_BOUND('',#3753,.T.);
#2759=FACE_OUTER_BOUND('',#3754,.T.);
#2760=FACE_OUTER_BOUND('',#3755,.T.);
#2761=FACE_OUTER_BOUND('',#3756,.T.);
#2762=FACE_OUTER_BOUND('',#3757,.T.);
#2763=FACE_OUTER_BOUND('',#3758,.T.);
#2764=FACE_OUTER_BOUND('',#3759,.T.);
#2765=FACE_OUTER_BOUND('',#3760,.T.);
#2766=FACE_OUTER_BOUND('',#3761,.T.);
#2767=FACE_OUTER_BOUND('',#3762,.T.);
#2768=FACE_OUTER_BOUND('',#3763,.T.);
#2769=FACE_OUTER_BOUND('',#3764,.T.);
#2770=FACE_OUTER_BOUND('',#3765,.T.);
#2771=FACE_OUTER_BOUND('',#3766,.T.);
#2772=FACE_OUTER_BOUND('',#3767,.T.);
#2773=FACE_OUTER_BOUND('',#3768,.T.);
#2774=FACE_OUTER_BOUND('',#3769,.T.);
#2775=FACE_OUTER_BOUND('',#3770,.T.);
#2776=FACE_OUTER_BOUND('',#3771,.T.);
#2777=FACE_OUTER_BOUND('',#3772,.T.);
#2778=FACE_OUTER_BOUND('',#3773,.T.);
#2779=FACE_OUTER_BOUND('',#3774,.T.);
#2780=FACE_OUTER_BOUND('',#3775,.T.);
#2781=FACE_OUTER_BOUND('',#3776,.T.);
#2782=FACE_OUTER_BOUND('',#3777,.T.);
#2783=FACE_OUTER_BOUND('',#3778,.T.);
#2784=FACE_OUTER_BOUND('',#3779,.T.);
#2785=FACE_OUTER_BOUND('',#3780,.T.);
#2786=FACE_OUTER_BOUND('',#3781,.T.);
#2787=FACE_OUTER_BOUND('',#3782,.T.);
#2788=FACE_OUTER_BOUND('',#3783,.T.);
#2789=FACE_OUTER_BOUND('',#3784,.T.);
#2790=FACE_OUTER_BOUND('',#3785,.T.);
#2791=FACE_OUTER_BOUND('',#3786,.T.);
#2792=FACE_OUTER_BOUND('',#3787,.T.);
#2793=FACE_OUTER_BOUND('',#3788,.T.);
#2794=FACE_OUTER_BOUND('',#3789,.T.);
#2795=FACE_OUTER_BOUND('',#3790,.T.);
#2796=FACE_OUTER_BOUND('',#3791,.T.);
#2797=FACE_OUTER_BOUND('',#3792,.T.);
#2798=FACE_OUTER_BOUND('',#3793,.T.);
#2799=FACE_OUTER_BOUND('',#3794,.T.);
#2800=FACE_OUTER_BOUND('',#3795,.T.);
#2801=FACE_OUTER_BOUND('',#3796,.T.);
#2802=FACE_OUTER_BOUND('',#3797,.T.);
#2803=FACE_OUTER_BOUND('',#3798,.T.);
#2804=FACE_OUTER_BOUND('',#3799,.T.);
#2805=FACE_OUTER_BOUND('',#3800,.T.);
#2806=FACE_OUTER_BOUND('',#3801,.T.);
#2807=FACE_OUTER_BOUND('',#3802,.T.);
#2808=FACE_OUTER_BOUND('',#3803,.T.);
#2809=FACE_OUTER_BOUND('',#3804,.T.);
#2810=FACE_OUTER_BOUND('',#3805,.T.);
#2811=FACE_OUTER_BOUND('',#3806,.T.);
#2812=FACE_OUTER_BOUND('',#3807,.T.);
#2813=FACE_OUTER_BOUND('',#3808,.T.);
#2814=FACE_OUTER_BOUND('',#3809,.T.);
#2815=FACE_OUTER_BOUND('',#3810,.T.);
#2816=FACE_OUTER_BOUND('',#3811,.T.);
#2817=FACE_OUTER_BOUND('',#3812,.T.);
#2818=FACE_OUTER_BOUND('',#3813,.T.);
#2819=FACE_OUTER_BOUND('',#3814,.T.);
#2820=FACE_OUTER_BOUND('',#3815,.T.);
#2821=FACE_OUTER_BOUND('',#3816,.T.);
#2822=FACE_OUTER_BOUND('',#3817,.T.);
#2823=FACE_OUTER_BOUND('',#3818,.T.);
#2824=FACE_OUTER_BOUND('',#3819,.T.);
#2825=FACE_OUTER_BOUND('',#3820,.T.);
#2826=FACE_OUTER_BOUND('',#3821,.T.);
#2827=FACE_OUTER_BOUND('',#3822,.T.);
#2828=FACE_OUTER_BOUND('',#3823,.T.);
#2829=FACE_OUTER_BOUND('',#3824,.T.);
#2830=FACE_OUTER_BOUND('',#3825,.T.);
#2831=FACE_OUTER_BOUND('',#3826,.T.);
#2832=FACE_OUTER_BOUND('',#3827,.T.);
#2833=FACE_OUTER_BOUND('',#3828,.T.);
#2834=FACE_OUTER_BOUND('',#3829,.T.);
#2835=FACE_OUTER_BOUND('',#3830,.T.);
#2836=FACE_OUTER_BOUND('',#3831,.T.);
#2837=FACE_OUTER_BOUND('',#3832,.T.);
#2838=FACE_OUTER_BOUND('',#3833,.T.);
#2839=FACE_OUTER_BOUND('',#3834,.T.);
#2840=FACE_OUTER_BOUND('',#3835,.T.);
#2841=FACE_OUTER_BOUND('',#3836,.T.);
#2842=FACE_OUTER_BOUND('',#3837,.T.);
#2843=FACE_OUTER_BOUND('',#3838,.T.);
#2844=FACE_OUTER_BOUND('',#3839,.T.);
#2845=FACE_OUTER_BOUND('',#3840,.T.);
#2846=FACE_OUTER_BOUND('',#3841,.T.);
#2847=FACE_OUTER_BOUND('',#3842,.T.);
#2848=FACE_OUTER_BOUND('',#3843,.T.);
#2849=FACE_OUTER_BOUND('',#3844,.T.);
#2850=FACE_OUTER_BOUND('',#3845,.T.);
#2851=FACE_OUTER_BOUND('',#3846,.T.);
#2852=FACE_OUTER_BOUND('',#3847,.T.);
#2853=FACE_OUTER_BOUND('',#3848,.T.);
#2854=FACE_OUTER_BOUND('',#3849,.T.);
#2855=FACE_OUTER_BOUND('',#3850,.T.);
#2856=FACE_OUTER_BOUND('',#3851,.T.);
#2857=FACE_OUTER_BOUND('',#3852,.T.);
#2858=FACE_OUTER_BOUND('',#3853,.T.);
#2859=FACE_OUTER_BOUND('',#3854,.T.);
#2860=FACE_OUTER_BOUND('',#3856,.T.);
#2861=FACE_OUTER_BOUND('',#3857,.T.);
#2862=FACE_OUTER_BOUND('',#3858,.T.);
#2863=FACE_OUTER_BOUND('',#3865,.T.);
#2864=FACE_OUTER_BOUND('',#3866,.T.);
#2865=FACE_OUTER_BOUND('',#3867,.T.);
#2866=FACE_OUTER_BOUND('',#3868,.T.);
#2867=FACE_OUTER_BOUND('',#3869,.T.);
#2868=FACE_OUTER_BOUND('',#3870,.T.);
#2869=FACE_OUTER_BOUND('',#3871,.T.);
#2870=FACE_OUTER_BOUND('',#3872,.T.);
#2871=FACE_OUTER_BOUND('',#3873,.T.);
#2872=FACE_OUTER_BOUND('',#3874,.T.);
#2873=FACE_OUTER_BOUND('',#3875,.T.);
#2874=FACE_OUTER_BOUND('',#3876,.T.);
#2875=FACE_OUTER_BOUND('',#3877,.T.);
#2876=FACE_OUTER_BOUND('',#3878,.T.);
#2877=FACE_OUTER_BOUND('',#3879,.T.);
#2878=FACE_OUTER_BOUND('',#3880,.T.);
#2879=FACE_OUTER_BOUND('',#3881,.T.);
#2880=FACE_OUTER_BOUND('',#3882,.T.);
#2881=FACE_OUTER_BOUND('',#3883,.T.);
#2882=FACE_OUTER_BOUND('',#3884,.T.);
#2883=FACE_OUTER_BOUND('',#3885,.T.);
#2884=FACE_OUTER_BOUND('',#3886,.T.);
#2885=FACE_OUTER_BOUND('',#3887,.T.);
#2886=FACE_OUTER_BOUND('',#3888,.T.);
#2887=FACE_OUTER_BOUND('',#3889,.T.);
#2888=FACE_OUTER_BOUND('',#3890,.T.);
#2889=FACE_OUTER_BOUND('',#3891,.T.);
#2890=FACE_OUTER_BOUND('',#3892,.T.);
#2891=FACE_OUTER_BOUND('',#3893,.T.);
#2892=FACE_OUTER_BOUND('',#3894,.T.);
#2893=FACE_OUTER_BOUND('',#3895,.T.);
#2894=FACE_OUTER_BOUND('',#3896,.T.);
#2895=FACE_OUTER_BOUND('',#3897,.T.);
#2896=FACE_OUTER_BOUND('',#3898,.T.);
#2897=FACE_OUTER_BOUND('',#3899,.T.);
#2898=FACE_OUTER_BOUND('',#3900,.T.);
#2899=FACE_OUTER_BOUND('',#3901,.T.);
#2900=FACE_OUTER_BOUND('',#3902,.T.);
#2901=FACE_OUTER_BOUND('',#3903,.T.);
#2902=FACE_OUTER_BOUND('',#3904,.T.);
#2903=FACE_OUTER_BOUND('',#3905,.T.);
#2904=FACE_OUTER_BOUND('',#3906,.T.);
#2905=FACE_OUTER_BOUND('',#3907,.T.);
#2906=FACE_OUTER_BOUND('',#3908,.T.);
#2907=FACE_OUTER_BOUND('',#3909,.T.);
#2908=FACE_OUTER_BOUND('',#3910,.T.);
#2909=FACE_OUTER_BOUND('',#3911,.T.);
#2910=FACE_OUTER_BOUND('',#3912,.T.);
#2911=FACE_OUTER_BOUND('',#3913,.T.);
#2912=FACE_OUTER_BOUND('',#3914,.T.);
#2913=FACE_OUTER_BOUND('',#3915,.T.);
#2914=FACE_OUTER_BOUND('',#3916,.T.);
#2915=FACE_OUTER_BOUND('',#3917,.T.);
#2916=FACE_OUTER_BOUND('',#3918,.T.);
#2917=FACE_OUTER_BOUND('',#3919,.T.);
#2918=FACE_OUTER_BOUND('',#3920,.T.);
#2919=FACE_OUTER_BOUND('',#3921,.T.);
#2920=FACE_OUTER_BOUND('',#3922,.T.);
#2921=FACE_OUTER_BOUND('',#3923,.T.);
#2922=FACE_OUTER_BOUND('',#3924,.T.);
#2923=FACE_OUTER_BOUND('',#3925,.T.);
#2924=FACE_OUTER_BOUND('',#3926,.T.);
#2925=FACE_OUTER_BOUND('',#3927,.T.);
#2926=FACE_OUTER_BOUND('',#3928,.T.);
#2927=FACE_OUTER_BOUND('',#3929,.T.);
#2928=FACE_OUTER_BOUND('',#3930,.T.);
#2929=FACE_OUTER_BOUND('',#3931,.T.);
#2930=FACE_OUTER_BOUND('',#3932,.T.);
#2931=FACE_OUTER_BOUND('',#3933,.T.);
#2932=FACE_OUTER_BOUND('',#3934,.T.);
#2933=FACE_OUTER_BOUND('',#3935,.T.);
#2934=FACE_OUTER_BOUND('',#3936,.T.);
#2935=FACE_OUTER_BOUND('',#3937,.T.);
#2936=FACE_OUTER_BOUND('',#3938,.T.);
#2937=FACE_OUTER_BOUND('',#3939,.T.);
#2938=FACE_OUTER_BOUND('',#3940,.T.);
#2939=FACE_OUTER_BOUND('',#3941,.T.);
#2940=FACE_OUTER_BOUND('',#3942,.T.);
#2941=FACE_OUTER_BOUND('',#3943,.T.);
#2942=FACE_OUTER_BOUND('',#3944,.T.);
#2943=FACE_OUTER_BOUND('',#3945,.T.);
#2944=FACE_OUTER_BOUND('',#3946,.T.);
#2945=FACE_OUTER_BOUND('',#3947,.T.);
#2946=FACE_OUTER_BOUND('',#3948,.T.);
#2947=FACE_OUTER_BOUND('',#3949,.T.);
#2948=FACE_OUTER_BOUND('',#3950,.T.);
#2949=FACE_OUTER_BOUND('',#3951,.T.);
#2950=FACE_OUTER_BOUND('',#3952,.T.);
#2951=FACE_OUTER_BOUND('',#3953,.T.);
#2952=FACE_OUTER_BOUND('',#3954,.T.);
#2953=FACE_OUTER_BOUND('',#3955,.T.);
#2954=FACE_OUTER_BOUND('',#3956,.T.);
#2955=FACE_OUTER_BOUND('',#3957,.T.);
#2956=FACE_OUTER_BOUND('',#3958,.T.);
#2957=FACE_OUTER_BOUND('',#3959,.T.);
#2958=FACE_OUTER_BOUND('',#3960,.T.);
#2959=FACE_OUTER_BOUND('',#3961,.T.);
#2960=FACE_OUTER_BOUND('',#3962,.T.);
#2961=FACE_OUTER_BOUND('',#3963,.T.);
#2962=FACE_OUTER_BOUND('',#3964,.T.);
#2963=FACE_OUTER_BOUND('',#3965,.T.);
#2964=FACE_OUTER_BOUND('',#3966,.T.);
#2965=FACE_OUTER_BOUND('',#3967,.T.);
#2966=FACE_OUTER_BOUND('',#3968,.T.);
#2967=FACE_OUTER_BOUND('',#3969,.T.);
#2968=FACE_OUTER_BOUND('',#3970,.T.);
#2969=FACE_OUTER_BOUND('',#3971,.T.);
#2970=FACE_OUTER_BOUND('',#3972,.T.);
#2971=FACE_OUTER_BOUND('',#3973,.T.);
#2972=FACE_OUTER_BOUND('',#3974,.T.);
#2973=FACE_OUTER_BOUND('',#3975,.T.);
#2974=FACE_OUTER_BOUND('',#3976,.T.);
#2975=FACE_OUTER_BOUND('',#3977,.T.);
#2976=FACE_OUTER_BOUND('',#3978,.T.);
#2977=FACE_OUTER_BOUND('',#3979,.T.);
#2978=FACE_OUTER_BOUND('',#3980,.T.);
#2979=FACE_OUTER_BOUND('',#3981,.T.);
#2980=FACE_OUTER_BOUND('',#3982,.T.);
#2981=FACE_OUTER_BOUND('',#3983,.T.);
#2982=FACE_OUTER_BOUND('',#3984,.T.);
#2983=FACE_OUTER_BOUND('',#3985,.T.);
#2984=FACE_OUTER_BOUND('',#3986,.T.);
#2985=FACE_OUTER_BOUND('',#3987,.T.);
#2986=FACE_OUTER_BOUND('',#3988,.T.);
#3346=EDGE_LOOP('',(#10781,#10782,#10783,#10784));
#3347=EDGE_LOOP('',(#10785,#10786,#10787,#10788));
#3348=EDGE_LOOP('',(#10789,#10790,#10791,#10792,#10793,#10794));
#3349=EDGE_LOOP('',(#10795,#10796,#10797,#10798,#10799));
#3350=EDGE_LOOP('',(#10800,#10801,#10802,#10803));
#3351=EDGE_LOOP('',(#10804,#10805,#10806,#10807,#10808,#10809));
#3352=EDGE_LOOP('',(#10810,#10811,#10812,#10813));
#3353=EDGE_LOOP('',(#10814,#10815,#10816,#10817,#10818,#10819));
#3354=EDGE_LOOP('',(#10820,#10821,#10822,#10823,#10824));
#3355=EDGE_LOOP('',(#10825,#10826,#10827,#10828,#10829,#10830));
#3356=EDGE_LOOP('',(#10831,#10832,#10833,#10834));
#3357=EDGE_LOOP('',(#10835,#10836,#10837,#10838,#10839));
#3358=EDGE_LOOP('',(#10840,#10841,#10842,#10843));
#3359=EDGE_LOOP('',(#10844,#10845,#10846,#10847,#10848,#10849));
#3360=EDGE_LOOP('',(#10850,#10851,#10852,#10853,#10854));
#3361=EDGE_LOOP('',(#10855,#10856,#10857,#10858,#10859,#10860));
#3362=EDGE_LOOP('',(#10861,#10862,#10863,#10864));
#3363=EDGE_LOOP('',(#10865,#10866,#10867,#10868,#10869));
#3364=EDGE_LOOP('',(#10870,#10871,#10872,#10873,#10874));
#3365=EDGE_LOOP('',(#10875,#10876,#10877,#10878));
#3366=EDGE_LOOP('',(#10879,#10880,#10881,#10882,#10883,#10884));
#3367=EDGE_LOOP('',(#10885,#10886,#10887,#10888,#10889,#10890));
#3368=EDGE_LOOP('',(#10891,#10892,#10893,#10894,#10895));
#3369=EDGE_LOOP('',(#10896,#10897,#10898,#10899));
#3370=EDGE_LOOP('',(#10900,#10901,#10902,#10903,#10904,#10905));
#3371=EDGE_LOOP('',(#10906,#10907,#10908,#10909,#10910));
#3372=EDGE_LOOP('',(#10911,#10912,#10913,#10914,#10915,#10916));
#3373=EDGE_LOOP('',(#10917,#10918,#10919,#10920));
#3374=EDGE_LOOP('',(#10921,#10922,#10923,#10924,#10925));
#3375=EDGE_LOOP('',(#10926,#10927,#10928,#10929,#10930));
#3376=EDGE_LOOP('',(#10931,#10932,#10933,#10934,#10935,#10936));
#3377=EDGE_LOOP('',(#10937,#10938,#10939,#10940));
#3378=EDGE_LOOP('',(#10941,#10942,#10943,#10944,#10945));
#3379=EDGE_LOOP('',(#10946,#10947,#10948,#10949,#10950));
#3380=EDGE_LOOP('',(#10951,#10952,#10953,#10954,#10955,#10956));
#3381=EDGE_LOOP('',(#10957,#10958,#10959,#10960));
#3382=EDGE_LOOP('',(#10961,#10962,#10963,#10964,#10965));
#3383=EDGE_LOOP('',(#10966,#10967,#10968,#10969,#10970));
#3384=EDGE_LOOP('',(#10971,#10972,#10973,#10974,#10975,#10976));
#3385=EDGE_LOOP('',(#10977,#10978,#10979,#10980));
#3386=EDGE_LOOP('',(#10981,#10982,#10983,#10984,#10985));
#3387=EDGE_LOOP('',(#10986,#10987,#10988,#10989,#10990));
#3388=EDGE_LOOP('',(#10991,#10992,#10993,#10994,#10995,#10996));
#3389=EDGE_LOOP('',(#10997,#10998,#10999,#11000));
#3390=EDGE_LOOP('',(#11001,#11002,#11003,#11004,#11005));
#3391=EDGE_LOOP('',(#11006,#11007,#11008,#11009,#11010));
#3392=EDGE_LOOP('',(#11011,#11012,#11013,#11014,#11015,#11016));
#3393=EDGE_LOOP('',(#11017,#11018,#11019,#11020));
#3394=EDGE_LOOP('',(#11021,#11022,#11023,#11024,#11025));
#3395=EDGE_LOOP('',(#11026,#11027,#11028,#11029,#11030));
#3396=EDGE_LOOP('',(#11031,#11032,#11033,#11034,#11035,#11036));
#3397=EDGE_LOOP('',(#11037,#11038,#11039,#11040));
#3398=EDGE_LOOP('',(#11041,#11042,#11043,#11044,#11045));
#3399=EDGE_LOOP('',(#11046,#11047,#11048,#11049,#11050));
#3400=EDGE_LOOP('',(#11051,#11052,#11053,#11054,#11055,#11056));
#3401=EDGE_LOOP('',(#11057,#11058,#11059,#11060));
#3402=EDGE_LOOP('',(#11061,#11062,#11063,#11064,#11065));
#3403=EDGE_LOOP('',(#11066,#11067,#11068,#11069,#11070,#11071));
#3404=EDGE_LOOP('',(#11072,#11073,#11074,#11075,#11076,#11077));
#3405=EDGE_LOOP('',(#11078,#11079,#11080,#11081,#11082,#11083));
#3406=EDGE_LOOP('',(#11084,#11085,#11086,#11087,#11088,#11089));
#3407=EDGE_LOOP('',(#11090,#11091,#11092,#11093,#11094,#11095,#11096,#11097,
#11098,#11099,#11100,#11101,#11102,#11103,#11104,#11105,#11106,#11107,#11108,
#11109,#11110,#11111,#11112,#11113,#11114,#11115,#11116,#11117,#11118,#11119,
#11120,#11121,#11122,#11123,#11124,#11125,#11126,#11127,#11128,#11129,#11130,
#11131,#11132,#11133,#11134,#11135,#11136,#11137,#11138,#11139,#11140,#11141,
#11142,#11143,#11144,#11145,#11146,#11147,#11148,#11149,#11150,#11151,#11152,
#11153,#11154,#11155,#11156,#11157,#11158,#11159,#11160,#11161,#11162,#11163,
#11164,#11165,#11166,#11167,#11168,#11169,#11170,#11171,#11172,#11173,#11174,
#11175,#11176,#11177,#11178,#11179,#11180,#11181,#11182,#11183,#11184,#11185,
#11186,#11187,#11188,#11189,#11190,#11191,#11192,#11193,#11194,#11195,#11196,
#11197,#11198,#11199,#11200,#11201,#11202,#11203,#11204,#11205,#11206,#11207,
#11208,#11209,#11210,#11211,#11212,#11213,#11214,#11215,#11216,#11217,#11218,
#11219,#11220,#11221,#11222,#11223,#11224,#11225,#11226,#11227,#11228,#11229,
#11230,#11231,#11232,#11233,#11234,#11235,#11236,#11237,#11238,#11239,#11240,
#11241,#11242,#11243,#11244,#11245,#11246,#11247,#11248,#11249,#11250,#11251,
#11252,#11253,#11254,#11255,#11256,#11257,#11258,#11259,#11260,#11261,#11262,
#11263,#11264,#11265,#11266,#11267,#11268,#11269));
#3408=EDGE_LOOP('',(#11270));
#3409=EDGE_LOOP('',(#11271,#11272,#11273,#11274,#11275,#11276));
#3410=EDGE_LOOP('',(#11277,#11278,#11279,#11280));
#3411=EDGE_LOOP('',(#11281,#11282,#11283,#11284,#11285));
#3412=EDGE_LOOP('',(#11286,#11287,#11288,#11289,#11290,#11291));
#3413=EDGE_LOOP('',(#11292,#11293,#11294,#11295));
#3414=EDGE_LOOP('',(#11296,#11297,#11298,#11299,#11300));
#3415=EDGE_LOOP('',(#11301,#11302,#11303,#11304,#11305));
#3416=EDGE_LOOP('',(#11306,#11307,#11308,#11309,#11310,#11311));
#3417=EDGE_LOOP('',(#11312,#11313,#11314,#11315));
#3418=EDGE_LOOP('',(#11316,#11317,#11318,#11319,#11320));
#3419=EDGE_LOOP('',(#11321,#11322,#11323,#11324,#11325));
#3420=EDGE_LOOP('',(#11326,#11327,#11328,#11329,#11330,#11331));
#3421=EDGE_LOOP('',(#11332,#11333,#11334,#11335));
#3422=EDGE_LOOP('',(#11336,#11337,#11338,#11339));
#3423=EDGE_LOOP('',(#11340,#11341,#11342,#11343));
#3424=EDGE_LOOP('',(#11344,#11345,#11346,#11347,#11348,#11349));
#3425=EDGE_LOOP('',(#11350,#11351,#11352,#11353,#11354));
#3426=EDGE_LOOP('',(#11355,#11356,#11357,#11358));
#3427=EDGE_LOOP('',(#11359,#11360,#11361,#11362,#11363,#11364));
#3428=EDGE_LOOP('',(#11365,#11366,#11367,#11368));
#3429=EDGE_LOOP('',(#11369,#11370,#11371,#11372,#11373));
#3430=EDGE_LOOP('',(#11374,#11375,#11376,#11377,#11378));
#3431=EDGE_LOOP('',(#11379,#11380,#11381,#11382,#11383,#11384));
#3432=EDGE_LOOP('',(#11385,#11386,#11387,#11388));
#3433=EDGE_LOOP('',(#11389,#11390,#11391,#11392,#11393));
#3434=EDGE_LOOP('',(#11394,#11395,#11396,#11397,#11398));
#3435=EDGE_LOOP('',(#11399,#11400,#11401,#11402,#11403,#11404));
#3436=EDGE_LOOP('',(#11405,#11406,#11407,#11408));
#3437=EDGE_LOOP('',(#11409,#11410,#11411,#11412,#11413));
#3438=EDGE_LOOP('',(#11414,#11415,#11416,#11417,#11418));
#3439=EDGE_LOOP('',(#11419,#11420,#11421,#11422,#11423,#11424));
#3440=EDGE_LOOP('',(#11425,#11426,#11427,#11428));
#3441=EDGE_LOOP('',(#11429,#11430,#11431,#11432,#11433));
#3442=EDGE_LOOP('',(#11434,#11435,#11436,#11437,#11438));
#3443=EDGE_LOOP('',(#11439,#11440,#11441,#11442,#11443,#11444));
#3444=EDGE_LOOP('',(#11445,#11446,#11447,#11448));
#3445=EDGE_LOOP('',(#11449,#11450,#11451,#11452,#11453));
#3446=EDGE_LOOP('',(#11454,#11455,#11456,#11457,#11458));
#3447=EDGE_LOOP('',(#11459,#11460,#11461,#11462,#11463,#11464));
#3448=EDGE_LOOP('',(#11465,#11466,#11467,#11468));
#3449=EDGE_LOOP('',(#11469,#11470,#11471,#11472));
#3450=EDGE_LOOP('',(#11473,#11474,#11475,#11476,#11477,#11478));
#3451=EDGE_LOOP('',(#11479,#11480,#11481,#11482,#11483,#11484));
#3452=EDGE_LOOP('',(#11485,#11486,#11487,#11488,#11489,#11490));
#3453=EDGE_LOOP('',(#11491,#11492,#11493,#11494));
#3454=EDGE_LOOP('',(#11495,#11496,#11497,#11498));
#3455=EDGE_LOOP('',(#11499,#11500,#11501,#11502));
#3456=EDGE_LOOP('',(#11503,#11504,#11505,#11506));
#3457=EDGE_LOOP('',(#11507,#11508,#11509,#11510,#11511,#11512));
#3458=EDGE_LOOP('',(#11513,#11514,#11515,#11516,#11517,#11518));
#3459=EDGE_LOOP('',(#11519,#11520,#11521,#11522,#11523,#11524));
#3460=EDGE_LOOP('',(#11525,#11526,#11527,#11528,#11529,#11530));
#3461=EDGE_LOOP('',(#11531,#11532,#11533,#11534,#11535,#11536));
#3462=EDGE_LOOP('',(#11537,#11538,#11539,#11540,#11541,#11542));
#3463=EDGE_LOOP('',(#11543,#11544,#11545,#11546));
#3464=EDGE_LOOP('',(#11547,#11548,#11549,#11550));
#3465=EDGE_LOOP('',(#11551,#11552,#11553,#11554));
#3466=EDGE_LOOP('',(#11555,#11556,#11557,#11558));
#3467=EDGE_LOOP('',(#11559,#11560,#11561,#11562));
#3468=EDGE_LOOP('',(#11563,#11564,#11565,#11566,#11567));
#3469=EDGE_LOOP('',(#11568,#11569,#11570,#11571,#11572,#11573));
#3470=EDGE_LOOP('',(#11574,#11575,#11576,#11577));
#3471=EDGE_LOOP('',(#11578,#11579,#11580,#11581,#11582));
#3472=EDGE_LOOP('',(#11583,#11584,#11585,#11586,#11587,#11588));
#3473=EDGE_LOOP('',(#11589,#11590,#11591,#11592,#11593));
#3474=EDGE_LOOP('',(#11594,#11595,#11596,#11597,#11598,#11599));
#3475=EDGE_LOOP('',(#11600,#11601,#11602,#11603));
#3476=EDGE_LOOP('',(#11604,#11605,#11606,#11607,#11608));
#3477=EDGE_LOOP('',(#11609,#11610,#11611,#11612,#11613));
#3478=EDGE_LOOP('',(#11614,#11615,#11616,#11617,#11618,#11619));
#3479=EDGE_LOOP('',(#11620,#11621,#11622,#11623));
#3480=EDGE_LOOP('',(#11624,#11625,#11626,#11627,#11628));
#3481=EDGE_LOOP('',(#11629,#11630,#11631,#11632,#11633));
#3482=EDGE_LOOP('',(#11634,#11635,#11636,#11637,#11638,#11639));
#3483=EDGE_LOOP('',(#11640,#11641,#11642,#11643));
#3484=EDGE_LOOP('',(#11644,#11645,#11646,#11647));
#3485=EDGE_LOOP('',(#11648,#11649,#11650,#11651));
#3486=EDGE_LOOP('',(#11652,#11653,#11654,#11655,#11656,#11657));
#3487=EDGE_LOOP('',(#11658,#11659,#11660,#11661,#11662));
#3488=EDGE_LOOP('',(#11663,#11664,#11665,#11666));
#3489=EDGE_LOOP('',(#11667,#11668,#11669,#11670,#11671,#11672));
#3490=EDGE_LOOP('',(#11673,#11674,#11675,#11676));
#3491=EDGE_LOOP('',(#11677,#11678,#11679,#11680,#11681));
#3492=EDGE_LOOP('',(#11682,#11683,#11684,#11685,#11686));
#3493=EDGE_LOOP('',(#11687,#11688,#11689,#11690,#11691,#11692));
#3494=EDGE_LOOP('',(#11693,#11694,#11695,#11696));
#3495=EDGE_LOOP('',(#11697,#11698,#11699,#11700,#11701));
#3496=EDGE_LOOP('',(#11702,#11703,#11704,#11705,#11706));
#3497=EDGE_LOOP('',(#11707,#11708,#11709,#11710,#11711,#11712));
#3498=EDGE_LOOP('',(#11713,#11714,#11715,#11716));
#3499=EDGE_LOOP('',(#11717,#11718,#11719,#11720,#11721));
#3500=EDGE_LOOP('',(#11722,#11723,#11724,#11725,#11726));
#3501=EDGE_LOOP('',(#11727,#11728,#11729,#11730,#11731,#11732));
#3502=EDGE_LOOP('',(#11733,#11734,#11735,#11736));
#3503=EDGE_LOOP('',(#11737,#11738,#11739,#11740,#11741));
#3504=EDGE_LOOP('',(#11742,#11743,#11744,#11745,#11746));
#3505=EDGE_LOOP('',(#11747,#11748,#11749,#11750,#11751,#11752));
#3506=EDGE_LOOP('',(#11753,#11754,#11755,#11756));
#3507=EDGE_LOOP('',(#11757,#11758,#11759,#11760));
#3508=EDGE_LOOP('',(#11761,#11762,#11763,#11764,#11765,#11766));
#3509=EDGE_LOOP('',(#11767,#11768,#11769,#11770,#11771,#11772));
#3510=EDGE_LOOP('',(#11773,#11774,#11775,#11776,#11777,#11778));
#3511=EDGE_LOOP('',(#11779,#11780,#11781,#11782));
#3512=EDGE_LOOP('',(#11783,#11784,#11785,#11786));
#3513=EDGE_LOOP('',(#11787,#11788,#11789,#11790));
#3514=EDGE_LOOP('',(#11791,#11792,#11793,#11794));
#3515=EDGE_LOOP('',(#11795,#11796,#11797,#11798));
#3516=EDGE_LOOP('',(#11799,#11800,#11801,#11802,#11803,#11804));
#3517=EDGE_LOOP('',(#11805,#11806,#11807,#11808,#11809,#11810));
#3518=EDGE_LOOP('',(#11811,#11812,#11813,#11814,#11815,#11816));
#3519=EDGE_LOOP('',(#11817,#11818,#11819,#11820,#11821,#11822));
#3520=EDGE_LOOP('',(#11823,#11824,#11825,#11826,#11827,#11828));
#3521=EDGE_LOOP('',(#11829,#11830,#11831,#11832));
#3522=EDGE_LOOP('',(#11833,#11834,#11835,#11836));
#3523=EDGE_LOOP('',(#11837,#11838,#11839,#11840));
#3524=EDGE_LOOP('',(#11841,#11842,#11843,#11844));
#3525=EDGE_LOOP('',(#11845,#11846,#11847,#11848,#11849));
#3526=EDGE_LOOP('',(#11850,#11851,#11852,#11853,#11854,#11855));
#3527=EDGE_LOOP('',(#11856,#11857,#11858,#11859));
#3528=EDGE_LOOP('',(#11860,#11861,#11862,#11863,#11864));
#3529=EDGE_LOOP('',(#11865,#11866,#11867,#11868,#11869));
#3530=EDGE_LOOP('',(#11870,#11871,#11872,#11873,#11874,#11875));
#3531=EDGE_LOOP('',(#11876,#11877,#11878,#11879));
#3532=EDGE_LOOP('',(#11880,#11881,#11882,#11883,#11884));
#3533=EDGE_LOOP('',(#11885,#11886,#11887,#11888,#11889));
#3534=EDGE_LOOP('',(#11890,#11891,#11892,#11893,#11894,#11895));
#3535=EDGE_LOOP('',(#11896,#11897,#11898,#11899));
#3536=EDGE_LOOP('',(#11900,#11901,#11902,#11903,#11904));
#3537=EDGE_LOOP('',(#11905,#11906,#11907,#11908,#11909));
#3538=EDGE_LOOP('',(#11910,#11911,#11912,#11913,#11914,#11915));
#3539=EDGE_LOOP('',(#11916,#11917,#11918,#11919));
#3540=EDGE_LOOP('',(#11920,#11921,#11922,#11923,#11924));
#3541=EDGE_LOOP('',(#11925,#11926,#11927,#11928,#11929));
#3542=EDGE_LOOP('',(#11930,#11931,#11932,#11933,#11934,#11935));
#3543=EDGE_LOOP('',(#11936,#11937,#11938,#11939));
#3544=EDGE_LOOP('',(#11940,#11941,#11942,#11943));
#3545=EDGE_LOOP('',(#11944,#11945,#11946,#11947));
#3546=EDGE_LOOP('',(#11948,#11949,#11950,#11951,#11952,#11953));
#3547=EDGE_LOOP('',(#11954,#11955,#11956,#11957,#11958));
#3548=EDGE_LOOP('',(#11959,#11960,#11961,#11962));
#3549=EDGE_LOOP('',(#11963,#11964,#11965,#11966,#11967,#11968));
#3550=EDGE_LOOP('',(#11969,#11970,#11971,#11972));
#3551=EDGE_LOOP('',(#11973,#11974,#11975,#11976,#11977));
#3552=EDGE_LOOP('',(#11978,#11979,#11980,#11981,#11982));
#3553=EDGE_LOOP('',(#11983,#11984,#11985,#11986,#11987,#11988));
#3554=EDGE_LOOP('',(#11989,#11990,#11991,#11992));
#3555=EDGE_LOOP('',(#11993,#11994,#11995,#11996,#11997));
#3556=EDGE_LOOP('',(#11998,#11999,#12000,#12001,#12002));
#3557=EDGE_LOOP('',(#12003,#12004,#12005,#12006,#12007,#12008));
#3558=EDGE_LOOP('',(#12009,#12010,#12011,#12012));
#3559=EDGE_LOOP('',(#12013,#12014,#12015,#12016,#12017));
#3560=EDGE_LOOP('',(#12018,#12019,#12020,#12021,#12022));
#3561=EDGE_LOOP('',(#12023,#12024,#12025,#12026,#12027,#12028));
#3562=EDGE_LOOP('',(#12029,#12030,#12031,#12032));
#3563=EDGE_LOOP('',(#12033,#12034,#12035,#12036));
#3564=EDGE_LOOP('',(#12037,#12038,#12039,#12040,#12041,#12042));
#3565=EDGE_LOOP('',(#12043,#12044,#12045,#12046,#12047,#12048));
#3566=EDGE_LOOP('',(#12049,#12050,#12051,#12052,#12053,#12054));
#3567=EDGE_LOOP('',(#12055,#12056,#12057,#12058,#12059,#12060));
#3568=EDGE_LOOP('',(#12061,#12062,#12063,#12064,#12065,#12066));
#3569=EDGE_LOOP('',(#12067,#12068,#12069,#12070));
#3570=EDGE_LOOP('',(#12071,#12072,#12073,#12074));
#3571=EDGE_LOOP('',(#12075,#12076,#12077,#12078));
#3572=EDGE_LOOP('',(#12079,#12080,#12081,#12082));
#3573=EDGE_LOOP('',(#12083,#12084,#12085,#12086));
#3574=EDGE_LOOP('',(#12087,#12088,#12089,#12090));
#3575=EDGE_LOOP('',(#12091,#12092,#12093,#12094,#12095,#12096));
#3576=EDGE_LOOP('',(#12097,#12098,#12099,#12100,#12101,#12102));
#3577=EDGE_LOOP('',(#12103,#12104,#12105,#12106,#12107,#12108));
#3578=EDGE_LOOP('',(#12109,#12110,#12111,#12112,#12113,#12114));
#3579=EDGE_LOOP('',(#12115,#12116,#12117,#12118));
#3580=EDGE_LOOP('',(#12119,#12120,#12121,#12122));
#3581=EDGE_LOOP('',(#12123,#12124,#12125,#12126));
#3582=EDGE_LOOP('',(#12127,#12128,#12129,#12130,#12131));
#3583=EDGE_LOOP('',(#12132,#12133,#12134,#12135,#12136,#12137));
#3584=EDGE_LOOP('',(#12138,#12139,#12140,#12141));
#3585=EDGE_LOOP('',(#12142,#12143,#12144,#12145,#12146));
#3586=EDGE_LOOP('',(#12147,#12148,#12149,#12150,#12151,#12152));
#3587=EDGE_LOOP('',(#12153,#12154,#12155,#12156,#12157));
#3588=EDGE_LOOP('',(#12158,#12159,#12160,#12161,#12162,#12163));
#3589=EDGE_LOOP('',(#12164,#12165,#12166,#12167));
#3590=EDGE_LOOP('',(#12168,#12169,#12170,#12171,#12172));
#3591=EDGE_LOOP('',(#12173,#12174,#12175,#12176,#12177));
#3592=EDGE_LOOP('',(#12178,#12179,#12180,#12181,#12182,#12183));
#3593=EDGE_LOOP('',(#12184,#12185,#12186,#12187));
#3594=EDGE_LOOP('',(#12188,#12189,#12190,#12191,#12192));
#3595=EDGE_LOOP('',(#12193,#12194,#12195,#12196,#12197));
#3596=EDGE_LOOP('',(#12198,#12199,#12200,#12201,#12202,#12203));
#3597=EDGE_LOOP('',(#12204,#12205,#12206,#12207));
#3598=EDGE_LOOP('',(#12208,#12209,#12210,#12211,#12212));
#3599=EDGE_LOOP('',(#12213,#12214,#12215,#12216,#12217));
#3600=EDGE_LOOP('',(#12218,#12219,#12220,#12221,#12222,#12223));
#3601=EDGE_LOOP('',(#12224,#12225,#12226,#12227));
#3602=EDGE_LOOP('',(#12228,#12229,#12230,#12231,#12232));
#3603=EDGE_LOOP('',(#12233,#12234,#12235,#12236,#12237));
#3604=EDGE_LOOP('',(#12238,#12239,#12240,#12241,#12242,#12243));
#3605=EDGE_LOOP('',(#12244,#12245,#12246,#12247));
#3606=EDGE_LOOP('',(#12248,#12249,#12250,#12251));
#3607=EDGE_LOOP('',(#12252,#12253,#12254,#12255));
#3608=EDGE_LOOP('',(#12256,#12257,#12258,#12259,#12260,#12261));
#3609=EDGE_LOOP('',(#12262,#12263,#12264,#12265,#12266));
#3610=EDGE_LOOP('',(#12267,#12268,#12269,#12270));
#3611=EDGE_LOOP('',(#12271,#12272,#12273,#12274,#12275,#12276));
#3612=EDGE_LOOP('',(#12277,#12278,#12279,#12280));
#3613=EDGE_LOOP('',(#12281,#12282,#12283,#12284,#12285));
#3614=EDGE_LOOP('',(#12286,#12287,#12288,#12289,#12290));
#3615=EDGE_LOOP('',(#12291,#12292,#12293,#12294,#12295,#12296));
#3616=EDGE_LOOP('',(#12297,#12298,#12299,#12300));
#3617=EDGE_LOOP('',(#12301,#12302,#12303,#12304,#12305));
#3618=EDGE_LOOP('',(#12306,#12307,#12308,#12309,#12310));
#3619=EDGE_LOOP('',(#12311,#12312,#12313,#12314,#12315,#12316));
#3620=EDGE_LOOP('',(#12317,#12318,#12319,#12320));
#3621=EDGE_LOOP('',(#12321,#12322,#12323,#12324));
#3622=EDGE_LOOP('',(#12325,#12326,#12327,#12328,#12329,#12330));
#3623=EDGE_LOOP('',(#12331,#12332,#12333,#12334,#12335,#12336));
#3624=EDGE_LOOP('',(#12337,#12338,#12339,#12340,#12341,#12342));
#3625=EDGE_LOOP('',(#12343,#12344,#12345,#12346,#12347,#12348));
#3626=EDGE_LOOP('',(#12349,#12350,#12351,#12352,#12353,#12354));
#3627=EDGE_LOOP('',(#12355,#12356,#12357,#12358));
#3628=EDGE_LOOP('',(#12359,#12360,#12361,#12362));
#3629=EDGE_LOOP('',(#12363,#12364,#12365,#12366));
#3630=EDGE_LOOP('',(#12367,#12368,#12369,#12370));
#3631=EDGE_LOOP('',(#12371,#12372,#12373,#12374));
#3632=EDGE_LOOP('',(#12375,#12376,#12377,#12378));
#3633=EDGE_LOOP('',(#12379,#12380,#12381,#12382));
#3634=EDGE_LOOP('',(#12383,#12384,#12385,#12386,#12387,#12388));
#3635=EDGE_LOOP('',(#12389,#12390,#12391,#12392,#12393,#12394));
#3636=EDGE_LOOP('',(#12395,#12396,#12397,#12398,#12399,#12400));
#3637=EDGE_LOOP('',(#12401,#12402,#12403,#12404));
#3638=EDGE_LOOP('',(#12405,#12406,#12407,#12408));
#3639=EDGE_LOOP('',(#12409,#12410,#12411,#12412,#12413));
#3640=EDGE_LOOP('',(#12414,#12415,#12416,#12417,#12418,#12419));
#3641=EDGE_LOOP('',(#12420,#12421,#12422,#12423));
#3642=EDGE_LOOP('',(#12424,#12425,#12426,#12427,#12428));
#3643=EDGE_LOOP('',(#12429,#12430,#12431,#12432,#12433));
#3644=EDGE_LOOP('',(#12434,#12435,#12436,#12437,#12438,#12439));
#3645=EDGE_LOOP('',(#12440,#12441,#12442,#12443));
#3646=EDGE_LOOP('',(#12444,#12445,#12446,#12447,#12448));
#3647=EDGE_LOOP('',(#12449,#12450,#12451,#12452,#12453));
#3648=EDGE_LOOP('',(#12454,#12455,#12456,#12457,#12458,#12459));
#3649=EDGE_LOOP('',(#12460,#12461,#12462,#12463));
#3650=EDGE_LOOP('',(#12464,#12465,#12466,#12467,#12468));
#3651=EDGE_LOOP('',(#12469,#12470,#12471,#12472,#12473));
#3652=EDGE_LOOP('',(#12474,#12475,#12476,#12477,#12478,#12479));
#3653=EDGE_LOOP('',(#12480,#12481,#12482,#12483));
#3654=EDGE_LOOP('',(#12484,#12485,#12486,#12487,#12488));
#3655=EDGE_LOOP('',(#12489,#12490,#12491,#12492,#12493));
#3656=EDGE_LOOP('',(#12494,#12495,#12496,#12497,#12498,#12499));
#3657=EDGE_LOOP('',(#12500,#12501,#12502,#12503));
#3658=EDGE_LOOP('',(#12504,#12505,#12506,#12507,#12508));
#3659=EDGE_LOOP('',(#12509,#12510,#12511,#12512,#12513));
#3660=EDGE_LOOP('',(#12514,#12515,#12516,#12517,#12518,#12519));
#3661=EDGE_LOOP('',(#12520,#12521,#12522,#12523));
#3662=EDGE_LOOP('',(#12524,#12525,#12526,#12527,#12528));
#3663=EDGE_LOOP('',(#12529,#12530,#12531,#12532,#12533));
#3664=EDGE_LOOP('',(#12534,#12535,#12536,#12537,#12538,#12539));
#3665=EDGE_LOOP('',(#12540,#12541,#12542,#12543));
#3666=EDGE_LOOP('',(#12544,#12545,#12546,#12547));
#3667=EDGE_LOOP('',(#12548,#12549,#12550,#12551));
#3668=EDGE_LOOP('',(#12552,#12553,#12554,#12555,#12556,#12557));
#3669=EDGE_LOOP('',(#12558,#12559,#12560,#12561,#12562));
#3670=EDGE_LOOP('',(#12563,#12564,#12565,#12566));
#3671=EDGE_LOOP('',(#12567,#12568,#12569,#12570,#12571,#12572));
#3672=EDGE_LOOP('',(#12573,#12574,#12575,#12576));
#3673=EDGE_LOOP('',(#12577,#12578,#12579,#12580,#12581));
#3674=EDGE_LOOP('',(#12582,#12583,#12584,#12585,#12586));
#3675=EDGE_LOOP('',(#12587,#12588,#12589,#12590,#12591,#12592));
#3676=EDGE_LOOP('',(#12593,#12594,#12595,#12596));
#3677=EDGE_LOOP('',(#12597,#12598,#12599,#12600));
#3678=EDGE_LOOP('',(#12601,#12602,#12603,#12604,#12605,#12606));
#3679=EDGE_LOOP('',(#12607,#12608,#12609,#12610,#12611,#12612));
#3680=EDGE_LOOP('',(#12613,#12614,#12615,#12616,#12617,#12618));
#3681=EDGE_LOOP('',(#12619,#12620,#12621,#12622,#12623,#12624));
#3682=EDGE_LOOP('',(#12625,#12626,#12627,#12628,#12629,#12630));
#3683=EDGE_LOOP('',(#12631,#12632,#12633,#12634,#12635,#12636));
#3684=EDGE_LOOP('',(#12637,#12638,#12639,#12640,#12641,#12642));
#3685=EDGE_LOOP('',(#12643,#12644,#12645,#12646));
#3686=EDGE_LOOP('',(#12647,#12648,#12649,#12650));
#3687=EDGE_LOOP('',(#12651,#12652,#12653,#12654));
#3688=EDGE_LOOP('',(#12655,#12656,#12657,#12658));
#3689=EDGE_LOOP('',(#12659,#12660,#12661,#12662));
#3690=EDGE_LOOP('',(#12663,#12664,#12665,#12666));
#3691=EDGE_LOOP('',(#12667,#12668,#12669,#12670));
#3692=EDGE_LOOP('',(#12671,#12672,#12673,#12674));
#3693=EDGE_LOOP('',(#12675,#12676,#12677,#12678,#12679,#12680));
#3694=EDGE_LOOP('',(#12681,#12682,#12683,#12684,#12685,#12686));
#3695=EDGE_LOOP('',(#12687,#12688,#12689,#12690));
#3696=EDGE_LOOP('',(#12691,#12692,#12693,#12694,#12695));
#3697=EDGE_LOOP('',(#12696,#12697,#12698,#12699,#12700,#12701));
#3698=EDGE_LOOP('',(#12702,#12703,#12704,#12705));
#3699=EDGE_LOOP('',(#12706,#12707,#12708,#12709,#12710));
#3700=EDGE_LOOP('',(#12711,#12712,#12713,#12714,#12715));
#3701=EDGE_LOOP('',(#12716,#12717,#12718,#12719,#12720,#12721));
#3702=EDGE_LOOP('',(#12722,#12723,#12724,#12725));
#3703=EDGE_LOOP('',(#12726,#12727,#12728,#12729,#12730));
#3704=EDGE_LOOP('',(#12731,#12732,#12733,#12734,#12735));
#3705=EDGE_LOOP('',(#12736,#12737,#12738,#12739,#12740,#12741));
#3706=EDGE_LOOP('',(#12742,#12743,#12744,#12745));
#3707=EDGE_LOOP('',(#12746,#12747,#12748,#12749,#12750));
#3708=EDGE_LOOP('',(#12751,#12752,#12753,#12754,#12755));
#3709=EDGE_LOOP('',(#12756,#12757,#12758,#12759,#12760,#12761));
#3710=EDGE_LOOP('',(#12762,#12763,#12764,#12765));
#3711=EDGE_LOOP('',(#12766,#12767,#12768,#12769,#12770));
#3712=EDGE_LOOP('',(#12771,#12772,#12773,#12774,#12775));
#3713=EDGE_LOOP('',(#12776,#12777,#12778,#12779,#12780,#12781));
#3714=EDGE_LOOP('',(#12782,#12783,#12784,#12785));
#3715=EDGE_LOOP('',(#12786,#12787,#12788,#12789,#12790));
#3716=EDGE_LOOP('',(#12791,#12792,#12793,#12794,#12795));
#3717=EDGE_LOOP('',(#12796,#12797,#12798,#12799,#12800,#12801));
#3718=EDGE_LOOP('',(#12802,#12803,#12804,#12805));
#3719=EDGE_LOOP('',(#12806,#12807,#12808,#12809,#12810));
#3720=EDGE_LOOP('',(#12811,#12812,#12813,#12814,#12815));
#3721=EDGE_LOOP('',(#12816,#12817,#12818,#12819,#12820,#12821));
#3722=EDGE_LOOP('',(#12822,#12823,#12824,#12825));
#3723=EDGE_LOOP('',(#12826,#12827,#12828,#12829,#12830));
#3724=EDGE_LOOP('',(#12831,#12832,#12833,#12834,#12835));
#3725=EDGE_LOOP('',(#12836,#12837,#12838,#12839,#12840,#12841));
#3726=EDGE_LOOP('',(#12842,#12843,#12844,#12845));
#3727=EDGE_LOOP('',(#12846,#12847,#12848,#12849));
#3728=EDGE_LOOP('',(#12850,#12851,#12852,#12853));
#3729=EDGE_LOOP('',(#12854,#12855,#12856,#12857,#12858,#12859));
#3730=EDGE_LOOP('',(#12860,#12861,#12862,#12863,#12864));
#3731=EDGE_LOOP('',(#12865,#12866,#12867,#12868));
#3732=EDGE_LOOP('',(#12869,#12870,#12871,#12872,#12873,#12874));
#3733=EDGE_LOOP('',(#12875,#12876,#12877,#12878));
#3734=EDGE_LOOP('',(#12879,#12880,#12881,#12882));
#3735=EDGE_LOOP('',(#12883,#12884,#12885,#12886,#12887,#12888));
#3736=EDGE_LOOP('',(#12889,#12890,#12891,#12892,#12893,#12894));
#3737=EDGE_LOOP('',(#12895,#12896,#12897,#12898,#12899,#12900));
#3738=EDGE_LOOP('',(#12901,#12902,#12903,#12904,#12905,#12906));
#3739=EDGE_LOOP('',(#12907,#12908,#12909,#12910,#12911,#12912));
#3740=EDGE_LOOP('',(#12913,#12914,#12915,#12916,#12917,#12918));
#3741=EDGE_LOOP('',(#12919,#12920,#12921,#12922,#12923,#12924));
#3742=EDGE_LOOP('',(#12925,#12926,#12927,#12928,#12929,#12930));
#3743=EDGE_LOOP('',(#12931,#12932,#12933,#12934));
#3744=EDGE_LOOP('',(#12935,#12936,#12937,#12938));
#3745=EDGE_LOOP('',(#12939,#12940,#12941,#12942));
#3746=EDGE_LOOP('',(#12943,#12944,#12945,#12946));
#3747=EDGE_LOOP('',(#12947,#12948,#12949,#12950));
#3748=EDGE_LOOP('',(#12951,#12952,#12953,#12954));
#3749=EDGE_LOOP('',(#12955,#12956,#12957,#12958));
#3750=EDGE_LOOP('',(#12959,#12960,#12961,#12962));
#3751=EDGE_LOOP('',(#12963,#12964,#12965,#12966));
#3752=EDGE_LOOP('',(#12967,#12968,#12969,#12970,#12971,#12972));
#3753=EDGE_LOOP('',(#12973,#12974,#12975,#12976,#12977));
#3754=EDGE_LOOP('',(#12978,#12979,#12980,#12981,#12982,#12983));
#3755=EDGE_LOOP('',(#12984,#12985,#12986,#12987));
#3756=EDGE_LOOP('',(#12988,#12989,#12990,#12991,#12992));
#3757=EDGE_LOOP('',(#12993,#12994,#12995,#12996,#12997));
#3758=EDGE_LOOP('',(#12998,#12999,#13000,#13001,#13002,#13003));
#3759=EDGE_LOOP('',(#13004,#13005,#13006,#13007));
#3760=EDGE_LOOP('',(#13008,#13009,#13010,#13011,#13012));
#3761=EDGE_LOOP('',(#13013,#13014,#13015,#13016,#13017));
#3762=EDGE_LOOP('',(#13018,#13019,#13020,#13021,#13022,#13023));
#3763=EDGE_LOOP('',(#13024,#13025,#13026,#13027));
#3764=EDGE_LOOP('',(#13028,#13029,#13030,#13031,#13032));
#3765=EDGE_LOOP('',(#13033,#13034,#13035,#13036,#13037));
#3766=EDGE_LOOP('',(#13038,#13039,#13040,#13041,#13042,#13043));
#3767=EDGE_LOOP('',(#13044,#13045,#13046,#13047));
#3768=EDGE_LOOP('',(#13048,#13049,#13050,#13051,#13052));
#3769=EDGE_LOOP('',(#13053,#13054,#13055,#13056,#13057));
#3770=EDGE_LOOP('',(#13058,#13059,#13060,#13061,#13062,#13063));
#3771=EDGE_LOOP('',(#13064,#13065,#13066,#13067));
#3772=EDGE_LOOP('',(#13068,#13069,#13070,#13071,#13072));
#3773=EDGE_LOOP('',(#13073,#13074,#13075,#13076,#13077));
#3774=EDGE_LOOP('',(#13078,#13079,#13080,#13081,#13082,#13083));
#3775=EDGE_LOOP('',(#13084,#13085,#13086,#13087));
#3776=EDGE_LOOP('',(#13088,#13089,#13090,#13091,#13092));
#3777=EDGE_LOOP('',(#13093,#13094,#13095,#13096,#13097));
#3778=EDGE_LOOP('',(#13098,#13099,#13100,#13101,#13102,#13103));
#3779=EDGE_LOOP('',(#13104,#13105,#13106,#13107));
#3780=EDGE_LOOP('',(#13108,#13109,#13110,#13111,#13112));
#3781=EDGE_LOOP('',(#13113,#13114,#13115,#13116,#13117));
#3782=EDGE_LOOP('',(#13118,#13119,#13120,#13121,#13122,#13123));
#3783=EDGE_LOOP('',(#13124,#13125,#13126,#13127));
#3784=EDGE_LOOP('',(#13128,#13129,#13130,#13131,#13132));
#3785=EDGE_LOOP('',(#13133,#13134,#13135,#13136,#13137));
#3786=EDGE_LOOP('',(#13138,#13139,#13140,#13141,#13142,#13143));
#3787=EDGE_LOOP('',(#13144,#13145,#13146,#13147));
#3788=EDGE_LOOP('',(#13148,#13149,#13150,#13151,#13152));
#3789=EDGE_LOOP('',(#13153,#13154,#13155,#13156));
#3790=EDGE_LOOP('',(#13157,#13158,#13159,#13160,#13161,#13162));
#3791=EDGE_LOOP('',(#13163,#13164,#13165,#13166,#13167));
#3792=EDGE_LOOP('',(#13168,#13169,#13170,#13171,#13172,#13173));
#3793=EDGE_LOOP('',(#13174,#13175,#13176,#13177,#13178,#13179));
#3794=EDGE_LOOP('',(#13180,#13181,#13182,#13183,#13184,#13185));
#3795=EDGE_LOOP('',(#13186,#13187,#13188,#13189,#13190,#13191));
#3796=EDGE_LOOP('',(#13192,#13193,#13194,#13195,#13196,#13197));
#3797=EDGE_LOOP('',(#13198,#13199,#13200,#13201,#13202,#13203));
#3798=EDGE_LOOP('',(#13204,#13205,#13206,#13207,#13208,#13209));
#3799=EDGE_LOOP('',(#13210,#13211,#13212,#13213,#13214,#13215));
#3800=EDGE_LOOP('',(#13216,#13217,#13218,#13219));
#3801=EDGE_LOOP('',(#13220,#13221,#13222,#13223));
#3802=EDGE_LOOP('',(#13224,#13225,#13226,#13227));
#3803=EDGE_LOOP('',(#13228,#13229,#13230,#13231));
#3804=EDGE_LOOP('',(#13232,#13233,#13234,#13235));
#3805=EDGE_LOOP('',(#13236,#13237,#13238,#13239));
#3806=EDGE_LOOP('',(#13240,#13241,#13242,#13243));
#3807=EDGE_LOOP('',(#13244,#13245,#13246,#13247));
#3808=EDGE_LOOP('',(#13248,#13249,#13250,#13251));
#3809=EDGE_LOOP('',(#13252,#13253,#13254,#13255));
#3810=EDGE_LOOP('',(#13256,#13257,#13258,#13259));
#3811=EDGE_LOOP('',(#13260,#13261,#13262,#13263,#13264,#13265));
#3812=EDGE_LOOP('',(#13266,#13267,#13268,#13269,#13270,#13271));
#3813=EDGE_LOOP('',(#13272,#13273,#13274,#13275,#13276,#13277));
#3814=EDGE_LOOP('',(#13278,#13279,#13280,#13281,#13282,#13283));
#3815=EDGE_LOOP('',(#13284,#13285,#13286,#13287,#13288,#13289));
#3816=EDGE_LOOP('',(#13290,#13291,#13292,#13293,#13294,#13295));
#3817=EDGE_LOOP('',(#13296,#13297,#13298,#13299,#13300,#13301));
#3818=EDGE_LOOP('',(#13302,#13303,#13304,#13305,#13306,#13307));
#3819=EDGE_LOOP('',(#13308,#13309,#13310,#13311));
#3820=EDGE_LOOP('',(#13312,#13313,#13314,#13315));
#3821=EDGE_LOOP('',(#13316,#13317,#13318,#13319));
#3822=EDGE_LOOP('',(#13320,#13321,#13322,#13323));
#3823=EDGE_LOOP('',(#13324,#13325,#13326,#13327));
#3824=EDGE_LOOP('',(#13328,#13329,#13330,#13331));
#3825=EDGE_LOOP('',(#13332,#13333,#13334,#13335));
#3826=EDGE_LOOP('',(#13336,#13337,#13338,#13339));
#3827=EDGE_LOOP('',(#13340,#13341,#13342,#13343));
#3828=EDGE_LOOP('',(#13344,#13345,#13346,#13347));
#3829=EDGE_LOOP('',(#13348,#13349,#13350,#13351,#13352,#13353));
#3830=EDGE_LOOP('',(#13354,#13355,#13356,#13357));
#3831=EDGE_LOOP('',(#13358,#13359,#13360,#13361,#13362,#13363));
#3832=EDGE_LOOP('',(#13364,#13365,#13366,#13367));
#3833=EDGE_LOOP('',(#13368,#13369,#13370,#13371,#13372,#13373));
#3834=EDGE_LOOP('',(#13374,#13375,#13376,#13377));
#3835=EDGE_LOOP('',(#13378,#13379,#13380,#13381,#13382,#13383));
#3836=EDGE_LOOP('',(#13384,#13385,#13386,#13387));
#3837=EDGE_LOOP('',(#13388,#13389,#13390,#13391,#13392,#13393));
#3838=EDGE_LOOP('',(#13394,#13395,#13396,#13397));
#3839=EDGE_LOOP('',(#13398,#13399,#13400,#13401,#13402,#13403));
#3840=EDGE_LOOP('',(#13404,#13405,#13406,#13407));
#3841=EDGE_LOOP('',(#13408,#13409,#13410,#13411,#13412,#13413));
#3842=EDGE_LOOP('',(#13414,#13415,#13416,#13417));
#3843=EDGE_LOOP('',(#13418,#13419,#13420,#13421,#13422,#13423));
#3844=EDGE_LOOP('',(#13424,#13425,#13426,#13427));
#3845=EDGE_LOOP('',(#13428,#13429,#13430,#13431,#13432,#13433));
#3846=EDGE_LOOP('',(#13434,#13435,#13436,#13437));
#3847=EDGE_LOOP('',(#13438,#13439,#13440,#13441,#13442,#13443));
#3848=EDGE_LOOP('',(#13444,#13445,#13446,#13447));
#3849=EDGE_LOOP('',(#13448,#13449,#13450,#13451,#13452,#13453));
#3850=EDGE_LOOP('',(#13454,#13455,#13456,#13457));
#3851=EDGE_LOOP('',(#13458,#13459,#13460,#13461,#13462,#13463));
#3852=EDGE_LOOP('',(#13464,#13465,#13466,#13467));
#3853=EDGE_LOOP('',(#13468,#13469,#13470,#13471));
#3854=EDGE_LOOP('',(#13472));
#3855=EDGE_LOOP('',(#13473));
#3856=EDGE_LOOP('',(#13474,#13475,#13476,#13477,#13478,#13479,#13480,#13481,
#13482,#13483,#13484,#13485,#13486,#13487,#13488,#13489,#13490,#13491,#13492,
#13493,#13494,#13495,#13496,#13497,#13498,#13499,#13500,#13501,#13502,#13503,
#13504,#13505,#13506,#13507,#13508,#13509,#13510,#13511,#13512,#13513,#13514,
#13515,#13516,#13517,#13518,#13519,#13520,#13521,#13522,#13523,#13524,#13525,
#13526,#13527,#13528,#13529,#13530,#13531,#13532,#13533,#13534,#13535,#13536,
#13537,#13538,#13539,#13540,#13541,#13542,#13543,#13544,#13545,#13546,#13547,
#13548,#13549,#13550,#13551,#13552,#13553,#13554,#13555,#13556,#13557,#13558,
#13559,#13560,#13561,#13562,#13563,#13564,#13565,#13566,#13567,#13568,#13569,
#13570,#13571,#13572,#13573,#13574,#13575,#13576,#13577,#13578,#13579,#13580,
#13581,#13582,#13583,#13584,#13585,#13586,#13587,#13588,#13589,#13590,#13591,
#13592,#13593,#13594,#13595,#13596,#13597,#13598,#13599,#13600,#13601,#13602,
#13603,#13604,#13605,#13606,#13607,#13608,#13609,#13610,#13611,#13612,#13613,
#13614,#13615,#13616,#13617,#13618,#13619,#13620,#13621,#13622,#13623,#13624,
#13625,#13626,#13627,#13628,#13629,#13630,#13631,#13632,#13633,#13634,#13635,
#13636,#13637,#13638,#13639,#13640,#13641,#13642,#13643,#13644,#13645,#13646,
#13647,#13648,#13649,#13650,#13651,#13652,#13653,#13654,#13655,#13656,#13657));
#3857=EDGE_LOOP('',(#13658,#13659,#13660,#13661));
#3858=EDGE_LOOP('',(#13662));
#3859=EDGE_LOOP('',(#13663));
#3860=EDGE_LOOP('',(#13664));
#3861=EDGE_LOOP('',(#13665));
#3862=EDGE_LOOP('',(#13666));
#3863=EDGE_LOOP('',(#13667));
#3864=EDGE_LOOP('',(#13668));
#3865=EDGE_LOOP('',(#13669,#13670,#13671,#13672));
#3866=EDGE_LOOP('',(#13673,#13674,#13675,#13676));
#3867=EDGE_LOOP('',(#13677,#13678,#13679,#13680));
#3868=EDGE_LOOP('',(#13681,#13682,#13683,#13684));
#3869=EDGE_LOOP('',(#13685,#13686,#13687,#13688));
#3870=EDGE_LOOP('',(#13689,#13690,#13691,#13692));
#3871=EDGE_LOOP('',(#13693,#13694,#13695,#13696));
#3872=EDGE_LOOP('',(#13697,#13698,#13699,#13700));
#3873=EDGE_LOOP('',(#13701,#13702,#13703,#13704));
#3874=EDGE_LOOP('',(#13705,#13706,#13707,#13708));
#3875=EDGE_LOOP('',(#13709,#13710,#13711,#13712));
#3876=EDGE_LOOP('',(#13713,#13714,#13715,#13716));
#3877=EDGE_LOOP('',(#13717,#13718,#13719,#13720));
#3878=EDGE_LOOP('',(#13721,#13722,#13723,#13724));
#3879=EDGE_LOOP('',(#13725,#13726,#13727,#13728));
#3880=EDGE_LOOP('',(#13729,#13730,#13731,#13732));
#3881=EDGE_LOOP('',(#13733,#13734,#13735,#13736));
#3882=EDGE_LOOP('',(#13737,#13738,#13739,#13740));
#3883=EDGE_LOOP('',(#13741,#13742,#13743,#13744));
#3884=EDGE_LOOP('',(#13745,#13746,#13747,#13748));
#3885=EDGE_LOOP('',(#13749,#13750,#13751,#13752));
#3886=EDGE_LOOP('',(#13753,#13754,#13755,#13756));
#3887=EDGE_LOOP('',(#13757,#13758,#13759,#13760));
#3888=EDGE_LOOP('',(#13761,#13762,#13763,#13764));
#3889=EDGE_LOOP('',(#13765,#13766,#13767,#13768));
#3890=EDGE_LOOP('',(#13769,#13770,#13771,#13772));
#3891=EDGE_LOOP('',(#13773,#13774,#13775,#13776));
#3892=EDGE_LOOP('',(#13777,#13778,#13779,#13780,#13781,#13782));
#3893=EDGE_LOOP('',(#13783,#13784,#13785,#13786));
#3894=EDGE_LOOP('',(#13787,#13788,#13789,#13790));
#3895=EDGE_LOOP('',(#13791,#13792,#13793,#13794));
#3896=EDGE_LOOP('',(#13795,#13796,#13797,#13798));
#3897=EDGE_LOOP('',(#13799,#13800,#13801,#13802));
#3898=EDGE_LOOP('',(#13803,#13804,#13805,#13806));
#3899=EDGE_LOOP('',(#13807,#13808,#13809,#13810));
#3900=EDGE_LOOP('',(#13811,#13812,#13813,#13814));
#3901=EDGE_LOOP('',(#13815,#13816,#13817,#13818));
#3902=EDGE_LOOP('',(#13819,#13820,#13821,#13822));
#3903=EDGE_LOOP('',(#13823,#13824,#13825,#13826,#13827,#13828));
#3904=EDGE_LOOP('',(#13829,#13830,#13831,#13832));
#3905=EDGE_LOOP('',(#13833,#13834,#13835,#13836));
#3906=EDGE_LOOP('',(#13837,#13838,#13839,#13840));
#3907=EDGE_LOOP('',(#13841,#13842,#13843,#13844));
#3908=EDGE_LOOP('',(#13845,#13846,#13847,#13848));
#3909=EDGE_LOOP('',(#13849,#13850,#13851,#13852));
#3910=EDGE_LOOP('',(#13853,#13854,#13855,#13856));
#3911=EDGE_LOOP('',(#13857,#13858,#13859,#13860));
#3912=EDGE_LOOP('',(#13861,#13862,#13863,#13864));
#3913=EDGE_LOOP('',(#13865,#13866,#13867,#13868));
#3914=EDGE_LOOP('',(#13869,#13870,#13871,#13872,#13873,#13874));
#3915=EDGE_LOOP('',(#13875,#13876,#13877,#13878));
#3916=EDGE_LOOP('',(#13879,#13880,#13881,#13882));
#3917=EDGE_LOOP('',(#13883,#13884,#13885,#13886));
#3918=EDGE_LOOP('',(#13887,#13888,#13889,#13890));
#3919=EDGE_LOOP('',(#13891,#13892,#13893,#13894));
#3920=EDGE_LOOP('',(#13895,#13896,#13897,#13898));
#3921=EDGE_LOOP('',(#13899,#13900,#13901,#13902));
#3922=EDGE_LOOP('',(#13903,#13904,#13905,#13906));
#3923=EDGE_LOOP('',(#13907,#13908,#13909,#13910));
#3924=EDGE_LOOP('',(#13911,#13912,#13913,#13914));
#3925=EDGE_LOOP('',(#13915,#13916,#13917,#13918));
#3926=EDGE_LOOP('',(#13919,#13920,#13921,#13922));
#3927=EDGE_LOOP('',(#13923,#13924,#13925,#13926));
#3928=EDGE_LOOP('',(#13927,#13928,#13929,#13930));
#3929=EDGE_LOOP('',(#13931,#13932,#13933,#13934));
#3930=EDGE_LOOP('',(#13935,#13936,#13937,#13938));
#3931=EDGE_LOOP('',(#13939,#13940,#13941,#13942));
#3932=EDGE_LOOP('',(#13943,#13944,#13945,#13946));
#3933=EDGE_LOOP('',(#13947,#13948,#13949,#13950,#13951));
#3934=EDGE_LOOP('',(#13952,#13953,#13954,#13955));
#3935=EDGE_LOOP('',(#13956,#13957,#13958,#13959));
#3936=EDGE_LOOP('',(#13960,#13961,#13962,#13963));
#3937=EDGE_LOOP('',(#13964,#13965,#13966,#13967));
#3938=EDGE_LOOP('',(#13968,#13969,#13970,#13971));
#3939=EDGE_LOOP('',(#13972,#13973,#13974,#13975));
#3940=EDGE_LOOP('',(#13976,#13977,#13978,#13979));
#3941=EDGE_LOOP('',(#13980,#13981,#13982,#13983));
#3942=EDGE_LOOP('',(#13984,#13985,#13986,#13987));
#3943=EDGE_LOOP('',(#13988,#13989,#13990,#13991));
#3944=EDGE_LOOP('',(#13992,#13993,#13994,#13995));
#3945=EDGE_LOOP('',(#13996,#13997,#13998,#13999));
#3946=EDGE_LOOP('',(#14000,#14001,#14002,#14003));
#3947=EDGE_LOOP('',(#14004,#14005,#14006,#14007));
#3948=EDGE_LOOP('',(#14008,#14009,#14010,#14011));
#3949=EDGE_LOOP('',(#14012,#14013,#14014,#14015));
#3950=EDGE_LOOP('',(#14016,#14017,#14018,#14019));
#3951=EDGE_LOOP('',(#14020,#14021,#14022,#14023));
#3952=EDGE_LOOP('',(#14024,#14025,#14026,#14027));
#3953=EDGE_LOOP('',(#14028,#14029,#14030,#14031));
#3954=EDGE_LOOP('',(#14032,#14033,#14034,#14035));
#3955=EDGE_LOOP('',(#14036,#14037,#14038,#14039));
#3956=EDGE_LOOP('',(#14040,#14041,#14042,#14043,#14044,#14045));
#3957=EDGE_LOOP('',(#14046,#14047,#14048,#14049));
#3958=EDGE_LOOP('',(#14050,#14051,#14052,#14053));
#3959=EDGE_LOOP('',(#14054,#14055,#14056,#14057));
#3960=EDGE_LOOP('',(#14058,#14059,#14060,#14061));
#3961=EDGE_LOOP('',(#14062,#14063,#14064,#14065));
#3962=EDGE_LOOP('',(#14066,#14067,#14068,#14069));
#3963=EDGE_LOOP('',(#14070,#14071,#14072,#14073));
#3964=EDGE_LOOP('',(#14074,#14075,#14076,#14077));
#3965=EDGE_LOOP('',(#14078,#14079,#14080,#14081));
#3966=EDGE_LOOP('',(#14082,#14083,#14084,#14085,#14086,#14087));
#3967=EDGE_LOOP('',(#14088,#14089,#14090,#14091));
#3968=EDGE_LOOP('',(#14092,#14093,#14094,#14095));
#3969=EDGE_LOOP('',(#14096,#14097,#14098,#14099));
#3970=EDGE_LOOP('',(#14100,#14101,#14102,#14103));
#3971=EDGE_LOOP('',(#14104,#14105,#14106,#14107));
#3972=EDGE_LOOP('',(#14108,#14109,#14110,#14111));
#3973=EDGE_LOOP('',(#14112,#14113,#14114,#14115));
#3974=EDGE_LOOP('',(#14116,#14117,#14118,#14119));
#3975=EDGE_LOOP('',(#14120,#14121,#14122,#14123));
#3976=EDGE_LOOP('',(#14124,#14125,#14126,#14127));
#3977=EDGE_LOOP('',(#14128,#14129,#14130,#14131,#14132,#14133));
#3978=EDGE_LOOP('',(#14134,#14135,#14136,#14137));
#3979=EDGE_LOOP('',(#14138,#14139,#14140,#14141));
#3980=EDGE_LOOP('',(#14142,#14143,#14144,#14145));
#3981=EDGE_LOOP('',(#14146,#14147,#14148,#14149));
#3982=EDGE_LOOP('',(#14150,#14151,#14152));
#3983=EDGE_LOOP('',(#14153,#14154,#14155));
#3984=EDGE_LOOP('',(#14156,#14157,#14158));
#3985=EDGE_LOOP('',(#14159,#14160,#14161));
#3986=EDGE_LOOP('',(#14162,#14163,#14164));
#3987=EDGE_LOOP('',(#14165,#14166,#14167,#14168));
#3988=EDGE_LOOP('',(#14169));
#3989=EDGE_LOOP('',(#14170));
#3990=EDGE_LOOP('',(#14171));
#3991=EDGE_LOOP('',(#14172));
#3992=EDGE_LOOP('',(#14173));
#3993=EDGE_LOOP('',(#14174));
#3994=EDGE_LOOP('',(#14175));
#3995=EDGE_LOOP('',(#14176));
#3996=EDGE_LOOP('',(#14177));
#3997=EDGE_LOOP('',(#14178));
#3998=EDGE_LOOP('',(#14179));
#3999=EDGE_LOOP('',(#14180));
#4415=LINE('',#24001,#5390);
#4416=LINE('',#24003,#5391);
#4417=LINE('',#24004,#5392);
#4418=LINE('',#24009,#5393);
#4419=LINE('',#24034,#5394);
#4420=LINE('',#24036,#5395);
#4421=LINE('',#24038,#5396);
#4422=LINE('',#24046,#5397);
#4423=LINE('',#24066,#5398);
#4424=LINE('',#24067,#5399);
#4425=LINE('',#24077,#5400);
#4426=LINE('',#24086,#5401);
#4427=LINE('',#24088,#5402);
#4428=LINE('',#24090,#5403);
#4429=LINE('',#24115,#5404);
#4430=LINE('',#24119,#5405);
#4431=LINE('',#24121,#5406);
#4432=LINE('',#24130,#5407);
#4433=LINE('',#24148,#5408);
#4434=LINE('',#24150,#5409);
#4435=LINE('',#24152,#5410);
#4436=LINE('',#24177,#5411);
#4437=LINE('',#24180,#5412);
#4438=LINE('',#24182,#5413);
#4439=LINE('',#24188,#5414);
#4440=LINE('',#24190,#5415);
#4441=LINE('',#24197,#5416);
#4442=LINE('',#24199,#5417);
#4443=LINE('',#24204,#5418);
#4444=LINE('',#24219,#5419);
#4445=LINE('',#24242,#5420);
#4446=LINE('',#24244,#5421);
#4447=LINE('',#24246,#5422);
#4448=LINE('',#24254,#5423);
#4449=LINE('',#24276,#5424);
#4450=LINE('',#24278,#5425);
#4451=LINE('',#24287,#5426);
#4452=LINE('',#24309,#5427);
#4453=LINE('',#24312,#5428);
#4454=LINE('',#24314,#5429);
#4455=LINE('',#24321,#5430);
#4456=LINE('',#24323,#5431);
#4457=LINE('',#24332,#5432);
#4458=LINE('',#24354,#5433);
#4459=LINE('',#24357,#5434);
#4460=LINE('',#24359,#5435);
#4461=LINE('',#24366,#5436);
#4462=LINE('',#24368,#5437);
#4463=LINE('',#24377,#5438);
#4464=LINE('',#24399,#5439);
#4465=LINE('',#24402,#5440);
#4466=LINE('',#24404,#5441);
#4467=LINE('',#24411,#5442);
#4468=LINE('',#24413,#5443);
#4469=LINE('',#24422,#5444);
#4470=LINE('',#24444,#5445);
#4471=LINE('',#24447,#5446);
#4472=LINE('',#24449,#5447);
#4473=LINE('',#24456,#5448);
#4474=LINE('',#24458,#5449);
#4475=LINE('',#24467,#5450);
#4476=LINE('',#24489,#5451);
#4477=LINE('',#24492,#5452);
#4478=LINE('',#24494,#5453);
#4479=LINE('',#24501,#5454);
#4480=LINE('',#24503,#5455);
#4481=LINE('',#24512,#5456);
#4482=LINE('',#24534,#5457);
#4483=LINE('',#24537,#5458);
#4484=LINE('',#24539,#5459);
#4485=LINE('',#24546,#5460);
#4486=LINE('',#24548,#5461);
#4487=LINE('',#24557,#5462);
#4488=LINE('',#24579,#5463);
#4489=LINE('',#24582,#5464);
#4490=LINE('',#24584,#5465);
#4491=LINE('',#24591,#5466);
#4492=LINE('',#24593,#5467);
#4493=LINE('',#24602,#5468);
#4494=LINE('',#24624,#5469);
#4495=LINE('',#24627,#5470);
#4496=LINE('',#24629,#5471);
#4497=LINE('',#24978,#5472);
#4498=LINE('',#24982,#5473);
#4499=LINE('',#24989,#5474);
#4500=LINE('',#24990,#5475);
#4501=LINE('',#24998,#5476);
#4502=LINE('',#25000,#5477);
#4503=LINE('',#25002,#5478);
#4504=LINE('',#25024,#5479);
#4505=LINE('',#25027,#5480);
#4506=LINE('',#25029,#5481);
#4507=LINE('',#25040,#5482);
#4508=LINE('',#25042,#5483);
#4509=LINE('',#25044,#5484);
#4510=LINE('',#25066,#5485);
#4511=LINE('',#25069,#5486);
#4512=LINE('',#25071,#5487);
#4513=LINE('',#25082,#5488);
#4514=LINE('',#25084,#5489);
#4515=LINE('',#25086,#5490);
#4516=LINE('',#25108,#5491);
#4517=LINE('',#25115,#5492);
#4518=LINE('',#25116,#5493);
#4519=LINE('',#25121,#5494);
#4520=LINE('',#25128,#5495);
#4521=LINE('',#25132,#5496);
#4522=LINE('',#25134,#5497);
#4523=LINE('',#25139,#5498);
#4524=LINE('',#25158,#5499);
#4525=LINE('',#25161,#5500);
#4526=LINE('',#25163,#5501);
#4527=LINE('',#25170,#5502);
#4528=LINE('',#25172,#5503);
#4529=LINE('',#25181,#5504);
#4530=LINE('',#25200,#5505);
#4531=LINE('',#25203,#5506);
#4532=LINE('',#25205,#5507);
#4533=LINE('',#25212,#5508);
#4534=LINE('',#25214,#5509);
#4535=LINE('',#25223,#5510);
#4536=LINE('',#25242,#5511);
#4537=LINE('',#25245,#5512);
#4538=LINE('',#25247,#5513);
#4539=LINE('',#25254,#5514);
#4540=LINE('',#25256,#5515);
#4541=LINE('',#25265,#5516);
#4542=LINE('',#25284,#5517);
#4543=LINE('',#25287,#5518);
#4544=LINE('',#25289,#5519);
#4545=LINE('',#25296,#5520);
#4546=LINE('',#25298,#5521);
#4547=LINE('',#25307,#5522);
#4548=LINE('',#25326,#5523);
#4549=LINE('',#25329,#5524);
#4550=LINE('',#25331,#5525);
#4551=LINE('',#25338,#5526);
#4552=LINE('',#25340,#5527);
#4553=LINE('',#25349,#5528);
#4554=LINE('',#25368,#5529);
#4555=LINE('',#25372,#5530);
#4556=LINE('',#25374,#5531);
#4557=LINE('',#25376,#5532);
#4558=LINE('',#25399,#5533);
#4559=LINE('',#25400,#5534);
#4560=LINE('',#25430,#5535);
#4561=LINE('',#25432,#5536);
#4562=LINE('',#25434,#5537);
#4563=LINE('',#25456,#5538);
#4564=LINE('',#25459,#5539);
#4565=LINE('',#25461,#5540);
#4566=LINE('',#25478,#5541);
#4567=LINE('',#25480,#5542);
#4568=LINE('',#25482,#5543);
#4569=LINE('',#25500,#5544);
#4570=LINE('',#25503,#5545);
#4571=LINE('',#25505,#5546);
#4572=LINE('',#25516,#5547);
#4573=LINE('',#25518,#5548);
#4574=LINE('',#25520,#5549);
#4575=LINE('',#25542,#5550);
#4576=LINE('',#25545,#5551);
#4577=LINE('',#25547,#5552);
#4578=LINE('',#25558,#5553);
#4579=LINE('',#25560,#5554);
#4580=LINE('',#25562,#5555);
#4581=LINE('',#25584,#5556);
#4582=LINE('',#25592,#5557);
#4583=LINE('',#25594,#5558);
#4584=LINE('',#25595,#5559);
#4585=LINE('',#25600,#5560);
#4586=LINE('',#25611,#5561);
#4587=LINE('',#25615,#5562);
#4588=LINE('',#25617,#5563);
#4589=LINE('',#25622,#5564);
#4590=LINE('',#25641,#5565);
#4591=LINE('',#25644,#5566);
#4592=LINE('',#25646,#5567);
#4593=LINE('',#25653,#5568);
#4594=LINE('',#25655,#5569);
#4595=LINE('',#25664,#5570);
#4596=LINE('',#25683,#5571);
#4597=LINE('',#25686,#5572);
#4598=LINE('',#25688,#5573);
#4599=LINE('',#25695,#5574);
#4600=LINE('',#25697,#5575);
#4601=LINE('',#25706,#5576);
#4602=LINE('',#25725,#5577);
#4603=LINE('',#25728,#5578);
#4604=LINE('',#25730,#5579);
#4605=LINE('',#25737,#5580);
#4606=LINE('',#25739,#5581);
#4607=LINE('',#25748,#5582);
#4608=LINE('',#25767,#5583);
#4609=LINE('',#25770,#5584);
#4610=LINE('',#25772,#5585);
#4611=LINE('',#25779,#5586);
#4612=LINE('',#25781,#5587);
#4613=LINE('',#25790,#5588);
#4614=LINE('',#25809,#5589);
#4615=LINE('',#25813,#5590);
#4616=LINE('',#25815,#5591);
#4617=LINE('',#25817,#5592);
#4618=LINE('',#25842,#5593);
#4619=LINE('',#25843,#5594);
#4620=LINE('',#25869,#5595);
#4621=LINE('',#25871,#5596);
#4622=LINE('',#25873,#5597);
#4623=LINE('',#25895,#5598);
#4624=LINE('',#25898,#5599);
#4625=LINE('',#25900,#5600);
#4626=LINE('',#25911,#5601);
#4627=LINE('',#25913,#5602);
#4628=LINE('',#25915,#5603);
#4629=LINE('',#25937,#5604);
#4630=LINE('',#25940,#5605);
#4631=LINE('',#25942,#5606);
#4632=LINE('',#25953,#5607);
#4633=LINE('',#25955,#5608);
#4634=LINE('',#25957,#5609);
#4635=LINE('',#25979,#5610);
#4636=LINE('',#25982,#5611);
#4637=LINE('',#25984,#5612);
#4638=LINE('',#25995,#5613);
#4639=LINE('',#25997,#5614);
#4640=LINE('',#25999,#5615);
#4641=LINE('',#26021,#5616);
#4642=LINE('',#26024,#5617);
#4643=LINE('',#26026,#5618);
#4644=LINE('',#26037,#5619);
#4645=LINE('',#26039,#5620);
#4646=LINE('',#26041,#5621);
#4647=LINE('',#26063,#5622);
#4648=LINE('',#26071,#5623);
#4649=LINE('',#26073,#5624);
#4650=LINE('',#26074,#5625);
#4651=LINE('',#26079,#5626);
#4652=LINE('',#26090,#5627);
#4653=LINE('',#26094,#5628);
#4654=LINE('',#26096,#5629);
#4655=LINE('',#26101,#5630);
#4656=LINE('',#26120,#5631);
#4657=LINE('',#26123,#5632);
#4658=LINE('',#26125,#5633);
#4659=LINE('',#26132,#5634);
#4660=LINE('',#26134,#5635);
#4661=LINE('',#26143,#5636);
#4662=LINE('',#26162,#5637);
#4663=LINE('',#26165,#5638);
#4664=LINE('',#26167,#5639);
#4665=LINE('',#26174,#5640);
#4666=LINE('',#26176,#5641);
#4667=LINE('',#26185,#5642);
#4668=LINE('',#26204,#5643);
#4669=LINE('',#26207,#5644);
#4670=LINE('',#26209,#5645);
#4671=LINE('',#26216,#5646);
#4672=LINE('',#26218,#5647);
#4673=LINE('',#26227,#5648);
#4674=LINE('',#26246,#5649);
#4675=LINE('',#26250,#5650);
#4676=LINE('',#26252,#5651);
#4677=LINE('',#26254,#5652);
#4678=LINE('',#26285,#5653);
#4679=LINE('',#26286,#5654);
#4680=LINE('',#26308,#5655);
#4681=LINE('',#26310,#5656);
#4682=LINE('',#26312,#5657);
#4683=LINE('',#26334,#5658);
#4684=LINE('',#26337,#5659);
#4685=LINE('',#26339,#5660);
#4686=LINE('',#26356,#5661);
#4687=LINE('',#26358,#5662);
#4688=LINE('',#26360,#5663);
#4689=LINE('',#26378,#5664);
#4690=LINE('',#26381,#5665);
#4691=LINE('',#26383,#5666);
#4692=LINE('',#26394,#5667);
#4693=LINE('',#26396,#5668);
#4694=LINE('',#26398,#5669);
#4695=LINE('',#26420,#5670);
#4696=LINE('',#26423,#5671);
#4697=LINE('',#26425,#5672);
#4698=LINE('',#26436,#5673);
#4699=LINE('',#26438,#5674);
#4700=LINE('',#26440,#5675);
#4701=LINE('',#26462,#5676);
#4702=LINE('',#26465,#5677);
#4703=LINE('',#26467,#5678);
#4704=LINE('',#26478,#5679);
#4705=LINE('',#26480,#5680);
#4706=LINE('',#26482,#5681);
#4707=LINE('',#26504,#5682);
#4708=LINE('',#26507,#5683);
#4709=LINE('',#26509,#5684);
#4710=LINE('',#26520,#5685);
#4711=LINE('',#26522,#5686);
#4712=LINE('',#26524,#5687);
#4713=LINE('',#26546,#5688);
#4714=LINE('',#26554,#5689);
#4715=LINE('',#26556,#5690);
#4716=LINE('',#26557,#5691);
#4717=LINE('',#26562,#5692);
#4718=LINE('',#26573,#5693);
#4719=LINE('',#26577,#5694);
#4720=LINE('',#26579,#5695);
#4721=LINE('',#26584,#5696);
#4722=LINE('',#26603,#5697);
#4723=LINE('',#26606,#5698);
#4724=LINE('',#26608,#5699);
#4725=LINE('',#26615,#5700);
#4726=LINE('',#26617,#5701);
#4727=LINE('',#26626,#5702);
#4728=LINE('',#26645,#5703);
#4729=LINE('',#26648,#5704);
#4730=LINE('',#26650,#5705);
#4731=LINE('',#26657,#5706);
#4732=LINE('',#26659,#5707);
#4733=LINE('',#26668,#5708);
#4734=LINE('',#26687,#5709);
#4735=LINE('',#26691,#5710);
#4736=LINE('',#26693,#5711);
#4737=LINE('',#26695,#5712);
#4738=LINE('',#26728,#5713);
#4739=LINE('',#26729,#5714);
#4740=LINE('',#26747,#5715);
#4741=LINE('',#26749,#5716);
#4742=LINE('',#26751,#5717);
#4743=LINE('',#26773,#5718);
#4744=LINE('',#26776,#5719);
#4745=LINE('',#26778,#5720);
#4746=LINE('',#26789,#5721);
#4747=LINE('',#26791,#5722);
#4748=LINE('',#26793,#5723);
#4749=LINE('',#26815,#5724);
#4750=LINE('',#26818,#5725);
#4751=LINE('',#26820,#5726);
#4752=LINE('',#26831,#5727);
#4753=LINE('',#26833,#5728);
#4754=LINE('',#26835,#5729);
#4755=LINE('',#26857,#5730);
#4756=LINE('',#26860,#5731);
#4757=LINE('',#26862,#5732);
#4758=LINE('',#26873,#5733);
#4759=LINE('',#26875,#5734);
#4760=LINE('',#26877,#5735);
#4761=LINE('',#26899,#5736);
#4762=LINE('',#26902,#5737);
#4763=LINE('',#26904,#5738);
#4764=LINE('',#26915,#5739);
#4765=LINE('',#26917,#5740);
#4766=LINE('',#26919,#5741);
#4767=LINE('',#26941,#5742);
#4768=LINE('',#26944,#5743);
#4769=LINE('',#26946,#5744);
#4770=LINE('',#26957,#5745);
#4771=LINE('',#26959,#5746);
#4772=LINE('',#26961,#5747);
#4773=LINE('',#26983,#5748);
#4774=LINE('',#26986,#5749);
#4775=LINE('',#26988,#5750);
#4776=LINE('',#26999,#5751);
#4777=LINE('',#27001,#5752);
#4778=LINE('',#27003,#5753);
#4779=LINE('',#27025,#5754);
#4780=LINE('',#27033,#5755);
#4781=LINE('',#27035,#5756);
#4782=LINE('',#27036,#5757);
#4783=LINE('',#27041,#5758);
#4784=LINE('',#27052,#5759);
#4785=LINE('',#27056,#5760);
#4786=LINE('',#27058,#5761);
#4787=LINE('',#27063,#5762);
#4788=LINE('',#27082,#5763);
#4789=LINE('',#27085,#5764);
#4790=LINE('',#27087,#5765);
#4791=LINE('',#27094,#5766);
#4792=LINE('',#27096,#5767);
#4793=LINE('',#27105,#5768);
#4794=LINE('',#27124,#5769);
#4795=LINE('',#27128,#5770);
#4796=LINE('',#27130,#5771);
#4797=LINE('',#27132,#5772);
#4798=LINE('',#27171,#5773);
#4799=LINE('',#27172,#5774);
#4800=LINE('',#27186,#5775);
#4801=LINE('',#27188,#5776);
#4802=LINE('',#27190,#5777);
#4803=LINE('',#27212,#5778);
#4804=LINE('',#27215,#5779);
#4805=LINE('',#27217,#5780);
#4806=LINE('',#27228,#5781);
#4807=LINE('',#27230,#5782);
#4808=LINE('',#27232,#5783);
#4809=LINE('',#27254,#5784);
#4810=LINE('',#27257,#5785);
#4811=LINE('',#27259,#5786);
#4812=LINE('',#27270,#5787);
#4813=LINE('',#27272,#5788);
#4814=LINE('',#27274,#5789);
#4815=LINE('',#27296,#5790);
#4816=LINE('',#27299,#5791);
#4817=LINE('',#27301,#5792);
#4818=LINE('',#27312,#5793);
#4819=LINE('',#27314,#5794);
#4820=LINE('',#27316,#5795);
#4821=LINE('',#27338,#5796);
#4822=LINE('',#27341,#5797);
#4823=LINE('',#27343,#5798);
#4824=LINE('',#27354,#5799);
#4825=LINE('',#27356,#5800);
#4826=LINE('',#27358,#5801);
#4827=LINE('',#27380,#5802);
#4828=LINE('',#27383,#5803);
#4829=LINE('',#27385,#5804);
#4830=LINE('',#27396,#5805);
#4831=LINE('',#27398,#5806);
#4832=LINE('',#27400,#5807);
#4833=LINE('',#27422,#5808);
#4834=LINE('',#27425,#5809);
#4835=LINE('',#27427,#5810);
#4836=LINE('',#27438,#5811);
#4837=LINE('',#27440,#5812);
#4838=LINE('',#27442,#5813);
#4839=LINE('',#27464,#5814);
#4840=LINE('',#27467,#5815);
#4841=LINE('',#27469,#5816);
#4842=LINE('',#27480,#5817);
#4843=LINE('',#27482,#5818);
#4844=LINE('',#27484,#5819);
#4845=LINE('',#27506,#5820);
#4846=LINE('',#27514,#5821);
#4847=LINE('',#27516,#5822);
#4848=LINE('',#27517,#5823);
#4849=LINE('',#27522,#5824);
#4850=LINE('',#27533,#5825);
#4851=LINE('',#27537,#5826);
#4852=LINE('',#27539,#5827);
#4853=LINE('',#27544,#5828);
#4854=LINE('',#27563,#5829);
#4855=LINE('',#27567,#5830);
#4856=LINE('',#27569,#5831);
#4857=LINE('',#27571,#5832);
#4858=LINE('',#27614,#5833);
#4859=LINE('',#27615,#5834);
#4860=LINE('',#27621,#5835);
#4861=LINE('',#27623,#5836);
#4862=LINE('',#27627,#5837);
#4863=LINE('',#27642,#5838);
#4864=LINE('',#27645,#5839);
#4865=LINE('',#27647,#5840);
#4866=LINE('',#27654,#5841);
#4867=LINE('',#27656,#5842);
#4868=LINE('',#27665,#5843);
#4869=LINE('',#27684,#5844);
#4870=LINE('',#27687,#5845);
#4871=LINE('',#27689,#5846);
#4872=LINE('',#27696,#5847);
#4873=LINE('',#27698,#5848);
#4874=LINE('',#27707,#5849);
#4875=LINE('',#27726,#5850);
#4876=LINE('',#27729,#5851);
#4877=LINE('',#27731,#5852);
#4878=LINE('',#27738,#5853);
#4879=LINE('',#27740,#5854);
#4880=LINE('',#27749,#5855);
#4881=LINE('',#27768,#5856);
#4882=LINE('',#27771,#5857);
#4883=LINE('',#27773,#5858);
#4884=LINE('',#27780,#5859);
#4885=LINE('',#27782,#5860);
#4886=LINE('',#27791,#5861);
#4887=LINE('',#27810,#5862);
#4888=LINE('',#27813,#5863);
#4889=LINE('',#27815,#5864);
#4890=LINE('',#27822,#5865);
#4891=LINE('',#27824,#5866);
#4892=LINE('',#27833,#5867);
#4893=LINE('',#27852,#5868);
#4894=LINE('',#27855,#5869);
#4895=LINE('',#27857,#5870);
#4896=LINE('',#27864,#5871);
#4897=LINE('',#27866,#5872);
#4898=LINE('',#27875,#5873);
#4899=LINE('',#27894,#5874);
#4900=LINE('',#27897,#5875);
#4901=LINE('',#27899,#5876);
#4902=LINE('',#27906,#5877);
#4903=LINE('',#27908,#5878);
#4904=LINE('',#27917,#5879);
#4905=LINE('',#27936,#5880);
#4906=LINE('',#27939,#5881);
#4907=LINE('',#27941,#5882);
#4908=LINE('',#27948,#5883);
#4909=LINE('',#27950,#5884);
#4910=LINE('',#27959,#5885);
#4911=LINE('',#27978,#5886);
#4912=LINE('',#27981,#5887);
#4913=LINE('',#27986,#5888);
#4914=LINE('',#27991,#5889);
#4915=LINE('',#27998,#5890);
#4916=LINE('',#28034,#5891);
#4917=LINE('',#28038,#5892);
#4918=LINE('',#28041,#5893);
#4919=LINE('',#28042,#5894);
#4920=LINE('',#28079,#5895);
#4921=LINE('',#28081,#5896);
#4922=LINE('',#28082,#5897);
#4923=LINE('',#28087,#5898);
#4924=LINE('',#28089,#5899);
#4925=LINE('',#28108,#5900);
#4926=LINE('',#28110,#5901);
#4927=LINE('',#28111,#5902);
#4928=LINE('',#28116,#5903);
#4929=LINE('',#28124,#5904);
#4930=LINE('',#28126,#5905);
#4931=LINE('',#28128,#5906);
#4932=LINE('',#28146,#5907);
#4933=LINE('',#28147,#5908);
#4934=LINE('',#28155,#5909);
#4935=LINE('',#28159,#5910);
#4936=LINE('',#28161,#5911);
#4937=LINE('',#28180,#5912);
#4938=LINE('',#28182,#5913);
#4939=LINE('',#28183,#5914);
#4940=LINE('',#28188,#5915);
#4941=LINE('',#28196,#5916);
#4942=LINE('',#28198,#5917);
#4943=LINE('',#28200,#5918);
#4944=LINE('',#28218,#5919);
#4945=LINE('',#28219,#5920);
#4946=LINE('',#28227,#5921);
#4947=LINE('',#28231,#5922);
#4948=LINE('',#28233,#5923);
#4949=LINE('',#28252,#5924);
#4950=LINE('',#28254,#5925);
#4951=LINE('',#28255,#5926);
#4952=LINE('',#28260,#5927);
#4953=LINE('',#28267,#5928);
#4954=LINE('',#28269,#5929);
#4955=LINE('',#28283,#5930);
#4956=LINE('',#28284,#5931);
#4957=LINE('',#28289,#5932);
#4958=LINE('',#28296,#5933);
#4959=LINE('',#28402,#5934);
#4960=LINE('',#28419,#5935);
#4961=LINE('',#28423,#5936);
#4962=LINE('',#28427,#5937);
#4963=LINE('',#28431,#5938);
#4964=LINE('',#28435,#5939);
#4965=LINE('',#28439,#5940);
#4966=LINE('',#28443,#5941);
#4967=LINE('',#28447,#5942);
#4968=LINE('',#28451,#5943);
#4969=LINE('',#28455,#5944);
#4970=LINE('',#28458,#5945);
#4971=LINE('',#28575,#5946);
#4972=LINE('',#28580,#5947);
#4973=LINE('',#28585,#5948);
#4974=LINE('',#28590,#5949);
#4975=LINE('',#28595,#5950);
#4976=LINE('',#28598,#5951);
#5390=VECTOR('',#19365,10.);
#5391=VECTOR('',#19366,10.);
#5392=VECTOR('',#19367,10.);
#5393=VECTOR('',#19372,10.);
#5394=VECTOR('',#19381,10.);
#5395=VECTOR('',#19382,10.);
#5396=VECTOR('',#19383,10.);
#5397=VECTOR('',#19388,10.);
#5398=VECTOR('',#19397,10.);
#5399=VECTOR('',#19398,10.);
#5400=VECTOR('',#19403,10.);
#5401=VECTOR('',#19408,10.);
#5402=VECTOR('',#19409,10.);
#5403=VECTOR('',#19410,10.);
#5404=VECTOR('',#19421,10.);
#5405=VECTOR('',#19424,10.);
#5406=VECTOR('',#19425,10.);
#5407=VECTOR('',#19426,10.);
#5408=VECTOR('',#19439,10.);
#5409=VECTOR('',#19440,10.);
#5410=VECTOR('',#19441,10.);
#5411=VECTOR('',#19452,10.);
#5412=VECTOR('',#19455,10.);
#5413=VECTOR('',#19456,10.);
#5414=VECTOR('',#19459,10.);
#5415=VECTOR('',#19460,10.);
#5416=VECTOR('',#19463,10.);
#5417=VECTOR('',#19464,10.);
#5418=VECTOR('',#19465,10.);
#5419=VECTOR('',#19470,10.);
#5420=VECTOR('',#19481,10.);
#5421=VECTOR('',#19482,10.);
#5422=VECTOR('',#19483,10.);
#5423=VECTOR('',#19488,10.);
#5424=VECTOR('',#19497,10.);
#5425=VECTOR('',#19498,10.);
#5426=VECTOR('',#19499,10.);
#5427=VECTOR('',#19510,10.);
#5428=VECTOR('',#19513,10.);
#5429=VECTOR('',#19514,10.);
#5430=VECTOR('',#19517,10.);
#5431=VECTOR('',#19518,10.);
#5432=VECTOR('',#19519,10.);
#5433=VECTOR('',#19530,10.);
#5434=VECTOR('',#19533,10.);
#5435=VECTOR('',#19534,10.);
#5436=VECTOR('',#19537,10.);
#5437=VECTOR('',#19538,10.);
#5438=VECTOR('',#19539,10.);
#5439=VECTOR('',#19550,10.);
#5440=VECTOR('',#19553,10.);
#5441=VECTOR('',#19554,10.);
#5442=VECTOR('',#19557,10.);
#5443=VECTOR('',#19558,10.);
#5444=VECTOR('',#19559,10.);
#5445=VECTOR('',#19570,10.);
#5446=VECTOR('',#19573,10.);
#5447=VECTOR('',#19574,10.);
#5448=VECTOR('',#19577,10.);
#5449=VECTOR('',#19578,10.);
#5450=VECTOR('',#19579,10.);
#5451=VECTOR('',#19590,10.);
#5452=VECTOR('',#19593,10.);
#5453=VECTOR('',#19594,10.);
#5454=VECTOR('',#19597,10.);
#5455=VECTOR('',#19598,10.);
#5456=VECTOR('',#19599,10.);
#5457=VECTOR('',#19610,10.);
#5458=VECTOR('',#19613,10.);
#5459=VECTOR('',#19614,10.);
#5460=VECTOR('',#19617,10.);
#5461=VECTOR('',#19618,10.);
#5462=VECTOR('',#19619,10.);
#5463=VECTOR('',#19630,10.);
#5464=VECTOR('',#19633,10.);
#5465=VECTOR('',#19634,10.);
#5466=VECTOR('',#19637,10.);
#5467=VECTOR('',#19638,10.);
#5468=VECTOR('',#19639,10.);
#5469=VECTOR('',#19650,10.);
#5470=VECTOR('',#19653,10.);
#5471=VECTOR('',#19654,10.);
#5472=VECTOR('',#20003,10.);
#5473=VECTOR('',#20006,10.);
#5474=VECTOR('',#20009,10.);
#5475=VECTOR('',#20010,10.);
#5476=VECTOR('',#20013,10.);
#5477=VECTOR('',#20014,10.);
#5478=VECTOR('',#20015,10.);
#5479=VECTOR('',#20024,10.);
#5480=VECTOR('',#20027,10.);
#5481=VECTOR('',#20028,10.);
#5482=VECTOR('',#20031,10.);
#5483=VECTOR('',#20032,10.);
#5484=VECTOR('',#20033,10.);
#5485=VECTOR('',#20042,10.);
#5486=VECTOR('',#20045,10.);
#5487=VECTOR('',#20046,10.);
#5488=VECTOR('',#20049,10.);
#5489=VECTOR('',#20050,10.);
#5490=VECTOR('',#20051,10.);
#5491=VECTOR('',#20060,10.);
#5492=VECTOR('',#20063,10.);
#5493=VECTOR('',#20064,10.);
#5494=VECTOR('',#20069,10.);
#5495=VECTOR('',#20076,10.);
#5496=VECTOR('',#20079,10.);
#5497=VECTOR('',#20080,10.);
#5498=VECTOR('',#20081,10.);
#5499=VECTOR('',#20090,10.);
#5500=VECTOR('',#20093,10.);
#5501=VECTOR('',#20094,10.);
#5502=VECTOR('',#20097,10.);
#5503=VECTOR('',#20098,10.);
#5504=VECTOR('',#20099,10.);
#5505=VECTOR('',#20108,10.);
#5506=VECTOR('',#20111,10.);
#5507=VECTOR('',#20112,10.);
#5508=VECTOR('',#20115,10.);
#5509=VECTOR('',#20116,10.);
#5510=VECTOR('',#20117,10.);
#5511=VECTOR('',#20126,10.);
#5512=VECTOR('',#20129,10.);
#5513=VECTOR('',#20130,10.);
#5514=VECTOR('',#20133,10.);
#5515=VECTOR('',#20134,10.);
#5516=VECTOR('',#20135,10.);
#5517=VECTOR('',#20144,10.);
#5518=VECTOR('',#20147,10.);
#5519=VECTOR('',#20148,10.);
#5520=VECTOR('',#20151,10.);
#5521=VECTOR('',#20152,10.);
#5522=VECTOR('',#20153,10.);
#5523=VECTOR('',#20162,10.);
#5524=VECTOR('',#20165,10.);
#5525=VECTOR('',#20166,10.);
#5526=VECTOR('',#20169,10.);
#5527=VECTOR('',#20170,10.);
#5528=VECTOR('',#20171,10.);
#5529=VECTOR('',#20180,10.);
#5530=VECTOR('',#20183,10.);
#5531=VECTOR('',#20184,10.);
#5532=VECTOR('',#20185,10.);
#5533=VECTOR('',#20212,10.);
#5534=VECTOR('',#20213,10.);
#5535=VECTOR('',#20260,10.);
#5536=VECTOR('',#20261,10.);
#5537=VECTOR('',#20262,10.);
#5538=VECTOR('',#20271,10.);
#5539=VECTOR('',#20274,10.);
#5540=VECTOR('',#20275,10.);
#5541=VECTOR('',#20282,10.);
#5542=VECTOR('',#20283,10.);
#5543=VECTOR('',#20284,10.);
#5544=VECTOR('',#20293,10.);
#5545=VECTOR('',#20296,10.);
#5546=VECTOR('',#20297,10.);
#5547=VECTOR('',#20300,10.);
#5548=VECTOR('',#20301,10.);
#5549=VECTOR('',#20302,10.);
#5550=VECTOR('',#20311,10.);
#5551=VECTOR('',#20314,10.);
#5552=VECTOR('',#20315,10.);
#5553=VECTOR('',#20318,10.);
#5554=VECTOR('',#20319,10.);
#5555=VECTOR('',#20320,10.);
#5556=VECTOR('',#20329,10.);
#5557=VECTOR('',#20332,10.);
#5558=VECTOR('',#20333,10.);
#5559=VECTOR('',#20334,10.);
#5560=VECTOR('',#20339,10.);
#5561=VECTOR('',#20346,10.);
#5562=VECTOR('',#20349,10.);
#5563=VECTOR('',#20350,10.);
#5564=VECTOR('',#20351,10.);
#5565=VECTOR('',#20360,10.);
#5566=VECTOR('',#20363,10.);
#5567=VECTOR('',#20364,10.);
#5568=VECTOR('',#20367,10.);
#5569=VECTOR('',#20368,10.);
#5570=VECTOR('',#20369,10.);
#5571=VECTOR('',#20378,10.);
#5572=VECTOR('',#20381,10.);
#5573=VECTOR('',#20382,10.);
#5574=VECTOR('',#20385,10.);
#5575=VECTOR('',#20386,10.);
#5576=VECTOR('',#20387,10.);
#5577=VECTOR('',#20396,10.);
#5578=VECTOR('',#20399,10.);
#5579=VECTOR('',#20400,10.);
#5580=VECTOR('',#20403,10.);
#5581=VECTOR('',#20404,10.);
#5582=VECTOR('',#20405,10.);
#5583=VECTOR('',#20414,10.);
#5584=VECTOR('',#20417,10.);
#5585=VECTOR('',#20418,10.);
#5586=VECTOR('',#20421,10.);
#5587=VECTOR('',#20422,10.);
#5588=VECTOR('',#20423,10.);
#5589=VECTOR('',#20432,10.);
#5590=VECTOR('',#20435,10.);
#5591=VECTOR('',#20436,10.);
#5592=VECTOR('',#20437,10.);
#5593=VECTOR('',#20468,10.);
#5594=VECTOR('',#20469,10.);
#5595=VECTOR('',#20508,10.);
#5596=VECTOR('',#20509,10.);
#5597=VECTOR('',#20510,10.);
#5598=VECTOR('',#20519,10.);
#5599=VECTOR('',#20522,10.);
#5600=VECTOR('',#20523,10.);
#5601=VECTOR('',#20526,10.);
#5602=VECTOR('',#20527,10.);
#5603=VECTOR('',#20528,10.);
#5604=VECTOR('',#20537,10.);
#5605=VECTOR('',#20540,10.);
#5606=VECTOR('',#20541,10.);
#5607=VECTOR('',#20544,10.);
#5608=VECTOR('',#20545,10.);
#5609=VECTOR('',#20546,10.);
#5610=VECTOR('',#20555,10.);
#5611=VECTOR('',#20558,10.);
#5612=VECTOR('',#20559,10.);
#5613=VECTOR('',#20562,10.);
#5614=VECTOR('',#20563,10.);
#5615=VECTOR('',#20564,10.);
#5616=VECTOR('',#20573,10.);
#5617=VECTOR('',#20576,10.);
#5618=VECTOR('',#20577,10.);
#5619=VECTOR('',#20580,10.);
#5620=VECTOR('',#20581,10.);
#5621=VECTOR('',#20582,10.);
#5622=VECTOR('',#20591,10.);
#5623=VECTOR('',#20594,10.);
#5624=VECTOR('',#20595,10.);
#5625=VECTOR('',#20596,10.);
#5626=VECTOR('',#20601,10.);
#5627=VECTOR('',#20608,10.);
#5628=VECTOR('',#20611,10.);
#5629=VECTOR('',#20612,10.);
#5630=VECTOR('',#20613,10.);
#5631=VECTOR('',#20622,10.);
#5632=VECTOR('',#20625,10.);
#5633=VECTOR('',#20626,10.);
#5634=VECTOR('',#20629,10.);
#5635=VECTOR('',#20630,10.);
#5636=VECTOR('',#20631,10.);
#5637=VECTOR('',#20640,10.);
#5638=VECTOR('',#20643,10.);
#5639=VECTOR('',#20644,10.);
#5640=VECTOR('',#20647,10.);
#5641=VECTOR('',#20648,10.);
#5642=VECTOR('',#20649,10.);
#5643=VECTOR('',#20658,10.);
#5644=VECTOR('',#20661,10.);
#5645=VECTOR('',#20662,10.);
#5646=VECTOR('',#20665,10.);
#5647=VECTOR('',#20666,10.);
#5648=VECTOR('',#20667,10.);
#5649=VECTOR('',#20676,10.);
#5650=VECTOR('',#20679,10.);
#5651=VECTOR('',#20680,10.);
#5652=VECTOR('',#20681,10.);
#5653=VECTOR('',#20724,10.);
#5654=VECTOR('',#20725,10.);
#5655=VECTOR('',#20756,10.);
#5656=VECTOR('',#20757,10.);
#5657=VECTOR('',#20758,10.);
#5658=VECTOR('',#20767,10.);
#5659=VECTOR('',#20770,10.);
#5660=VECTOR('',#20771,10.);
#5661=VECTOR('',#20778,10.);
#5662=VECTOR('',#20779,10.);
#5663=VECTOR('',#20780,10.);
#5664=VECTOR('',#20789,10.);
#5665=VECTOR('',#20792,10.);
#5666=VECTOR('',#20793,10.);
#5667=VECTOR('',#20796,10.);
#5668=VECTOR('',#20797,10.);
#5669=VECTOR('',#20798,10.);
#5670=VECTOR('',#20807,10.);
#5671=VECTOR('',#20810,10.);
#5672=VECTOR('',#20811,10.);
#5673=VECTOR('',#20814,10.);
#5674=VECTOR('',#20815,10.);
#5675=VECTOR('',#20816,10.);
#5676=VECTOR('',#20825,10.);
#5677=VECTOR('',#20828,10.);
#5678=VECTOR('',#20829,10.);
#5679=VECTOR('',#20832,10.);
#5680=VECTOR('',#20833,10.);
#5681=VECTOR('',#20834,10.);
#5682=VECTOR('',#20843,10.);
#5683=VECTOR('',#20846,10.);
#5684=VECTOR('',#20847,10.);
#5685=VECTOR('',#20850,10.);
#5686=VECTOR('',#20851,10.);
#5687=VECTOR('',#20852,10.);
#5688=VECTOR('',#20861,10.);
#5689=VECTOR('',#20864,10.);
#5690=VECTOR('',#20865,10.);
#5691=VECTOR('',#20866,10.);
#5692=VECTOR('',#20871,10.);
#5693=VECTOR('',#20878,10.);
#5694=VECTOR('',#20881,10.);
#5695=VECTOR('',#20882,10.);
#5696=VECTOR('',#20883,10.);
#5697=VECTOR('',#20892,10.);
#5698=VECTOR('',#20895,10.);
#5699=VECTOR('',#20896,10.);
#5700=VECTOR('',#20899,10.);
#5701=VECTOR('',#20900,10.);
#5702=VECTOR('',#20901,10.);
#5703=VECTOR('',#20910,10.);
#5704=VECTOR('',#20913,10.);
#5705=VECTOR('',#20914,10.);
#5706=VECTOR('',#20917,10.);
#5707=VECTOR('',#20918,10.);
#5708=VECTOR('',#20919,10.);
#5709=VECTOR('',#20928,10.);
#5710=VECTOR('',#20931,10.);
#5711=VECTOR('',#20932,10.);
#5712=VECTOR('',#20933,10.);
#5713=VECTOR('',#20980,10.);
#5714=VECTOR('',#20981,10.);
#5715=VECTOR('',#21004,10.);
#5716=VECTOR('',#21005,10.);
#5717=VECTOR('',#21006,10.);
#5718=VECTOR('',#21015,10.);
#5719=VECTOR('',#21018,10.);
#5720=VECTOR('',#21019,10.);
#5721=VECTOR('',#21022,10.);
#5722=VECTOR('',#21023,10.);
#5723=VECTOR('',#21024,10.);
#5724=VECTOR('',#21033,10.);
#5725=VECTOR('',#21036,10.);
#5726=VECTOR('',#21037,10.);
#5727=VECTOR('',#21040,10.);
#5728=VECTOR('',#21041,10.);
#5729=VECTOR('',#21042,10.);
#5730=VECTOR('',#21051,10.);
#5731=VECTOR('',#21054,10.);
#5732=VECTOR('',#21055,10.);
#5733=VECTOR('',#21058,10.);
#5734=VECTOR('',#21059,10.);
#5735=VECTOR('',#21060,10.);
#5736=VECTOR('',#21069,10.);
#5737=VECTOR('',#21072,10.);
#5738=VECTOR('',#21073,10.);
#5739=VECTOR('',#21076,10.);
#5740=VECTOR('',#21077,10.);
#5741=VECTOR('',#21078,10.);
#5742=VECTOR('',#21087,10.);
#5743=VECTOR('',#21090,10.);
#5744=VECTOR('',#21091,10.);
#5745=VECTOR('',#21094,10.);
#5746=VECTOR('',#21095,10.);
#5747=VECTOR('',#21096,10.);
#5748=VECTOR('',#21105,10.);
#5749=VECTOR('',#21108,10.);
#5750=VECTOR('',#21109,10.);
#5751=VECTOR('',#21112,10.);
#5752=VECTOR('',#21113,10.);
#5753=VECTOR('',#21114,10.);
#5754=VECTOR('',#21123,10.);
#5755=VECTOR('',#21126,10.);
#5756=VECTOR('',#21127,10.);
#5757=VECTOR('',#21128,10.);
#5758=VECTOR('',#21133,10.);
#5759=VECTOR('',#21140,10.);
#5760=VECTOR('',#21143,10.);
#5761=VECTOR('',#21144,10.);
#5762=VECTOR('',#21145,10.);
#5763=VECTOR('',#21154,10.);
#5764=VECTOR('',#21157,10.);
#5765=VECTOR('',#21158,10.);
#5766=VECTOR('',#21161,10.);
#5767=VECTOR('',#21162,10.);
#5768=VECTOR('',#21163,10.);
#5769=VECTOR('',#21172,10.);
#5770=VECTOR('',#21175,10.);
#5771=VECTOR('',#21176,10.);
#5772=VECTOR('',#21177,10.);
#5773=VECTOR('',#21236,10.);
#5774=VECTOR('',#21237,10.);
#5775=VECTOR('',#21252,10.);
#5776=VECTOR('',#21253,10.);
#5777=VECTOR('',#21254,10.);
#5778=VECTOR('',#21263,10.);
#5779=VECTOR('',#21266,10.);
#5780=VECTOR('',#21267,10.);
#5781=VECTOR('',#21270,10.);
#5782=VECTOR('',#21271,10.);
#5783=VECTOR('',#21272,10.);
#5784=VECTOR('',#21281,10.);
#5785=VECTOR('',#21284,10.);
#5786=VECTOR('',#21285,10.);
#5787=VECTOR('',#21288,10.);
#5788=VECTOR('',#21289,10.);
#5789=VECTOR('',#21290,10.);
#5790=VECTOR('',#21299,10.);
#5791=VECTOR('',#21302,10.);
#5792=VECTOR('',#21303,10.);
#5793=VECTOR('',#21306,10.);
#5794=VECTOR('',#21307,10.);
#5795=VECTOR('',#21308,10.);
#5796=VECTOR('',#21317,10.);
#5797=VECTOR('',#21320,10.);
#5798=VECTOR('',#21321,10.);
#5799=VECTOR('',#21324,10.);
#5800=VECTOR('',#21325,10.);
#5801=VECTOR('',#21326,10.);
#5802=VECTOR('',#21335,10.);
#5803=VECTOR('',#21338,10.);
#5804=VECTOR('',#21339,10.);
#5805=VECTOR('',#21342,10.);
#5806=VECTOR('',#21343,10.);
#5807=VECTOR('',#21344,10.);
#5808=VECTOR('',#21353,10.);
#5809=VECTOR('',#21356,10.);
#5810=VECTOR('',#21357,10.);
#5811=VECTOR('',#21360,10.);
#5812=VECTOR('',#21361,10.);
#5813=VECTOR('',#21362,10.);
#5814=VECTOR('',#21371,10.);
#5815=VECTOR('',#21374,10.);
#5816=VECTOR('',#21375,10.);
#5817=VECTOR('',#21378,10.);
#5818=VECTOR('',#21379,10.);
#5819=VECTOR('',#21380,10.);
#5820=VECTOR('',#21389,10.);
#5821=VECTOR('',#21392,10.);
#5822=VECTOR('',#21393,10.);
#5823=VECTOR('',#21394,10.);
#5824=VECTOR('',#21399,10.);
#5825=VECTOR('',#21406,10.);
#5826=VECTOR('',#21409,10.);
#5827=VECTOR('',#21410,10.);
#5828=VECTOR('',#21411,10.);
#5829=VECTOR('',#21420,10.);
#5830=VECTOR('',#21423,10.);
#5831=VECTOR('',#21424,10.);
#5832=VECTOR('',#21425,10.);
#5833=VECTOR('',#21492,10.);
#5834=VECTOR('',#21493,10.);
#5835=VECTOR('',#21500,10.);
#5836=VECTOR('',#21501,10.);
#5837=VECTOR('',#21502,10.);
#5838=VECTOR('',#21511,10.);
#5839=VECTOR('',#21514,10.);
#5840=VECTOR('',#21515,10.);
#5841=VECTOR('',#21518,10.);
#5842=VECTOR('',#21519,10.);
#5843=VECTOR('',#21520,10.);
#5844=VECTOR('',#21529,10.);
#5845=VECTOR('',#21532,10.);
#5846=VECTOR('',#21533,10.);
#5847=VECTOR('',#21536,10.);
#5848=VECTOR('',#21537,10.);
#5849=VECTOR('',#21538,10.);
#5850=VECTOR('',#21547,10.);
#5851=VECTOR('',#21550,10.);
#5852=VECTOR('',#21551,10.);
#5853=VECTOR('',#21554,10.);
#5854=VECTOR('',#21555,10.);
#5855=VECTOR('',#21556,10.);
#5856=VECTOR('',#21565,10.);
#5857=VECTOR('',#21568,10.);
#5858=VECTOR('',#21569,10.);
#5859=VECTOR('',#21572,10.);
#5860=VECTOR('',#21573,10.);
#5861=VECTOR('',#21574,10.);
#5862=VECTOR('',#21583,10.);
#5863=VECTOR('',#21586,10.);
#5864=VECTOR('',#21587,10.);
#5865=VECTOR('',#21590,10.);
#5866=VECTOR('',#21591,10.);
#5867=VECTOR('',#21592,10.);
#5868=VECTOR('',#21601,10.);
#5869=VECTOR('',#21604,10.);
#5870=VECTOR('',#21605,10.);
#5871=VECTOR('',#21608,10.);
#5872=VECTOR('',#21609,10.);
#5873=VECTOR('',#21610,10.);
#5874=VECTOR('',#21619,10.);
#5875=VECTOR('',#21622,10.);
#5876=VECTOR('',#21623,10.);
#5877=VECTOR('',#21626,10.);
#5878=VECTOR('',#21627,10.);
#5879=VECTOR('',#21628,10.);
#5880=VECTOR('',#21637,10.);
#5881=VECTOR('',#21640,10.);
#5882=VECTOR('',#21641,10.);
#5883=VECTOR('',#21644,10.);
#5884=VECTOR('',#21645,10.);
#5885=VECTOR('',#21646,10.);
#5886=VECTOR('',#21655,10.);
#5887=VECTOR('',#21658,10.);
#5888=VECTOR('',#21659,10.);
#5889=VECTOR('',#21664,10.);
#5890=VECTOR('',#21671,10.);
#5891=VECTOR('',#21740,49.75);
#5892=VECTOR('',#21745,49.5);
#5893=VECTOR('',#21748,10.);
#5894=VECTOR('',#21749,10.);
#5895=VECTOR('',#21820,10.);
#5896=VECTOR('',#21821,10.);
#5897=VECTOR('',#21822,10.);
#5898=VECTOR('',#21829,10.);
#5899=VECTOR('',#21830,10.);
#5900=VECTOR('',#21837,10.);
#5901=VECTOR('',#21838,10.);
#5902=VECTOR('',#21839,10.);
#5903=VECTOR('',#21844,10.);
#5904=VECTOR('',#21847,10.);
#5905=VECTOR('',#21848,10.);
#5906=VECTOR('',#21849,10.);
#5907=VECTOR('',#21856,10.);
#5908=VECTOR('',#21857,10.);
#5909=VECTOR('',#21860,10.);
#5910=VECTOR('',#21865,10.);
#5911=VECTOR('',#21866,10.);
#5912=VECTOR('',#21873,10.);
#5913=VECTOR('',#21874,10.);
#5914=VECTOR('',#21875,10.);
#5915=VECTOR('',#21880,10.);
#5916=VECTOR('',#21883,10.);
#5917=VECTOR('',#21884,10.);
#5918=VECTOR('',#21885,10.);
#5919=VECTOR('',#21892,10.);
#5920=VECTOR('',#21893,10.);
#5921=VECTOR('',#21896,10.);
#5922=VECTOR('',#21901,10.);
#5923=VECTOR('',#21902,10.);
#5924=VECTOR('',#21909,10.);
#5925=VECTOR('',#21910,10.);
#5926=VECTOR('',#21911,10.);
#5927=VECTOR('',#21916,10.);
#5928=VECTOR('',#21919,10.);
#5929=VECTOR('',#21920,10.);
#5930=VECTOR('',#21927,10.);
#5931=VECTOR('',#21928,10.);
#5932=VECTOR('',#21933,52.6267766952966);
#5933=VECTOR('',#21942,53.1);
#5934=VECTOR('',#22149,12.7);
#5935=VECTOR('',#22168,12.5);
#5936=VECTOR('',#22173,12.7);
#5937=VECTOR('',#22178,12.5);
#5938=VECTOR('',#22183,12.7);
#5939=VECTOR('',#22188,12.5);
#5940=VECTOR('',#22193,12.7);
#5941=VECTOR('',#22198,12.5);
#5942=VECTOR('',#22203,12.7);
#5943=VECTOR('',#22208,12.5);
#5944=VECTOR('',#22213,50.8);
#5945=VECTOR('',#22218,50.5);
#5946=VECTOR('',#22447,1.5);
#5947=VECTOR('',#22452,1.5);
#5948=VECTOR('',#22457,1.5);
#5949=VECTOR('',#22462,1.5);
#5950=VECTOR('',#22467,1.5);
#5951=VECTOR('',#22470,5.025);
#6339=VERTEX_POINT('',#23995);
#6340=VERTEX_POINT('',#23996);
#6341=VERTEX_POINT('',#24000);
#6342=VERTEX_POINT('',#24002);
#6343=VERTEX_POINT('',#24006);
#6344=VERTEX_POINT('',#24008);
#6345=VERTEX_POINT('',#24012);
#6346=VERTEX_POINT('',#24017);
#6347=VERTEX_POINT('',#24019);
#6348=VERTEX_POINT('',#24028);
#6349=VERTEX_POINT('',#24029);
#6350=VERTEX_POINT('',#24033);
#6351=VERTEX_POINT('',#24035);
#6352=VERTEX_POINT('',#24037);
#6353=VERTEX_POINT('',#24043);
#6354=VERTEX_POINT('',#24045);
#6355=VERTEX_POINT('',#24049);
#6356=VERTEX_POINT('',#24054);
#6357=VERTEX_POINT('',#24056);
#6358=VERTEX_POINT('',#24065);
#6359=VERTEX_POINT('',#24069);
#6360=VERTEX_POINT('',#24071);
#6361=VERTEX_POINT('',#24076);
#6362=VERTEX_POINT('',#24080);
#6363=VERTEX_POINT('',#24081);
#6364=VERTEX_POINT('',#24085);
#6365=VERTEX_POINT('',#24087);
#6366=VERTEX_POINT('',#24089);
#6367=VERTEX_POINT('',#24095);
#6368=VERTEX_POINT('',#24097);
#6369=VERTEX_POINT('',#24101);
#6370=VERTEX_POINT('',#24106);
#6371=VERTEX_POINT('',#24113);
#6372=VERTEX_POINT('',#24117);
#6373=VERTEX_POINT('',#24118);
#6374=VERTEX_POINT('',#24120);
#6375=VERTEX_POINT('',#24122);
#6376=VERTEX_POINT('',#24126);
#6377=VERTEX_POINT('',#24135);
#6378=VERTEX_POINT('',#24142);
#6379=VERTEX_POINT('',#24143);
#6380=VERTEX_POINT('',#24147);
#6381=VERTEX_POINT('',#24149);
#6382=VERTEX_POINT('',#24151);
#6383=VERTEX_POINT('',#24157);
#6384=VERTEX_POINT('',#24159);
#6385=VERTEX_POINT('',#24163);
#6386=VERTEX_POINT('',#24168);
#6387=VERTEX_POINT('',#24175);
#6388=VERTEX_POINT('',#24179);
#6389=VERTEX_POINT('',#24181);
#6390=VERTEX_POINT('',#24187);
#6391=VERTEX_POINT('',#24189);
#6392=VERTEX_POINT('',#24195);
#6393=VERTEX_POINT('',#24196);
#6394=VERTEX_POINT('',#24198);
#6395=VERTEX_POINT('',#24200);
#6396=VERTEX_POINT('',#24206);
#6397=VERTEX_POINT('',#24211);
#6398=VERTEX_POINT('',#24213);
#6399=VERTEX_POINT('',#24218);
#6400=VERTEX_POINT('',#24222);
#6401=VERTEX_POINT('',#24224);
#6402=VERTEX_POINT('',#24229);
#6403=VERTEX_POINT('',#24236);
#6404=VERTEX_POINT('',#24237);
#6405=VERTEX_POINT('',#24241);
#6406=VERTEX_POINT('',#24243);
#6407=VERTEX_POINT('',#24245);
#6408=VERTEX_POINT('',#24251);
#6409=VERTEX_POINT('',#24253);
#6410=VERTEX_POINT('',#24257);
#6411=VERTEX_POINT('',#24262);
#6412=VERTEX_POINT('',#24264);
#6413=VERTEX_POINT('',#24274);
#6414=VERTEX_POINT('',#24275);
#6415=VERTEX_POINT('',#24277);
#6416=VERTEX_POINT('',#24279);
#6417=VERTEX_POINT('',#24283);
#6418=VERTEX_POINT('',#24289);
#6419=VERTEX_POINT('',#24291);
#6420=VERTEX_POINT('',#24295);
#6421=VERTEX_POINT('',#24300);
#6422=VERTEX_POINT('',#24307);
#6423=VERTEX_POINT('',#24311);
#6424=VERTEX_POINT('',#24313);
#6425=VERTEX_POINT('',#24319);
#6426=VERTEX_POINT('',#24320);
#6427=VERTEX_POINT('',#24322);
#6428=VERTEX_POINT('',#24324);
#6429=VERTEX_POINT('',#24328);
#6430=VERTEX_POINT('',#24334);
#6431=VERTEX_POINT('',#24336);
#6432=VERTEX_POINT('',#24340);
#6433=VERTEX_POINT('',#24345);
#6434=VERTEX_POINT('',#24352);
#6435=VERTEX_POINT('',#24356);
#6436=VERTEX_POINT('',#24358);
#6437=VERTEX_POINT('',#24364);
#6438=VERTEX_POINT('',#24365);
#6439=VERTEX_POINT('',#24367);
#6440=VERTEX_POINT('',#24369);
#6441=VERTEX_POINT('',#24373);
#6442=VERTEX_POINT('',#24379);
#6443=VERTEX_POINT('',#24381);
#6444=VERTEX_POINT('',#24385);
#6445=VERTEX_POINT('',#24390);
#6446=VERTEX_POINT('',#24397);
#6447=VERTEX_POINT('',#24401);
#6448=VERTEX_POINT('',#24403);
#6449=VERTEX_POINT('',#24409);
#6450=VERTEX_POINT('',#24410);
#6451=VERTEX_POINT('',#24412);
#6452=VERTEX_POINT('',#24414);
#6453=VERTEX_POINT('',#24418);
#6454=VERTEX_POINT('',#24424);
#6455=VERTEX_POINT('',#24426);
#6456=VERTEX_POINT('',#24430);
#6457=VERTEX_POINT('',#24435);
#6458=VERTEX_POINT('',#24442);
#6459=VERTEX_POINT('',#24446);
#6460=VERTEX_POINT('',#24448);
#6461=VERTEX_POINT('',#24454);
#6462=VERTEX_POINT('',#24455);
#6463=VERTEX_POINT('',#24457);
#6464=VERTEX_POINT('',#24459);
#6465=VERTEX_POINT('',#24463);
#6466=VERTEX_POINT('',#24469);
#6467=VERTEX_POINT('',#24471);
#6468=VERTEX_POINT('',#24475);
#6469=VERTEX_POINT('',#24480);
#6470=VERTEX_POINT('',#24487);
#6471=VERTEX_POINT('',#24491);
#6472=VERTEX_POINT('',#24493);
#6473=VERTEX_POINT('',#24499);
#6474=VERTEX_POINT('',#24500);
#6475=VERTEX_POINT('',#24502);
#6476=VERTEX_POINT('',#24504);
#6477=VERTEX_POINT('',#24508);
#6478=VERTEX_POINT('',#24514);
#6479=VERTEX_POINT('',#24516);
#6480=VERTEX_POINT('',#24520);
#6481=VERTEX_POINT('',#24525);
#6482=VERTEX_POINT('',#24532);
#6483=VERTEX_POINT('',#24536);
#6484=VERTEX_POINT('',#24538);
#6485=VERTEX_POINT('',#24544);
#6486=VERTEX_POINT('',#24545);
#6487=VERTEX_POINT('',#24547);
#6488=VERTEX_POINT('',#24549);
#6489=VERTEX_POINT('',#24553);
#6490=VERTEX_POINT('',#24559);
#6491=VERTEX_POINT('',#24561);
#6492=VERTEX_POINT('',#24565);
#6493=VERTEX_POINT('',#24570);
#6494=VERTEX_POINT('',#24577);
#6495=VERTEX_POINT('',#24581);
#6496=VERTEX_POINT('',#24583);
#6497=VERTEX_POINT('',#24589);
#6498=VERTEX_POINT('',#24590);
#6499=VERTEX_POINT('',#24592);
#6500=VERTEX_POINT('',#24594);
#6501=VERTEX_POINT('',#24598);
#6502=VERTEX_POINT('',#24604);
#6503=VERTEX_POINT('',#24606);
#6504=VERTEX_POINT('',#24610);
#6505=VERTEX_POINT('',#24615);
#6506=VERTEX_POINT('',#24622);
#6507=VERTEX_POINT('',#24626);
#6508=VERTEX_POINT('',#24628);
#6509=VERTEX_POINT('',#24634);
#6510=VERTEX_POINT('',#24636);
#6511=VERTEX_POINT('',#24640);
#6512=VERTEX_POINT('',#24655);
#6513=VERTEX_POINT('',#24657);
#6514=VERTEX_POINT('',#24661);
#6515=VERTEX_POINT('',#24668);
#6516=VERTEX_POINT('',#24670);
#6517=VERTEX_POINT('',#24672);
#6518=VERTEX_POINT('',#24674);
#6519=VERTEX_POINT('',#24676);
#6520=VERTEX_POINT('',#24678);
#6521=VERTEX_POINT('',#24680);
#6522=VERTEX_POINT('',#24682);
#6523=VERTEX_POINT('',#24684);
#6524=VERTEX_POINT('',#24686);
#6525=VERTEX_POINT('',#24688);
#6526=VERTEX_POINT('',#24700);
#6527=VERTEX_POINT('',#24702);
#6528=VERTEX_POINT('',#24704);
#6529=VERTEX_POINT('',#24706);
#6530=VERTEX_POINT('',#24708);
#6531=VERTEX_POINT('',#24710);
#6532=VERTEX_POINT('',#24712);
#6533=VERTEX_POINT('',#24714);
#6534=VERTEX_POINT('',#24716);
#6535=VERTEX_POINT('',#24718);
#6536=VERTEX_POINT('',#24720);
#6537=VERTEX_POINT('',#24722);
#6538=VERTEX_POINT('',#24724);
#6539=VERTEX_POINT('',#24726);
#6540=VERTEX_POINT('',#24728);
#6541=VERTEX_POINT('',#24730);
#6542=VERTEX_POINT('',#24732);
#6543=VERTEX_POINT('',#24735);
#6544=VERTEX_POINT('',#24737);
#6545=VERTEX_POINT('',#24739);
#6546=VERTEX_POINT('',#24741);
#6547=VERTEX_POINT('',#24743);
#6548=VERTEX_POINT('',#24745);
#6549=VERTEX_POINT('',#24747);
#6550=VERTEX_POINT('',#24749);
#6551=VERTEX_POINT('',#24751);
#6552=VERTEX_POINT('',#24753);
#6553=VERTEX_POINT('',#24755);
#6554=VERTEX_POINT('',#24757);
#6555=VERTEX_POINT('',#24759);
#6556=VERTEX_POINT('',#24761);
#6557=VERTEX_POINT('',#24763);
#6558=VERTEX_POINT('',#24765);
#6559=VERTEX_POINT('',#24767);
#6560=VERTEX_POINT('',#24769);
#6561=VERTEX_POINT('',#24771);
#6562=VERTEX_POINT('',#24773);
#6563=VERTEX_POINT('',#24775);
#6564=VERTEX_POINT('',#24777);
#6565=VERTEX_POINT('',#24779);
#6566=VERTEX_POINT('',#24781);
#6567=VERTEX_POINT('',#24783);
#6568=VERTEX_POINT('',#24785);
#6569=VERTEX_POINT('',#24787);
#6570=VERTEX_POINT('',#24789);
#6571=VERTEX_POINT('',#24791);
#6572=VERTEX_POINT('',#24793);
#6573=VERTEX_POINT('',#24795);
#6574=VERTEX_POINT('',#24797);
#6575=VERTEX_POINT('',#24799);
#6576=VERTEX_POINT('',#24801);
#6577=VERTEX_POINT('',#24803);
#6578=VERTEX_POINT('',#24805);
#6579=VERTEX_POINT('',#24807);
#6580=VERTEX_POINT('',#24809);
#6581=VERTEX_POINT('',#24811);
#6582=VERTEX_POINT('',#24813);
#6583=VERTEX_POINT('',#24815);
#6584=VERTEX_POINT('',#24817);
#6585=VERTEX_POINT('',#24819);
#6586=VERTEX_POINT('',#24821);
#6587=VERTEX_POINT('',#24823);
#6588=VERTEX_POINT('',#24825);
#6589=VERTEX_POINT('',#24827);
#6590=VERTEX_POINT('',#24829);
#6591=VERTEX_POINT('',#24831);
#6592=VERTEX_POINT('',#24833);
#6593=VERTEX_POINT('',#24835);
#6594=VERTEX_POINT('',#24837);
#6595=VERTEX_POINT('',#24839);
#6596=VERTEX_POINT('',#24841);
#6597=VERTEX_POINT('',#24843);
#6598=VERTEX_POINT('',#24845);
#6599=VERTEX_POINT('',#24847);
#6600=VERTEX_POINT('',#24849);
#6601=VERTEX_POINT('',#24851);
#6602=VERTEX_POINT('',#24853);
#6603=VERTEX_POINT('',#24855);
#6604=VERTEX_POINT('',#24857);
#6605=VERTEX_POINT('',#24859);
#6606=VERTEX_POINT('',#24861);
#6607=VERTEX_POINT('',#24863);
#6608=VERTEX_POINT('',#24865);
#6609=VERTEX_POINT('',#24867);
#6610=VERTEX_POINT('',#24869);
#6611=VERTEX_POINT('',#24871);
#6612=VERTEX_POINT('',#24873);
#6613=VERTEX_POINT('',#24875);
#6614=VERTEX_POINT('',#24877);
#6615=VERTEX_POINT('',#24879);
#6616=VERTEX_POINT('',#24881);
#6617=VERTEX_POINT('',#24883);
#6618=VERTEX_POINT('',#24885);
#6619=VERTEX_POINT('',#24887);
#6620=VERTEX_POINT('',#24889);
#6621=VERTEX_POINT('',#24891);
#6622=VERTEX_POINT('',#24893);
#6623=VERTEX_POINT('',#24895);
#6624=VERTEX_POINT('',#24897);
#6625=VERTEX_POINT('',#24899);
#6626=VERTEX_POINT('',#24901);
#6627=VERTEX_POINT('',#24903);
#6628=VERTEX_POINT('',#24905);
#6629=VERTEX_POINT('',#24907);
#6630=VERTEX_POINT('',#24909);
#6631=VERTEX_POINT('',#24911);
#6632=VERTEX_POINT('',#24913);
#6633=VERTEX_POINT('',#24915);
#6634=VERTEX_POINT('',#24917);
#6635=VERTEX_POINT('',#24919);
#6636=VERTEX_POINT('',#24921);
#6637=VERTEX_POINT('',#24923);
#6638=VERTEX_POINT('',#24925);
#6639=VERTEX_POINT('',#24927);
#6640=VERTEX_POINT('',#24929);
#6641=VERTEX_POINT('',#24931);
#6642=VERTEX_POINT('',#24933);
#6643=VERTEX_POINT('',#24935);
#6644=VERTEX_POINT('',#24937);
#6645=VERTEX_POINT('',#24939);
#6646=VERTEX_POINT('',#24941);
#6647=VERTEX_POINT('',#24943);
#6648=VERTEX_POINT('',#24945);
#6649=VERTEX_POINT('',#24947);
#6650=VERTEX_POINT('',#24949);
#6651=VERTEX_POINT('',#24951);
#6652=VERTEX_POINT('',#24953);
#6653=VERTEX_POINT('',#24955);
#6654=VERTEX_POINT('',#24957);
#6655=VERTEX_POINT('',#24959);
#6656=VERTEX_POINT('',#24961);
#6657=VERTEX_POINT('',#24963);
#6658=VERTEX_POINT('',#24965);
#6659=VERTEX_POINT('',#24967);
#6660=VERTEX_POINT('',#24969);
#6661=VERTEX_POINT('',#24971);
#6662=VERTEX_POINT('',#24974);
#6663=VERTEX_POINT('',#24977);
#6664=VERTEX_POINT('',#24979);
#6665=VERTEX_POINT('',#24981);
#6666=VERTEX_POINT('',#24988);
#6667=VERTEX_POINT('',#24992);
#6668=VERTEX_POINT('',#24993);
#6669=VERTEX_POINT('',#24997);
#6670=VERTEX_POINT('',#24999);
#6671=VERTEX_POINT('',#25001);
#6672=VERTEX_POINT('',#25007);
#6673=VERTEX_POINT('',#25009);
#6674=VERTEX_POINT('',#25022);
#6675=VERTEX_POINT('',#25026);
#6676=VERTEX_POINT('',#25028);
#6677=VERTEX_POINT('',#25034);
#6678=VERTEX_POINT('',#25035);
#6679=VERTEX_POINT('',#25039);
#6680=VERTEX_POINT('',#25041);
#6681=VERTEX_POINT('',#25043);
#6682=VERTEX_POINT('',#25049);
#6683=VERTEX_POINT('',#25051);
#6684=VERTEX_POINT('',#25064);
#6685=VERTEX_POINT('',#25068);
#6686=VERTEX_POINT('',#25070);
#6687=VERTEX_POINT('',#25076);
#6688=VERTEX_POINT('',#25077);
#6689=VERTEX_POINT('',#25081);
#6690=VERTEX_POINT('',#25083);
#6691=VERTEX_POINT('',#25085);
#6692=VERTEX_POINT('',#25091);
#6693=VERTEX_POINT('',#25093);
#6694=VERTEX_POINT('',#25106);
#6695=VERTEX_POINT('',#25110);
#6696=VERTEX_POINT('',#25114);
#6697=VERTEX_POINT('',#25118);
#6698=VERTEX_POINT('',#25120);
#6699=VERTEX_POINT('',#25130);
#6700=VERTEX_POINT('',#25131);
#6701=VERTEX_POINT('',#25133);
#6702=VERTEX_POINT('',#25135);
#6703=VERTEX_POINT('',#25141);
#6704=VERTEX_POINT('',#25143);
#6705=VERTEX_POINT('',#25156);
#6706=VERTEX_POINT('',#25160);
#6707=VERTEX_POINT('',#25162);
#6708=VERTEX_POINT('',#25168);
#6709=VERTEX_POINT('',#25169);
#6710=VERTEX_POINT('',#25171);
#6711=VERTEX_POINT('',#25173);
#6712=VERTEX_POINT('',#25177);
#6713=VERTEX_POINT('',#25183);
#6714=VERTEX_POINT('',#25185);
#6715=VERTEX_POINT('',#25198);
#6716=VERTEX_POINT('',#25202);
#6717=VERTEX_POINT('',#25204);
#6718=VERTEX_POINT('',#25210);
#6719=VERTEX_POINT('',#25211);
#6720=VERTEX_POINT('',#25213);
#6721=VERTEX_POINT('',#25215);
#6722=VERTEX_POINT('',#25219);
#6723=VERTEX_POINT('',#25225);
#6724=VERTEX_POINT('',#25227);
#6725=VERTEX_POINT('',#25240);
#6726=VERTEX_POINT('',#25244);
#6727=VERTEX_POINT('',#25246);
#6728=VERTEX_POINT('',#25252);
#6729=VERTEX_POINT('',#25253);
#6730=VERTEX_POINT('',#25255);
#6731=VERTEX_POINT('',#25257);
#6732=VERTEX_POINT('',#25261);
#6733=VERTEX_POINT('',#25267);
#6734=VERTEX_POINT('',#25269);
#6735=VERTEX_POINT('',#25282);
#6736=VERTEX_POINT('',#25286);
#6737=VERTEX_POINT('',#25288);
#6738=VERTEX_POINT('',#25294);
#6739=VERTEX_POINT('',#25295);
#6740=VERTEX_POINT('',#25297);
#6741=VERTEX_POINT('',#25299);
#6742=VERTEX_POINT('',#25303);
#6743=VERTEX_POINT('',#25309);
#6744=VERTEX_POINT('',#25311);
#6745=VERTEX_POINT('',#25324);
#6746=VERTEX_POINT('',#25328);
#6747=VERTEX_POINT('',#25330);
#6748=VERTEX_POINT('',#25336);
#6749=VERTEX_POINT('',#25337);
#6750=VERTEX_POINT('',#25339);
#6751=VERTEX_POINT('',#25341);
#6752=VERTEX_POINT('',#25345);
#6753=VERTEX_POINT('',#25351);
#6754=VERTEX_POINT('',#25353);
#6755=VERTEX_POINT('',#25366);
#6756=VERTEX_POINT('',#25370);
#6757=VERTEX_POINT('',#25371);
#6758=VERTEX_POINT('',#25373);
#6759=VERTEX_POINT('',#25375);
#6760=VERTEX_POINT('',#25398);
#6761=VERTEX_POINT('',#25424);
#6762=VERTEX_POINT('',#25425);
#6763=VERTEX_POINT('',#25429);
#6764=VERTEX_POINT('',#25431);
#6765=VERTEX_POINT('',#25433);
#6766=VERTEX_POINT('',#25439);
#6767=VERTEX_POINT('',#25441);
#6768=VERTEX_POINT('',#25454);
#6769=VERTEX_POINT('',#25458);
#6770=VERTEX_POINT('',#25460);
#6771=VERTEX_POINT('',#25466);
#6772=VERTEX_POINT('',#25468);
#6773=VERTEX_POINT('',#25477);
#6774=VERTEX_POINT('',#25479);
#6775=VERTEX_POINT('',#25481);
#6776=VERTEX_POINT('',#25487);
#6777=VERTEX_POINT('',#25489);
#6778=VERTEX_POINT('',#25498);
#6779=VERTEX_POINT('',#25502);
#6780=VERTEX_POINT('',#25504);
#6781=VERTEX_POINT('',#25510);
#6782=VERTEX_POINT('',#25511);
#6783=VERTEX_POINT('',#25515);
#6784=VERTEX_POINT('',#25517);
#6785=VERTEX_POINT('',#25519);
#6786=VERTEX_POINT('',#25525);
#6787=VERTEX_POINT('',#25527);
#6788=VERTEX_POINT('',#25540);
#6789=VERTEX_POINT('',#25544);
#6790=VERTEX_POINT('',#25546);
#6791=VERTEX_POINT('',#25552);
#6792=VERTEX_POINT('',#25553);
#6793=VERTEX_POINT('',#25557);
#6794=VERTEX_POINT('',#25559);
#6795=VERTEX_POINT('',#25561);
#6796=VERTEX_POINT('',#25567);
#6797=VERTEX_POINT('',#25569);
#6798=VERTEX_POINT('',#25582);
#6799=VERTEX_POINT('',#25586);
#6800=VERTEX_POINT('',#25587);
#6801=VERTEX_POINT('',#25591);
#6802=VERTEX_POINT('',#25593);
#6803=VERTEX_POINT('',#25597);
#6804=VERTEX_POINT('',#25599);
#6805=VERTEX_POINT('',#25613);
#6806=VERTEX_POINT('',#25614);
#6807=VERTEX_POINT('',#25616);
#6808=VERTEX_POINT('',#25618);
#6809=VERTEX_POINT('',#25624);
#6810=VERTEX_POINT('',#25626);
#6811=VERTEX_POINT('',#25639);
#6812=VERTEX_POINT('',#25643);
#6813=VERTEX_POINT('',#25645);
#6814=VERTEX_POINT('',#25651);
#6815=VERTEX_POINT('',#25652);
#6816=VERTEX_POINT('',#25654);
#6817=VERTEX_POINT('',#25656);
#6818=VERTEX_POINT('',#25660);
#6819=VERTEX_POINT('',#25666);
#6820=VERTEX_POINT('',#25668);
#6821=VERTEX_POINT('',#25681);
#6822=VERTEX_POINT('',#25685);
#6823=VERTEX_POINT('',#25687);
#6824=VERTEX_POINT('',#25693);
#6825=VERTEX_POINT('',#25694);
#6826=VERTEX_POINT('',#25696);
#6827=VERTEX_POINT('',#25698);
#6828=VERTEX_POINT('',#25702);
#6829=VERTEX_POINT('',#25708);
#6830=VERTEX_POINT('',#25710);
#6831=VERTEX_POINT('',#25723);
#6832=VERTEX_POINT('',#25727);
#6833=VERTEX_POINT('',#25729);
#6834=VERTEX_POINT('',#25735);
#6835=VERTEX_POINT('',#25736);
#6836=VERTEX_POINT('',#25738);
#6837=VERTEX_POINT('',#25740);
#6838=VERTEX_POINT('',#25744);
#6839=VERTEX_POINT('',#25750);
#6840=VERTEX_POINT('',#25752);
#6841=VERTEX_POINT('',#25765);
#6842=VERTEX_POINT('',#25769);
#6843=VERTEX_POINT('',#25771);
#6844=VERTEX_POINT('',#25777);
#6845=VERTEX_POINT('',#25778);
#6846=VERTEX_POINT('',#25780);
#6847=VERTEX_POINT('',#25782);
#6848=VERTEX_POINT('',#25786);
#6849=VERTEX_POINT('',#25792);
#6850=VERTEX_POINT('',#25794);
#6851=VERTEX_POINT('',#25807);
#6852=VERTEX_POINT('',#25811);
#6853=VERTEX_POINT('',#25812);
#6854=VERTEX_POINT('',#25814);
#6855=VERTEX_POINT('',#25816);
#6856=VERTEX_POINT('',#25841);
#6857=VERTEX_POINT('',#25863);
#6858=VERTEX_POINT('',#25864);
#6859=VERTEX_POINT('',#25868);
#6860=VERTEX_POINT('',#25870);
#6861=VERTEX_POINT('',#25872);
#6862=VERTEX_POINT('',#25878);
#6863=VERTEX_POINT('',#25880);
#6864=VERTEX_POINT('',#25893);
#6865=VERTEX_POINT('',#25897);
#6866=VERTEX_POINT('',#25899);
#6867=VERTEX_POINT('',#25905);
#6868=VERTEX_POINT('',#25906);
#6869=VERTEX_POINT('',#25910);
#6870=VERTEX_POINT('',#25912);
#6871=VERTEX_POINT('',#25914);
#6872=VERTEX_POINT('',#25920);
#6873=VERTEX_POINT('',#25922);
#6874=VERTEX_POINT('',#25935);
#6875=VERTEX_POINT('',#25939);
#6876=VERTEX_POINT('',#25941);
#6877=VERTEX_POINT('',#25947);
#6878=VERTEX_POINT('',#25948);
#6879=VERTEX_POINT('',#25952);
#6880=VERTEX_POINT('',#25954);
#6881=VERTEX_POINT('',#25956);
#6882=VERTEX_POINT('',#25962);
#6883=VERTEX_POINT('',#25964);
#6884=VERTEX_POINT('',#25977);
#6885=VERTEX_POINT('',#25981);
#6886=VERTEX_POINT('',#25983);
#6887=VERTEX_POINT('',#25989);
#6888=VERTEX_POINT('',#25990);
#6889=VERTEX_POINT('',#25994);
#6890=VERTEX_POINT('',#25996);
#6891=VERTEX_POINT('',#25998);
#6892=VERTEX_POINT('',#26004);
#6893=VERTEX_POINT('',#26006);
#6894=VERTEX_POINT('',#26019);
#6895=VERTEX_POINT('',#26023);
#6896=VERTEX_POINT('',#26025);
#6897=VERTEX_POINT('',#26031);
#6898=VERTEX_POINT('',#26032);
#6899=VERTEX_POINT('',#26036);
#6900=VERTEX_POINT('',#26038);
#6901=VERTEX_POINT('',#26040);
#6902=VERTEX_POINT('',#26046);
#6903=VERTEX_POINT('',#26048);
#6904=VERTEX_POINT('',#26061);
#6905=VERTEX_POINT('',#26065);
#6906=VERTEX_POINT('',#26066);
#6907=VERTEX_POINT('',#26070);
#6908=VERTEX_POINT('',#26072);
#6909=VERTEX_POINT('',#26076);
#6910=VERTEX_POINT('',#26078);
#6911=VERTEX_POINT('',#26092);
#6912=VERTEX_POINT('',#26093);
#6913=VERTEX_POINT('',#26095);
#6914=VERTEX_POINT('',#26097);
#6915=VERTEX_POINT('',#26103);
#6916=VERTEX_POINT('',#26105);
#6917=VERTEX_POINT('',#26118);
#6918=VERTEX_POINT('',#26122);
#6919=VERTEX_POINT('',#26124);
#6920=VERTEX_POINT('',#26130);
#6921=VERTEX_POINT('',#26131);
#6922=VERTEX_POINT('',#26133);
#6923=VERTEX_POINT('',#26135);
#6924=VERTEX_POINT('',#26139);
#6925=VERTEX_POINT('',#26145);
#6926=VERTEX_POINT('',#26147);
#6927=VERTEX_POINT('',#26160);
#6928=VERTEX_POINT('',#26164);
#6929=VERTEX_POINT('',#26166);
#6930=VERTEX_POINT('',#26172);
#6931=VERTEX_POINT('',#26173);
#6932=VERTEX_POINT('',#26175);
#6933=VERTEX_POINT('',#26177);
#6934=VERTEX_POINT('',#26181);
#6935=VERTEX_POINT('',#26187);
#6936=VERTEX_POINT('',#26189);
#6937=VERTEX_POINT('',#26202);
#6938=VERTEX_POINT('',#26206);
#6939=VERTEX_POINT('',#26208);
#6940=VERTEX_POINT('',#26214);
#6941=VERTEX_POINT('',#26215);
#6942=VERTEX_POINT('',#26217);
#6943=VERTEX_POINT('',#26219);
#6944=VERTEX_POINT('',#26223);
#6945=VERTEX_POINT('',#26229);
#6946=VERTEX_POINT('',#26231);
#6947=VERTEX_POINT('',#26244);
#6948=VERTEX_POINT('',#26248);
#6949=VERTEX_POINT('',#26249);
#6950=VERTEX_POINT('',#26251);
#6951=VERTEX_POINT('',#26253);
#6952=VERTEX_POINT('',#26284);
#6953=VERTEX_POINT('',#26302);
#6954=VERTEX_POINT('',#26303);
#6955=VERTEX_POINT('',#26307);
#6956=VERTEX_POINT('',#26309);
#6957=VERTEX_POINT('',#26311);
#6958=VERTEX_POINT('',#26317);
#6959=VERTEX_POINT('',#26319);
#6960=VERTEX_POINT('',#26332);
#6961=VERTEX_POINT('',#26336);
#6962=VERTEX_POINT('',#26338);
#6963=VERTEX_POINT('',#26344);
#6964=VERTEX_POINT('',#26346);
#6965=VERTEX_POINT('',#26355);
#6966=VERTEX_POINT('',#26357);
#6967=VERTEX_POINT('',#26359);
#6968=VERTEX_POINT('',#26365);
#6969=VERTEX_POINT('',#26367);
#6970=VERTEX_POINT('',#26376);
#6971=VERTEX_POINT('',#26380);
#6972=VERTEX_POINT('',#26382);
#6973=VERTEX_POINT('',#26388);
#6974=VERTEX_POINT('',#26389);
#6975=VERTEX_POINT('',#26393);
#6976=VERTEX_POINT('',#26395);
#6977=VERTEX_POINT('',#26397);
#6978=VERTEX_POINT('',#26403);
#6979=VERTEX_POINT('',#26405);
#6980=VERTEX_POINT('',#26418);
#6981=VERTEX_POINT('',#26422);
#6982=VERTEX_POINT('',#26424);
#6983=VERTEX_POINT('',#26430);
#6984=VERTEX_POINT('',#26431);
#6985=VERTEX_POINT('',#26435);
#6986=VERTEX_POINT('',#26437);
#6987=VERTEX_POINT('',#26439);
#6988=VERTEX_POINT('',#26445);
#6989=VERTEX_POINT('',#26447);
#6990=VERTEX_POINT('',#26460);
#6991=VERTEX_POINT('',#26464);
#6992=VERTEX_POINT('',#26466);
#6993=VERTEX_POINT('',#26472);
#6994=VERTEX_POINT('',#26473);
#6995=VERTEX_POINT('',#26477);
#6996=VERTEX_POINT('',#26479);
#6997=VERTEX_POINT('',#26481);
#6998=VERTEX_POINT('',#26487);
#6999=VERTEX_POINT('',#26489);
#7000=VERTEX_POINT('',#26502);
#7001=VERTEX_POINT('',#26506);
#7002=VERTEX_POINT('',#26508);
#7003=VERTEX_POINT('',#26514);
#7004=VERTEX_POINT('',#26515);
#7005=VERTEX_POINT('',#26519);
#7006=VERTEX_POINT('',#26521);
#7007=VERTEX_POINT('',#26523);
#7008=VERTEX_POINT('',#26529);
#7009=VERTEX_POINT('',#26531);
#7010=VERTEX_POINT('',#26544);
#7011=VERTEX_POINT('',#26548);
#7012=VERTEX_POINT('',#26549);
#7013=VERTEX_POINT('',#26553);
#7014=VERTEX_POINT('',#26555);
#7015=VERTEX_POINT('',#26559);
#7016=VERTEX_POINT('',#26561);
#7017=VERTEX_POINT('',#26575);
#7018=VERTEX_POINT('',#26576);
#7019=VERTEX_POINT('',#26578);
#7020=VERTEX_POINT('',#26580);
#7021=VERTEX_POINT('',#26586);
#7022=VERTEX_POINT('',#26588);
#7023=VERTEX_POINT('',#26601);
#7024=VERTEX_POINT('',#26605);
#7025=VERTEX_POINT('',#26607);
#7026=VERTEX_POINT('',#26613);
#7027=VERTEX_POINT('',#26614);
#7028=VERTEX_POINT('',#26616);
#7029=VERTEX_POINT('',#26618);
#7030=VERTEX_POINT('',#26622);
#7031=VERTEX_POINT('',#26628);
#7032=VERTEX_POINT('',#26630);
#7033=VERTEX_POINT('',#26643);
#7034=VERTEX_POINT('',#26647);
#7035=VERTEX_POINT('',#26649);
#7036=VERTEX_POINT('',#26655);
#7037=VERTEX_POINT('',#26656);
#7038=VERTEX_POINT('',#26658);
#7039=VERTEX_POINT('',#26660);
#7040=VERTEX_POINT('',#26664);
#7041=VERTEX_POINT('',#26670);
#7042=VERTEX_POINT('',#26672);
#7043=VERTEX_POINT('',#26685);
#7044=VERTEX_POINT('',#26689);
#7045=VERTEX_POINT('',#26690);
#7046=VERTEX_POINT('',#26692);
#7047=VERTEX_POINT('',#26694);
#7048=VERTEX_POINT('',#26727);
#7049=VERTEX_POINT('',#26741);
#7050=VERTEX_POINT('',#26742);
#7051=VERTEX_POINT('',#26746);
#7052=VERTEX_POINT('',#26748);
#7053=VERTEX_POINT('',#26750);
#7054=VERTEX_POINT('',#26756);
#7055=VERTEX_POINT('',#26758);
#7056=VERTEX_POINT('',#26771);
#7057=VERTEX_POINT('',#26775);
#7058=VERTEX_POINT('',#26777);
#7059=VERTEX_POINT('',#26783);
#7060=VERTEX_POINT('',#26784);
#7061=VERTEX_POINT('',#26788);
#7062=VERTEX_POINT('',#26790);
#7063=VERTEX_POINT('',#26792);
#7064=VERTEX_POINT('',#26798);
#7065=VERTEX_POINT('',#26800);
#7066=VERTEX_POINT('',#26813);
#7067=VERTEX_POINT('',#26817);
#7068=VERTEX_POINT('',#26819);
#7069=VERTEX_POINT('',#26825);
#7070=VERTEX_POINT('',#26826);
#7071=VERTEX_POINT('',#26830);
#7072=VERTEX_POINT('',#26832);
#7073=VERTEX_POINT('',#26834);
#7074=VERTEX_POINT('',#26840);
#7075=VERTEX_POINT('',#26842);
#7076=VERTEX_POINT('',#26855);
#7077=VERTEX_POINT('',#26859);
#7078=VERTEX_POINT('',#26861);
#7079=VERTEX_POINT('',#26867);
#7080=VERTEX_POINT('',#26868);
#7081=VERTEX_POINT('',#26872);
#7082=VERTEX_POINT('',#26874);
#7083=VERTEX_POINT('',#26876);
#7084=VERTEX_POINT('',#26882);
#7085=VERTEX_POINT('',#26884);
#7086=VERTEX_POINT('',#26897);
#7087=VERTEX_POINT('',#26901);
#7088=VERTEX_POINT('',#26903);
#7089=VERTEX_POINT('',#26909);
#7090=VERTEX_POINT('',#26910);
#7091=VERTEX_POINT('',#26914);
#7092=VERTEX_POINT('',#26916);
#7093=VERTEX_POINT('',#26918);
#7094=VERTEX_POINT('',#26924);
#7095=VERTEX_POINT('',#26926);
#7096=VERTEX_POINT('',#26939);
#7097=VERTEX_POINT('',#26943);
#7098=VERTEX_POINT('',#26945);
#7099=VERTEX_POINT('',#26951);
#7100=VERTEX_POINT('',#26952);
#7101=VERTEX_POINT('',#26956);
#7102=VERTEX_POINT('',#26958);
#7103=VERTEX_POINT('',#26960);
#7104=VERTEX_POINT('',#26966);
#7105=VERTEX_POINT('',#26968);
#7106=VERTEX_POINT('',#26981);
#7107=VERTEX_POINT('',#26985);
#7108=VERTEX_POINT('',#26987);
#7109=VERTEX_POINT('',#26993);
#7110=VERTEX_POINT('',#26994);
#7111=VERTEX_POINT('',#26998);
#7112=VERTEX_POINT('',#27000);
#7113=VERTEX_POINT('',#27002);
#7114=VERTEX_POINT('',#27008);
#7115=VERTEX_POINT('',#27010);
#7116=VERTEX_POINT('',#27023);
#7117=VERTEX_POINT('',#27027);
#7118=VERTEX_POINT('',#27028);
#7119=VERTEX_POINT('',#27032);
#7120=VERTEX_POINT('',#27034);
#7121=VERTEX_POINT('',#27038);
#7122=VERTEX_POINT('',#27040);
#7123=VERTEX_POINT('',#27054);
#7124=VERTEX_POINT('',#27055);
#7125=VERTEX_POINT('',#27057);
#7126=VERTEX_POINT('',#27059);
#7127=VERTEX_POINT('',#27065);
#7128=VERTEX_POINT('',#27067);
#7129=VERTEX_POINT('',#27080);
#7130=VERTEX_POINT('',#27084);
#7131=VERTEX_POINT('',#27086);
#7132=VERTEX_POINT('',#27092);
#7133=VERTEX_POINT('',#27093);
#7134=VERTEX_POINT('',#27095);
#7135=VERTEX_POINT('',#27097);
#7136=VERTEX_POINT('',#27101);
#7137=VERTEX_POINT('',#27107);
#7138=VERTEX_POINT('',#27109);
#7139=VERTEX_POINT('',#27122);
#7140=VERTEX_POINT('',#27126);
#7141=VERTEX_POINT('',#27127);
#7142=VERTEX_POINT('',#27129);
#7143=VERTEX_POINT('',#27131);
#7144=VERTEX_POINT('',#27170);
#7145=VERTEX_POINT('',#27180);
#7146=VERTEX_POINT('',#27181);
#7147=VERTEX_POINT('',#27185);
#7148=VERTEX_POINT('',#27187);
#7149=VERTEX_POINT('',#27189);
#7150=VERTEX_POINT('',#27195);
#7151=VERTEX_POINT('',#27197);
#7152=VERTEX_POINT('',#27210);
#7153=VERTEX_POINT('',#27214);
#7154=VERTEX_POINT('',#27216);
#7155=VERTEX_POINT('',#27222);
#7156=VERTEX_POINT('',#27223);
#7157=VERTEX_POINT('',#27227);
#7158=VERTEX_POINT('',#27229);
#7159=VERTEX_POINT('',#27231);
#7160=VERTEX_POINT('',#27237);
#7161=VERTEX_POINT('',#27239);
#7162=VERTEX_POINT('',#27252);
#7163=VERTEX_POINT('',#27256);
#7164=VERTEX_POINT('',#27258);
#7165=VERTEX_POINT('',#27264);
#7166=VERTEX_POINT('',#27265);
#7167=VERTEX_POINT('',#27269);
#7168=VERTEX_POINT('',#27271);
#7169=VERTEX_POINT('',#27273);
#7170=VERTEX_POINT('',#27279);
#7171=VERTEX_POINT('',#27281);
#7172=VERTEX_POINT('',#27294);
#7173=VERTEX_POINT('',#27298);
#7174=VERTEX_POINT('',#27300);
#7175=VERTEX_POINT('',#27306);
#7176=VERTEX_POINT('',#27307);
#7177=VERTEX_POINT('',#27311);
#7178=VERTEX_POINT('',#27313);
#7179=VERTEX_POINT('',#27315);
#7180=VERTEX_POINT('',#27321);
#7181=VERTEX_POINT('',#27323);
#7182=VERTEX_POINT('',#27336);
#7183=VERTEX_POINT('',#27340);
#7184=VERTEX_POINT('',#27342);
#7185=VERTEX_POINT('',#27348);
#7186=VERTEX_POINT('',#27349);
#7187=VERTEX_POINT('',#27353);
#7188=VERTEX_POINT('',#27355);
#7189=VERTEX_POINT('',#27357);
#7190=VERTEX_POINT('',#27363);
#7191=VERTEX_POINT('',#27365);
#7192=VERTEX_POINT('',#27378);
#7193=VERTEX_POINT('',#27382);
#7194=VERTEX_POINT('',#27384);
#7195=VERTEX_POINT('',#27390);
#7196=VERTEX_POINT('',#27391);
#7197=VERTEX_POINT('',#27395);
#7198=VERTEX_POINT('',#27397);
#7199=VERTEX_POINT('',#27399);
#7200=VERTEX_POINT('',#27405);
#7201=VERTEX_POINT('',#27407);
#7202=VERTEX_POINT('',#27420);
#7203=VERTEX_POINT('',#27424);
#7204=VERTEX_POINT('',#27426);
#7205=VERTEX_POINT('',#27432);
#7206=VERTEX_POINT('',#27433);
#7207=VERTEX_POINT('',#27437);
#7208=VERTEX_POINT('',#27439);
#7209=VERTEX_POINT('',#27441);
#7210=VERTEX_POINT('',#27447);
#7211=VERTEX_POINT('',#27449);
#7212=VERTEX_POINT('',#27462);
#7213=VERTEX_POINT('',#27466);
#7214=VERTEX_POINT('',#27468);
#7215=VERTEX_POINT('',#27474);
#7216=VERTEX_POINT('',#27475);
#7217=VERTEX_POINT('',#27479);
#7218=VERTEX_POINT('',#27481);
#7219=VERTEX_POINT('',#27483);
#7220=VERTEX_POINT('',#27489);
#7221=VERTEX_POINT('',#27491);
#7222=VERTEX_POINT('',#27504);
#7223=VERTEX_POINT('',#27508);
#7224=VERTEX_POINT('',#27509);
#7225=VERTEX_POINT('',#27513);
#7226=VERTEX_POINT('',#27515);
#7227=VERTEX_POINT('',#27519);
#7228=VERTEX_POINT('',#27521);
#7229=VERTEX_POINT('',#27535);
#7230=VERTEX_POINT('',#27536);
#7231=VERTEX_POINT('',#27538);
#7232=VERTEX_POINT('',#27540);
#7233=VERTEX_POINT('',#27546);
#7234=VERTEX_POINT('',#27548);
#7235=VERTEX_POINT('',#27561);
#7236=VERTEX_POINT('',#27565);
#7237=VERTEX_POINT('',#27566);
#7238=VERTEX_POINT('',#27568);
#7239=VERTEX_POINT('',#27570);
#7240=VERTEX_POINT('',#27613);
#7241=VERTEX_POINT('',#27619);
#7242=VERTEX_POINT('',#27620);
#7243=VERTEX_POINT('',#27622);
#7244=VERTEX_POINT('',#27629);
#7245=VERTEX_POINT('',#27631);
#7246=VERTEX_POINT('',#27640);
#7247=VERTEX_POINT('',#27644);
#7248=VERTEX_POINT('',#27646);
#7249=VERTEX_POINT('',#27652);
#7250=VERTEX_POINT('',#27653);
#7251=VERTEX_POINT('',#27655);
#7252=VERTEX_POINT('',#27657);
#7253=VERTEX_POINT('',#27661);
#7254=VERTEX_POINT('',#27667);
#7255=VERTEX_POINT('',#27669);
#7256=VERTEX_POINT('',#27682);
#7257=VERTEX_POINT('',#27686);
#7258=VERTEX_POINT('',#27688);
#7259=VERTEX_POINT('',#27694);
#7260=VERTEX_POINT('',#27695);
#7261=VERTEX_POINT('',#27697);
#7262=VERTEX_POINT('',#27699);
#7263=VERTEX_POINT('',#27703);
#7264=VERTEX_POINT('',#27709);
#7265=VERTEX_POINT('',#27711);
#7266=VERTEX_POINT('',#27724);
#7267=VERTEX_POINT('',#27728);
#7268=VERTEX_POINT('',#27730);
#7269=VERTEX_POINT('',#27736);
#7270=VERTEX_POINT('',#27737);
#7271=VERTEX_POINT('',#27739);
#7272=VERTEX_POINT('',#27741);
#7273=VERTEX_POINT('',#27745);
#7274=VERTEX_POINT('',#27751);
#7275=VERTEX_POINT('',#27753);
#7276=VERTEX_POINT('',#27766);
#7277=VERTEX_POINT('',#27770);
#7278=VERTEX_POINT('',#27772);
#7279=VERTEX_POINT('',#27778);
#7280=VERTEX_POINT('',#27779);
#7281=VERTEX_POINT('',#27781);
#7282=VERTEX_POINT('',#27783);
#7283=VERTEX_POINT('',#27787);
#7284=VERTEX_POINT('',#27793);
#7285=VERTEX_POINT('',#27795);
#7286=VERTEX_POINT('',#27808);
#7287=VERTEX_POINT('',#27812);
#7288=VERTEX_POINT('',#27814);
#7289=VERTEX_POINT('',#27820);
#7290=VERTEX_POINT('',#27821);
#7291=VERTEX_POINT('',#27823);
#7292=VERTEX_POINT('',#27825);
#7293=VERTEX_POINT('',#27829);
#7294=VERTEX_POINT('',#27835);
#7295=VERTEX_POINT('',#27837);
#7296=VERTEX_POINT('',#27850);
#7297=VERTEX_POINT('',#27854);
#7298=VERTEX_POINT('',#27856);
#7299=VERTEX_POINT('',#27862);
#7300=VERTEX_POINT('',#27863);
#7301=VERTEX_POINT('',#27865);
#7302=VERTEX_POINT('',#27867);
#7303=VERTEX_POINT('',#27871);
#7304=VERTEX_POINT('',#27877);
#7305=VERTEX_POINT('',#27879);
#7306=VERTEX_POINT('',#27892);
#7307=VERTEX_POINT('',#27896);
#7308=VERTEX_POINT('',#27898);
#7309=VERTEX_POINT('',#27904);
#7310=VERTEX_POINT('',#27905);
#7311=VERTEX_POINT('',#27907);
#7312=VERTEX_POINT('',#27909);
#7313=VERTEX_POINT('',#27913);
#7314=VERTEX_POINT('',#27919);
#7315=VERTEX_POINT('',#27921);
#7316=VERTEX_POINT('',#27934);
#7317=VERTEX_POINT('',#27938);
#7318=VERTEX_POINT('',#27940);
#7319=VERTEX_POINT('',#27946);
#7320=VERTEX_POINT('',#27947);
#7321=VERTEX_POINT('',#27949);
#7322=VERTEX_POINT('',#27951);
#7323=VERTEX_POINT('',#27955);
#7324=VERTEX_POINT('',#27961);
#7325=VERTEX_POINT('',#27963);
#7326=VERTEX_POINT('',#27976);
#7327=VERTEX_POINT('',#27980);
#7328=VERTEX_POINT('',#27982);
#7329=VERTEX_POINT('',#27988);
#7330=VERTEX_POINT('',#27990);
#7331=VERTEX_POINT('',#28032);
#7332=VERTEX_POINT('',#28036);
#7333=VERTEX_POINT('',#28040);
#7334=VERTEX_POINT('',#28078);
#7335=VERTEX_POINT('',#28080);
#7336=VERTEX_POINT('',#28086);
#7337=VERTEX_POINT('',#28088);
#7338=VERTEX_POINT('',#28095);
#7339=VERTEX_POINT('',#28097);
#7340=VERTEX_POINT('',#28107);
#7341=VERTEX_POINT('',#28109);
#7342=VERTEX_POINT('',#28113);
#7343=VERTEX_POINT('',#28115);
#7344=VERTEX_POINT('',#28122);
#7345=VERTEX_POINT('',#28123);
#7346=VERTEX_POINT('',#28125);
#7347=VERTEX_POINT('',#28127);
#7348=VERTEX_POINT('',#28134);
#7349=VERTEX_POINT('',#28145);
#7350=VERTEX_POINT('',#28149);
#7351=VERTEX_POINT('',#28154);
#7352=VERTEX_POINT('',#28158);
#7353=VERTEX_POINT('',#28160);
#7354=VERTEX_POINT('',#28167);
#7355=VERTEX_POINT('',#28169);
#7356=VERTEX_POINT('',#28179);
#7357=VERTEX_POINT('',#28181);
#7358=VERTEX_POINT('',#28185);
#7359=VERTEX_POINT('',#28187);
#7360=VERTEX_POINT('',#28194);
#7361=VERTEX_POINT('',#28195);
#7362=VERTEX_POINT('',#28197);
#7363=VERTEX_POINT('',#28199);
#7364=VERTEX_POINT('',#28206);
#7365=VERTEX_POINT('',#28217);
#7366=VERTEX_POINT('',#28221);
#7367=VERTEX_POINT('',#28226);
#7368=VERTEX_POINT('',#28230);
#7369=VERTEX_POINT('',#28232);
#7370=VERTEX_POINT('',#28239);
#7371=VERTEX_POINT('',#28241);
#7372=VERTEX_POINT('',#28251);
#7373=VERTEX_POINT('',#28253);
#7374=VERTEX_POINT('',#28257);
#7375=VERTEX_POINT('',#28259);
#7376=VERTEX_POINT('',#28266);
#7377=VERTEX_POINT('',#28268);
#7378=VERTEX_POINT('',#28275);
#7379=VERTEX_POINT('',#28282);
#7380=VERTEX_POINT('',#28286);
#7381=VERTEX_POINT('',#28288);
#7382=VERTEX_POINT('',#28292);
#7383=VERTEX_POINT('',#28295);
#7384=VERTEX_POINT('',#28399);
#7385=VERTEX_POINT('',#28401);
#7386=VERTEX_POINT('',#28405);
#7387=VERTEX_POINT('',#28407);
#7388=VERTEX_POINT('',#28409);
#7389=VERTEX_POINT('',#28411);
#7390=VERTEX_POINT('',#28413);
#7391=VERTEX_POINT('',#28415);
#7392=VERTEX_POINT('',#28418);
#7393=VERTEX_POINT('',#28422);
#7394=VERTEX_POINT('',#28426);
#7395=VERTEX_POINT('',#28430);
#7396=VERTEX_POINT('',#28434);
#7397=VERTEX_POINT('',#28438);
#7398=VERTEX_POINT('',#28442);
#7399=VERTEX_POINT('',#28446);
#7400=VERTEX_POINT('',#28450);
#7401=VERTEX_POINT('',#28454);
#7402=VERTEX_POINT('',#28572);
#7403=VERTEX_POINT('',#28574);
#7404=VERTEX_POINT('',#28577);
#7405=VERTEX_POINT('',#28579);
#7406=VERTEX_POINT('',#28582);
#7407=VERTEX_POINT('',#28584);
#7408=VERTEX_POINT('',#28587);
#7409=VERTEX_POINT('',#28589);
#7410=VERTEX_POINT('',#28592);
#7411=VERTEX_POINT('',#28594);
#7412=VERTEX_POINT('',#28597);
#8042=EDGE_CURVE('',#6339,#6340,#1053,.T.);
#8043=EDGE_CURVE('',#6340,#6341,#4415,.T.);
#8044=EDGE_CURVE('',#6341,#6342,#4416,.F.);
#8045=EDGE_CURVE('',#6342,#6339,#4417,.T.);
#8046=EDGE_CURVE('',#6343,#6340,#1501,.T.);
#8047=EDGE_CURVE('',#6344,#6343,#4418,.T.);
#8048=EDGE_CURVE('',#6341,#6344,#1502,.T.);
#8049=EDGE_CURVE('',#6345,#6339,#431,.T.);
#8050=EDGE_CURVE('',#6345,#6346,#1503,.T.);
#8051=EDGE_CURVE('',#6346,#6347,#432,.T.);
#8052=EDGE_CURVE('',#6343,#6347,#1054,.T.);
#8053=EDGE_CURVE('',#6348,#6349,#1055,.T.);
#8054=EDGE_CURVE('',#6349,#6350,#4419,.T.);
#8055=EDGE_CURVE('',#6350,#6351,#4420,.F.);
#8056=EDGE_CURVE('',#6351,#6352,#4421,.T.);
#8057=EDGE_CURVE('',#6352,#6348,#1056,.T.);
#8058=EDGE_CURVE('',#6353,#6349,#1504,.T.);
#8059=EDGE_CURVE('',#6354,#6353,#4422,.T.);
#8060=EDGE_CURVE('',#6350,#6354,#1505,.T.);
#8061=EDGE_CURVE('',#6348,#6355,#433,.T.);
#8062=EDGE_CURVE('',#6355,#6356,#1506,.T.);
#8063=EDGE_CURVE('',#6357,#6356,#434,.T.);
#8064=EDGE_CURVE('',#6353,#6357,#1057,.T.);
#8065=EDGE_CURVE('',#6354,#6358,#4423,.T.);
#8066=EDGE_CURVE('',#6357,#6358,#4424,.T.);
#8067=EDGE_CURVE('',#6359,#6356,#1507,.T.);
#8068=EDGE_CURVE('',#6359,#6360,#435,.T.);
#8069=EDGE_CURVE('',#6361,#6360,#4425,.T.);
#8070=EDGE_CURVE('',#6361,#6358,#1508,.T.);
#8071=EDGE_CURVE('',#6362,#6363,#1058,.T.);
#8072=EDGE_CURVE('',#6363,#6364,#4426,.T.);
#8073=EDGE_CURVE('',#6364,#6365,#4427,.F.);
#8074=EDGE_CURVE('',#6365,#6366,#4428,.T.);
#8075=EDGE_CURVE('',#6366,#6362,#1059,.T.);
#8076=EDGE_CURVE('',#6366,#6367,#1509,.T.);
#8077=EDGE_CURVE('',#6368,#6367,#1060,.T.);
#8078=EDGE_CURVE('',#6368,#6369,#436,.T.);
#8079=EDGE_CURVE('',#6369,#6370,#1510,.T.);
#8080=EDGE_CURVE('',#6362,#6370,#437,.T.);
#8081=EDGE_CURVE('',#6365,#6371,#1511,.T.);
#8082=EDGE_CURVE('',#6367,#6371,#4429,.T.);
#8083=EDGE_CURVE('',#6372,#6373,#4430,.T.);
#8084=EDGE_CURVE('',#6372,#6374,#4431,.T.);
#8085=EDGE_CURVE('',#6374,#6375,#1061,.T.);
#8086=EDGE_CURVE('',#6375,#6376,#1062,.T.);
#8087=EDGE_CURVE('',#6376,#6373,#4432,.T.);
#8088=EDGE_CURVE('',#6351,#6373,#1512,.T.);
#8089=EDGE_CURVE('',#6352,#6376,#1513,.T.);
#8090=EDGE_CURVE('',#6375,#6377,#438,.T.);
#8091=EDGE_CURVE('',#6377,#6355,#1514,.T.);
#8092=EDGE_CURVE('',#6378,#6379,#1063,.T.);
#8093=EDGE_CURVE('',#6379,#6380,#4433,.T.);
#8094=EDGE_CURVE('',#6380,#6381,#4434,.F.);
#8095=EDGE_CURVE('',#6381,#6382,#4435,.T.);
#8096=EDGE_CURVE('',#6382,#6378,#1064,.T.);
#8097=EDGE_CURVE('',#6382,#6383,#1515,.T.);
#8098=EDGE_CURVE('',#6384,#6383,#1065,.T.);
#8099=EDGE_CURVE('',#6384,#6385,#439,.T.);
#8100=EDGE_CURVE('',#6385,#6386,#1516,.T.);
#8101=EDGE_CURVE('',#6378,#6386,#440,.T.);
#8102=EDGE_CURVE('',#6381,#6387,#1517,.T.);
#8103=EDGE_CURVE('',#6383,#6387,#4436,.T.);
#8104=EDGE_CURVE('',#6388,#6371,#4437,.T.);
#8105=EDGE_CURVE('',#6388,#6389,#4438,.T.);
#8106=EDGE_CURVE('',#6389,#6368,#1066,.T.);
#8107=EDGE_CURVE('',#6390,#6387,#4439,.T.);
#8108=EDGE_CURVE('',#6390,#6391,#4440,.T.);
#8109=EDGE_CURVE('',#6391,#6384,#1067,.T.);
#8110=EDGE_CURVE('',#6392,#6393,#4441,.T.);
#8111=EDGE_CURVE('',#6392,#6394,#4442,.T.);
#8112=EDGE_CURVE('',#6394,#6395,#1068,.T.);
#8113=EDGE_CURVE('',#6395,#6393,#4443,.T.);
#8114=EDGE_CURVE('',#6395,#6396,#441,.T.);
#8115=EDGE_CURVE('',#6397,#6396,#1518,.T.);
#8116=EDGE_CURVE('',#6398,#6397,#442,.T.);
#8117=EDGE_CURVE('',#6399,#6398,#4444,.T.);
#8118=EDGE_CURVE('',#6399,#6393,#1519,.T.);
#8119=EDGE_CURVE('',#6394,#6400,#1520,.T.);
#8120=EDGE_CURVE('',#6400,#6401,#443,.T.);
#8121=EDGE_CURVE('',#6401,#6402,#444,.T.);
#8122=EDGE_CURVE('',#6402,#6396,#1521,.T.);
#8123=EDGE_CURVE('',#6403,#6404,#1069,.T.);
#8124=EDGE_CURVE('',#6404,#6405,#4445,.T.);
#8125=EDGE_CURVE('',#6405,#6406,#4446,.F.);
#8126=EDGE_CURVE('',#6406,#6407,#4447,.T.);
#8127=EDGE_CURVE('',#6407,#6403,#1070,.T.);
#8128=EDGE_CURVE('',#6408,#6404,#1522,.T.);
#8129=EDGE_CURVE('',#6409,#6408,#4448,.T.);
#8130=EDGE_CURVE('',#6405,#6409,#1523,.T.);
#8131=EDGE_CURVE('',#6403,#6410,#445,.T.);
#8132=EDGE_CURVE('',#6410,#6411,#1524,.T.);
#8133=EDGE_CURVE('',#6411,#6412,#446,.T.);
#8134=EDGE_CURVE('',#6408,#6412,#447,.T.);
#8135=EDGE_CURVE('',#6413,#6414,#4449,.T.);
#8136=EDGE_CURVE('',#6413,#6415,#4450,.T.);
#8137=EDGE_CURVE('',#6415,#6416,#1071,.T.);
#8138=EDGE_CURVE('',#6416,#6417,#1072,.T.);
#8139=EDGE_CURVE('',#6417,#6414,#4451,.T.);
#8140=EDGE_CURVE('',#6415,#6418,#1525,.T.);
#8141=EDGE_CURVE('',#6419,#6418,#1073,.T.);
#8142=EDGE_CURVE('',#6419,#6420,#448,.T.);
#8143=EDGE_CURVE('',#6420,#6421,#1526,.T.);
#8144=EDGE_CURVE('',#6416,#6421,#449,.T.);
#8145=EDGE_CURVE('',#6422,#6413,#1527,.T.);
#8146=EDGE_CURVE('',#6418,#6422,#4452,.T.);
#8147=EDGE_CURVE('',#6422,#6423,#4453,.F.);
#8148=EDGE_CURVE('',#6423,#6424,#4454,.T.);
#8149=EDGE_CURVE('',#6424,#6419,#1074,.T.);
#8150=EDGE_CURVE('',#6425,#6426,#4455,.T.);
#8151=EDGE_CURVE('',#6425,#6427,#4456,.T.);
#8152=EDGE_CURVE('',#6427,#6428,#1075,.T.);
#8153=EDGE_CURVE('',#6428,#6429,#1076,.T.);
#8154=EDGE_CURVE('',#6429,#6426,#4457,.T.);
#8155=EDGE_CURVE('',#6427,#6430,#1528,.T.);
#8156=EDGE_CURVE('',#6431,#6430,#1077,.T.);
#8157=EDGE_CURVE('',#6431,#6432,#450,.T.);
#8158=EDGE_CURVE('',#6432,#6433,#1529,.T.);
#8159=EDGE_CURVE('',#6428,#6433,#451,.T.);
#8160=EDGE_CURVE('',#6434,#6425,#1530,.T.);
#8161=EDGE_CURVE('',#6430,#6434,#4458,.T.);
#8162=EDGE_CURVE('',#6434,#6435,#4459,.F.);
#8163=EDGE_CURVE('',#6435,#6436,#4460,.T.);
#8164=EDGE_CURVE('',#6436,#6431,#1078,.T.);
#8165=EDGE_CURVE('',#6437,#6438,#4461,.T.);
#8166=EDGE_CURVE('',#6437,#6439,#4462,.T.);
#8167=EDGE_CURVE('',#6439,#6440,#1079,.T.);
#8168=EDGE_CURVE('',#6440,#6441,#1080,.T.);
#8169=EDGE_CURVE('',#6441,#6438,#4463,.T.);
#8170=EDGE_CURVE('',#6439,#6442,#1531,.T.);
#8171=EDGE_CURVE('',#6443,#6442,#1081,.T.);
#8172=EDGE_CURVE('',#6443,#6444,#452,.T.);
#8173=EDGE_CURVE('',#6444,#6445,#1532,.T.);
#8174=EDGE_CURVE('',#6440,#6445,#453,.T.);
#8175=EDGE_CURVE('',#6446,#6437,#1533,.T.);
#8176=EDGE_CURVE('',#6442,#6446,#4464,.T.);
#8177=EDGE_CURVE('',#6446,#6447,#4465,.F.);
#8178=EDGE_CURVE('',#6447,#6448,#4466,.T.);
#8179=EDGE_CURVE('',#6448,#6443,#1082,.T.);
#8180=EDGE_CURVE('',#6449,#6450,#4467,.T.);
#8181=EDGE_CURVE('',#6449,#6451,#4468,.T.);
#8182=EDGE_CURVE('',#6451,#6452,#1083,.T.);
#8183=EDGE_CURVE('',#6452,#6453,#1084,.T.);
#8184=EDGE_CURVE('',#6453,#6450,#4469,.T.);
#8185=EDGE_CURVE('',#6451,#6454,#1534,.T.);
#8186=EDGE_CURVE('',#6455,#6454,#1085,.T.);
#8187=EDGE_CURVE('',#6455,#6456,#454,.T.);
#8188=EDGE_CURVE('',#6456,#6457,#1535,.T.);
#8189=EDGE_CURVE('',#6452,#6457,#455,.T.);
#8190=EDGE_CURVE('',#6458,#6449,#1536,.T.);
#8191=EDGE_CURVE('',#6454,#6458,#4470,.T.);
#8192=EDGE_CURVE('',#6458,#6459,#4471,.F.);
#8193=EDGE_CURVE('',#6459,#6460,#4472,.T.);
#8194=EDGE_CURVE('',#6460,#6455,#1086,.T.);
#8195=EDGE_CURVE('',#6461,#6462,#4473,.T.);
#8196=EDGE_CURVE('',#6461,#6463,#4474,.T.);
#8197=EDGE_CURVE('',#6463,#6464,#1087,.T.);
#8198=EDGE_CURVE('',#6464,#6465,#1088,.T.);
#8199=EDGE_CURVE('',#6465,#6462,#4475,.T.);
#8200=EDGE_CURVE('',#6463,#6466,#1537,.T.);
#8201=EDGE_CURVE('',#6467,#6466,#1089,.T.);
#8202=EDGE_CURVE('',#6467,#6468,#456,.T.);
#8203=EDGE_CURVE('',#6468,#6469,#1538,.T.);
#8204=EDGE_CURVE('',#6464,#6469,#457,.T.);
#8205=EDGE_CURVE('',#6470,#6461,#1539,.T.);
#8206=EDGE_CURVE('',#6466,#6470,#4476,.T.);
#8207=EDGE_CURVE('',#6470,#6471,#4477,.F.);
#8208=EDGE_CURVE('',#6471,#6472,#4478,.T.);
#8209=EDGE_CURVE('',#6472,#6467,#1090,.T.);
#8210=EDGE_CURVE('',#6473,#6474,#4479,.T.);
#8211=EDGE_CURVE('',#6473,#6475,#4480,.T.);
#8212=EDGE_CURVE('',#6475,#6476,#1091,.T.);
#8213=EDGE_CURVE('',#6476,#6477,#1092,.T.);
#8214=EDGE_CURVE('',#6477,#6474,#4481,.T.);
#8215=EDGE_CURVE('',#6475,#6478,#1540,.T.);
#8216=EDGE_CURVE('',#6479,#6478,#1093,.T.);
#8217=EDGE_CURVE('',#6479,#6480,#458,.T.);
#8218=EDGE_CURVE('',#6480,#6481,#1541,.T.);
#8219=EDGE_CURVE('',#6476,#6481,#459,.T.);
#8220=EDGE_CURVE('',#6482,#6473,#1542,.T.);
#8221=EDGE_CURVE('',#6478,#6482,#4482,.T.);
#8222=EDGE_CURVE('',#6482,#6483,#4483,.F.);
#8223=EDGE_CURVE('',#6483,#6484,#4484,.T.);
#8224=EDGE_CURVE('',#6484,#6479,#1094,.T.);
#8225=EDGE_CURVE('',#6485,#6486,#4485,.T.);
#8226=EDGE_CURVE('',#6485,#6487,#4486,.T.);
#8227=EDGE_CURVE('',#6487,#6488,#1095,.T.);
#8228=EDGE_CURVE('',#6488,#6489,#1096,.T.);
#8229=EDGE_CURVE('',#6489,#6486,#4487,.T.);
#8230=EDGE_CURVE('',#6487,#6490,#1543,.T.);
#8231=EDGE_CURVE('',#6491,#6490,#1097,.T.);
#8232=EDGE_CURVE('',#6491,#6492,#460,.T.);
#8233=EDGE_CURVE('',#6492,#6493,#1544,.T.);
#8234=EDGE_CURVE('',#6488,#6493,#461,.T.);
#8235=EDGE_CURVE('',#6494,#6485,#1545,.T.);
#8236=EDGE_CURVE('',#6490,#6494,#4488,.T.);
#8237=EDGE_CURVE('',#6494,#6495,#4489,.F.);
#8238=EDGE_CURVE('',#6495,#6496,#4490,.T.);
#8239=EDGE_CURVE('',#6496,#6491,#1098,.T.);
#8240=EDGE_CURVE('',#6497,#6498,#4491,.T.);
#8241=EDGE_CURVE('',#6497,#6499,#4492,.T.);
#8242=EDGE_CURVE('',#6499,#6500,#1099,.T.);
#8243=EDGE_CURVE('',#6500,#6501,#1100,.T.);
#8244=EDGE_CURVE('',#6501,#6498,#4493,.T.);
#8245=EDGE_CURVE('',#6499,#6502,#1546,.T.);
#8246=EDGE_CURVE('',#6503,#6502,#1101,.T.);
#8247=EDGE_CURVE('',#6503,#6504,#462,.T.);
#8248=EDGE_CURVE('',#6504,#6505,#1547,.T.);
#8249=EDGE_CURVE('',#6500,#6505,#463,.T.);
#8250=EDGE_CURVE('',#6506,#6497,#1548,.T.);
#8251=EDGE_CURVE('',#6502,#6506,#4494,.T.);
#8252=EDGE_CURVE('',#6506,#6507,#4495,.F.);
#8253=EDGE_CURVE('',#6507,#6508,#4496,.T.);
#8254=EDGE_CURVE('',#6508,#6503,#1102,.T.);
#8255=EDGE_CURVE('',#6508,#6509,#1549,.T.);
#8256=EDGE_CURVE('',#6510,#6509,#1103,.T.);
#8257=EDGE_CURVE('',#6511,#6510,#464,.T.);
#8258=EDGE_CURVE('',#6511,#6504,#1550,.T.);
#8259=EDGE_CURVE('',#6370,#6377,#1551,.T.);
#8260=EDGE_CURVE('',#6374,#6363,#1552,.T.);
#8261=EDGE_CURVE('',#6386,#6369,#1553,.T.);
#8262=EDGE_CURVE('',#6389,#6379,#1554,.T.);
#8263=EDGE_CURVE('',#6391,#6512,#1555,.T.);
#8264=EDGE_CURVE('',#6512,#6513,#1104,.T.);
#8265=EDGE_CURVE('',#6514,#6513,#465,.T.);
#8266=EDGE_CURVE('',#6514,#6385,#1556,.T.);
#8267=EDGE_CURVE('',#6514,#6515,#1557,.T.);
#8268=EDGE_CURVE('',#6516,#6515,#1558,.T.);
#8269=EDGE_CURVE('',#6516,#6517,#1559,.T.);
#8270=EDGE_CURVE('',#6518,#6517,#1560,.T.);
#8271=EDGE_CURVE('',#6518,#6519,#1561,.T.);
#8272=EDGE_CURVE('',#6520,#6519,#1562,.T.);
#8273=EDGE_CURVE('',#6520,#6521,#1563,.T.);
#8274=EDGE_CURVE('',#6522,#6521,#1564,.T.);
#8275=EDGE_CURVE('',#6522,#6523,#1565,.T.);
#8276=EDGE_CURVE('',#6524,#6523,#1566,.T.);
#8277=EDGE_CURVE('',#6524,#6525,#1567,.T.);
#8278=EDGE_CURVE('',#6397,#6525,#1568,.T.);
#8279=EDGE_CURVE('',#6402,#6411,#1569,.T.);
#8280=EDGE_CURVE('',#6421,#6410,#1570,.T.);
#8281=EDGE_CURVE('',#6433,#6420,#1571,.T.);
#8282=EDGE_CURVE('',#6445,#6432,#1572,.T.);
#8283=EDGE_CURVE('',#6457,#6444,#1573,.T.);
#8284=EDGE_CURVE('',#6469,#6456,#1574,.T.);
#8285=EDGE_CURVE('',#6481,#6468,#1575,.T.);
#8286=EDGE_CURVE('',#6493,#6480,#1576,.T.);
#8287=EDGE_CURVE('',#6505,#6492,#1577,.T.);
#8288=EDGE_CURVE('',#6526,#6511,#1578,.T.);
#8289=EDGE_CURVE('',#6527,#6526,#1579,.T.);
#8290=EDGE_CURVE('',#6528,#6527,#1580,.T.);
#8291=EDGE_CURVE('',#6529,#6528,#1581,.T.);
#8292=EDGE_CURVE('',#6530,#6529,#1582,.T.);
#8293=EDGE_CURVE('',#6531,#6530,#1583,.T.);
#8294=EDGE_CURVE('',#6532,#6531,#1584,.T.);
#8295=EDGE_CURVE('',#6533,#6532,#1585,.T.);
#8296=EDGE_CURVE('',#6534,#6533,#1586,.T.);
#8297=EDGE_CURVE('',#6535,#6534,#1587,.T.);
#8298=EDGE_CURVE('',#6536,#6535,#1588,.T.);
#8299=EDGE_CURVE('',#6537,#6536,#1589,.T.);
#8300=EDGE_CURVE('',#6538,#6537,#1590,.T.);
#8301=EDGE_CURVE('',#6539,#6538,#1591,.T.);
#8302=EDGE_CURVE('',#6540,#6539,#1592,.T.);
#8303=EDGE_CURVE('',#6541,#6540,#1593,.T.);
#8304=EDGE_CURVE('',#6542,#6541,#1594,.T.);
#8305=EDGE_CURVE('',#6346,#6542,#1595,.T.);
#8306=EDGE_CURVE('',#6345,#6543,#1596,.T.);
#8307=EDGE_CURVE('',#6544,#6543,#1597,.T.);
#8308=EDGE_CURVE('',#6544,#6545,#1598,.T.);
#8309=EDGE_CURVE('',#6546,#6545,#1599,.T.);
#8310=EDGE_CURVE('',#6547,#6546,#1600,.T.);
#8311=EDGE_CURVE('',#6548,#6547,#1601,.T.);
#8312=EDGE_CURVE('',#6549,#6548,#1602,.T.);
#8313=EDGE_CURVE('',#6550,#6549,#1603,.T.);
#8314=EDGE_CURVE('',#6551,#6550,#1604,.T.);
#8315=EDGE_CURVE('',#6552,#6551,#1605,.T.);
#8316=EDGE_CURVE('',#6553,#6552,#1606,.T.);
#8317=EDGE_CURVE('',#6554,#6553,#1607,.T.);
#8318=EDGE_CURVE('',#6555,#6554,#1608,.T.);
#8319=EDGE_CURVE('',#6556,#6555,#1609,.T.);
#8320=EDGE_CURVE('',#6557,#6556,#1610,.T.);
#8321=EDGE_CURVE('',#6558,#6557,#1611,.T.);
#8322=EDGE_CURVE('',#6559,#6558,#1612,.T.);
#8323=EDGE_CURVE('',#6560,#6559,#1613,.T.);
#8324=EDGE_CURVE('',#6561,#6560,#1614,.T.);
#8325=EDGE_CURVE('',#6562,#6561,#1615,.T.);
#8326=EDGE_CURVE('',#6562,#6563,#1616,.T.);
#8327=EDGE_CURVE('',#6564,#6563,#1617,.T.);
#8328=EDGE_CURVE('',#6565,#6564,#1618,.T.);
#8329=EDGE_CURVE('',#6566,#6565,#1619,.T.);
#8330=EDGE_CURVE('',#6566,#6567,#1620,.T.);
#8331=EDGE_CURVE('',#6568,#6567,#1621,.T.);
#8332=EDGE_CURVE('',#6569,#6568,#1622,.T.);
#8333=EDGE_CURVE('',#6570,#6569,#1623,.T.);
#8334=EDGE_CURVE('',#6571,#6570,#1624,.T.);
#8335=EDGE_CURVE('',#6572,#6571,#1625,.T.);
#8336=EDGE_CURVE('',#6573,#6572,#1626,.T.);
#8337=EDGE_CURVE('',#6574,#6573,#1627,.T.);
#8338=EDGE_CURVE('',#6575,#6574,#1628,.T.);
#8339=EDGE_CURVE('',#6576,#6575,#1629,.T.);
#8340=EDGE_CURVE('',#6577,#6576,#1630,.T.);
#8341=EDGE_CURVE('',#6578,#6577,#1631,.T.);
#8342=EDGE_CURVE('',#6579,#6578,#1632,.T.);
#8343=EDGE_CURVE('',#6580,#6579,#1633,.T.);
#8344=EDGE_CURVE('',#6581,#6580,#1634,.T.);
#8345=EDGE_CURVE('',#6582,#6581,#1635,.T.);
#8346=EDGE_CURVE('',#6582,#6583,#1636,.T.);
#8347=EDGE_CURVE('',#6584,#6583,#1637,.T.);
#8348=EDGE_CURVE('',#6585,#6584,#1638,.T.);
#8349=EDGE_CURVE('',#6586,#6585,#1639,.T.);
#8350=EDGE_CURVE('',#6587,#6586,#1640,.T.);
#8351=EDGE_CURVE('',#6588,#6587,#1641,.T.);
#8352=EDGE_CURVE('',#6588,#6589,#1642,.T.);
#8353=EDGE_CURVE('',#6590,#6589,#1643,.T.);
#8354=EDGE_CURVE('',#6591,#6590,#1644,.T.);
#8355=EDGE_CURVE('',#6592,#6591,#1645,.T.);
#8356=EDGE_CURVE('',#6593,#6592,#1646,.T.);
#8357=EDGE_CURVE('',#6594,#6593,#1647,.T.);
#8358=EDGE_CURVE('',#6595,#6594,#1648,.T.);
#8359=EDGE_CURVE('',#6596,#6595,#1649,.T.);
#8360=EDGE_CURVE('',#6597,#6596,#1650,.T.);
#8361=EDGE_CURVE('',#6598,#6597,#1651,.T.);
#8362=EDGE_CURVE('',#6599,#6598,#1652,.T.);
#8363=EDGE_CURVE('',#6600,#6599,#1653,.T.);
#8364=EDGE_CURVE('',#6601,#6600,#1654,.T.);
#8365=EDGE_CURVE('',#6602,#6601,#1655,.T.);
#8366=EDGE_CURVE('',#6602,#6603,#1656,.T.);
#8367=EDGE_CURVE('',#6604,#6603,#1657,.T.);
#8368=EDGE_CURVE('',#6605,#6604,#1658,.T.);
#8369=EDGE_CURVE('',#6606,#6605,#1659,.T.);
#8370=EDGE_CURVE('',#6607,#6606,#1660,.T.);
#8371=EDGE_CURVE('',#6608,#6607,#1661,.T.);
#8372=EDGE_CURVE('',#6609,#6608,#1662,.T.);
#8373=EDGE_CURVE('',#6610,#6609,#1663,.T.);
#8374=EDGE_CURVE('',#6610,#6611,#1664,.T.);
#8375=EDGE_CURVE('',#6612,#6611,#1665,.T.);
#8376=EDGE_CURVE('',#6613,#6612,#1666,.T.);
#8377=EDGE_CURVE('',#6614,#6613,#1667,.T.);
#8378=EDGE_CURVE('',#6615,#6614,#1668,.T.);
#8379=EDGE_CURVE('',#6616,#6615,#1669,.T.);
#8380=EDGE_CURVE('',#6617,#6616,#1670,.T.);
#8381=EDGE_CURVE('',#6618,#6617,#1671,.T.);
#8382=EDGE_CURVE('',#6619,#6618,#1672,.T.);
#8383=EDGE_CURVE('',#6620,#6619,#1673,.T.);
#8384=EDGE_CURVE('',#6621,#6620,#1674,.T.);
#8385=EDGE_CURVE('',#6622,#6621,#1675,.T.);
#8386=EDGE_CURVE('',#6622,#6623,#1676,.T.);
#8387=EDGE_CURVE('',#6624,#6623,#1677,.T.);
#8388=EDGE_CURVE('',#6625,#6624,#1678,.T.);
#8389=EDGE_CURVE('',#6626,#6625,#1679,.T.);
#8390=EDGE_CURVE('',#6627,#6626,#1680,.T.);
#8391=EDGE_CURVE('',#6628,#6627,#1681,.T.);
#8392=EDGE_CURVE('',#6629,#6628,#1682,.T.);
#8393=EDGE_CURVE('',#6630,#6629,#1683,.T.);
#8394=EDGE_CURVE('',#6631,#6630,#1684,.T.);
#8395=EDGE_CURVE('',#6632,#6631,#1685,.T.);
#8396=EDGE_CURVE('',#6632,#6633,#1686,.T.);
#8397=EDGE_CURVE('',#6634,#6633,#1687,.T.);
#8398=EDGE_CURVE('',#6635,#6634,#1688,.T.);
#8399=EDGE_CURVE('',#6636,#6635,#1689,.T.);
#8400=EDGE_CURVE('',#6637,#6636,#1690,.T.);
#8401=EDGE_CURVE('',#6638,#6637,#1691,.T.);
#8402=EDGE_CURVE('',#6639,#6638,#1692,.T.);
#8403=EDGE_CURVE('',#6640,#6639,#1693,.T.);
#8404=EDGE_CURVE('',#6641,#6640,#1694,.T.);
#8405=EDGE_CURVE('',#6642,#6641,#1695,.T.);
#8406=EDGE_CURVE('',#6642,#6643,#1696,.T.);
#8407=EDGE_CURVE('',#6644,#6643,#1697,.T.);
#8408=EDGE_CURVE('',#6645,#6644,#1698,.T.);
#8409=EDGE_CURVE('',#6646,#6645,#1699,.T.);
#8410=EDGE_CURVE('',#6647,#6646,#1700,.T.);
#8411=EDGE_CURVE('',#6648,#6647,#1701,.T.);
#8412=EDGE_CURVE('',#6649,#6648,#1702,.T.);
#8413=EDGE_CURVE('',#6650,#6649,#1703,.T.);
#8414=EDGE_CURVE('',#6651,#6650,#1704,.T.);
#8415=EDGE_CURVE('',#6652,#6651,#1705,.T.);
#8416=EDGE_CURVE('',#6653,#6652,#1706,.T.);
#8417=EDGE_CURVE('',#6654,#6653,#1707,.T.);
#8418=EDGE_CURVE('',#6654,#6655,#1708,.T.);
#8419=EDGE_CURVE('',#6656,#6655,#1709,.T.);
#8420=EDGE_CURVE('',#6657,#6656,#1710,.T.);
#8421=EDGE_CURVE('',#6658,#6657,#1711,.T.);
#8422=EDGE_CURVE('',#6659,#6658,#1712,.T.);
#8423=EDGE_CURVE('',#6660,#6659,#1713,.T.);
#8424=EDGE_CURVE('',#6661,#6660,#1714,.T.);
#8425=EDGE_CURVE('',#6359,#6661,#1715,.T.);
#8426=EDGE_CURVE('',#6662,#6662,#1716,.T.);
#8427=EDGE_CURVE('',#6663,#6513,#4497,.T.);
#8428=EDGE_CURVE('',#6663,#6664,#1717,.T.);
#8429=EDGE_CURVE('',#6665,#6664,#4498,.T.);
#8430=EDGE_CURVE('',#6515,#6665,#466,.T.);
#8431=EDGE_CURVE('',#6512,#6666,#4499,.T.);
#8432=EDGE_CURVE('',#6666,#6663,#4500,.F.);
#8433=EDGE_CURVE('',#6667,#6668,#1105,.T.);
#8434=EDGE_CURVE('',#6668,#6669,#4501,.T.);
#8435=EDGE_CURVE('',#6669,#6670,#4502,.F.);
#8436=EDGE_CURVE('',#6670,#6671,#4503,.T.);
#8437=EDGE_CURVE('',#6671,#6667,#1106,.T.);
#8438=EDGE_CURVE('',#6671,#6672,#1718,.T.);
#8439=EDGE_CURVE('',#6673,#6672,#1107,.T.);
#8440=EDGE_CURVE('',#6673,#6657,#467,.T.);
#8441=EDGE_CURVE('',#6667,#6656,#468,.T.);
#8442=EDGE_CURVE('',#6670,#6674,#1719,.T.);
#8443=EDGE_CURVE('',#6672,#6674,#4504,.T.);
#8444=EDGE_CURVE('',#6675,#6674,#4505,.T.);
#8445=EDGE_CURVE('',#6675,#6676,#4506,.T.);
#8446=EDGE_CURVE('',#6676,#6673,#1108,.T.);
#8447=EDGE_CURVE('',#6677,#6678,#1109,.T.);
#8448=EDGE_CURVE('',#6678,#6679,#4507,.T.);
#8449=EDGE_CURVE('',#6679,#6680,#4508,.F.);
#8450=EDGE_CURVE('',#6680,#6681,#4509,.T.);
#8451=EDGE_CURVE('',#6681,#6677,#1110,.T.);
#8452=EDGE_CURVE('',#6681,#6682,#1720,.T.);
#8453=EDGE_CURVE('',#6683,#6682,#1111,.T.);
#8454=EDGE_CURVE('',#6683,#6659,#469,.T.);
#8455=EDGE_CURVE('',#6677,#6658,#470,.T.);
#8456=EDGE_CURVE('',#6680,#6684,#1721,.T.);
#8457=EDGE_CURVE('',#6682,#6684,#4510,.T.);
#8458=EDGE_CURVE('',#6685,#6684,#4511,.T.);
#8459=EDGE_CURVE('',#6685,#6686,#4512,.T.);
#8460=EDGE_CURVE('',#6686,#6683,#1112,.T.);
#8461=EDGE_CURVE('',#6687,#6688,#1113,.T.);
#8462=EDGE_CURVE('',#6688,#6689,#4513,.T.);
#8463=EDGE_CURVE('',#6689,#6690,#4514,.F.);
#8464=EDGE_CURVE('',#6690,#6691,#4515,.T.);
#8465=EDGE_CURVE('',#6691,#6687,#1114,.T.);
#8466=EDGE_CURVE('',#6691,#6692,#1722,.T.);
#8467=EDGE_CURVE('',#6693,#6692,#1115,.T.);
#8468=EDGE_CURVE('',#6693,#6661,#471,.T.);
#8469=EDGE_CURVE('',#6687,#6660,#472,.T.);
#8470=EDGE_CURVE('',#6690,#6694,#1723,.T.);
#8471=EDGE_CURVE('',#6692,#6694,#4516,.T.);
#8472=EDGE_CURVE('',#6360,#6695,#1116,.T.);
#8473=EDGE_CURVE('',#6695,#6696,#4517,.T.);
#8474=EDGE_CURVE('',#6696,#6361,#4518,.F.);
#8475=EDGE_CURVE('',#6697,#6695,#1724,.T.);
#8476=EDGE_CURVE('',#6698,#6697,#4519,.T.);
#8477=EDGE_CURVE('',#6696,#6698,#1725,.T.);
#8478=EDGE_CURVE('',#6697,#6693,#1117,.T.);
#8479=EDGE_CURVE('',#6698,#6694,#4520,.T.);
#8480=EDGE_CURVE('',#6699,#6700,#4521,.T.);
#8481=EDGE_CURVE('',#6699,#6701,#4522,.T.);
#8482=EDGE_CURVE('',#6701,#6702,#1118,.T.);
#8483=EDGE_CURVE('',#6702,#6700,#4523,.T.);
#8484=EDGE_CURVE('',#6701,#6703,#1726,.T.);
#8485=EDGE_CURVE('',#6704,#6703,#1119,.T.);
#8486=EDGE_CURVE('',#6704,#6644,#473,.T.);
#8487=EDGE_CURVE('',#6702,#6643,#474,.T.);
#8488=EDGE_CURVE('',#6705,#6699,#1727,.T.);
#8489=EDGE_CURVE('',#6703,#6705,#4524,.T.);
#8490=EDGE_CURVE('',#6705,#6706,#4525,.F.);
#8491=EDGE_CURVE('',#6706,#6707,#4526,.T.);
#8492=EDGE_CURVE('',#6707,#6704,#1120,.T.);
#8493=EDGE_CURVE('',#6708,#6709,#4527,.T.);
#8494=EDGE_CURVE('',#6708,#6710,#4528,.T.);
#8495=EDGE_CURVE('',#6710,#6711,#1121,.T.);
#8496=EDGE_CURVE('',#6711,#6712,#1122,.T.);
#8497=EDGE_CURVE('',#6712,#6709,#4529,.T.);
#8498=EDGE_CURVE('',#6710,#6713,#1728,.T.);
#8499=EDGE_CURVE('',#6714,#6713,#1123,.T.);
#8500=EDGE_CURVE('',#6714,#6646,#475,.T.);
#8501=EDGE_CURVE('',#6711,#6645,#476,.T.);
#8502=EDGE_CURVE('',#6715,#6708,#1729,.T.);
#8503=EDGE_CURVE('',#6713,#6715,#4530,.T.);
#8504=EDGE_CURVE('',#6715,#6716,#4531,.F.);
#8505=EDGE_CURVE('',#6716,#6717,#4532,.T.);
#8506=EDGE_CURVE('',#6717,#6714,#1124,.T.);
#8507=EDGE_CURVE('',#6718,#6719,#4533,.T.);
#8508=EDGE_CURVE('',#6718,#6720,#4534,.T.);
#8509=EDGE_CURVE('',#6720,#6721,#1125,.T.);
#8510=EDGE_CURVE('',#6721,#6722,#1126,.T.);
#8511=EDGE_CURVE('',#6722,#6719,#4535,.T.);
#8512=EDGE_CURVE('',#6720,#6723,#1730,.T.);
#8513=EDGE_CURVE('',#6724,#6723,#1127,.T.);
#8514=EDGE_CURVE('',#6724,#6648,#477,.T.);
#8515=EDGE_CURVE('',#6721,#6647,#478,.T.);
#8516=EDGE_CURVE('',#6725,#6718,#1731,.T.);
#8517=EDGE_CURVE('',#6723,#6725,#4536,.T.);
#8518=EDGE_CURVE('',#6725,#6726,#4537,.F.);
#8519=EDGE_CURVE('',#6726,#6727,#4538,.T.);
#8520=EDGE_CURVE('',#6727,#6724,#1128,.T.);
#8521=EDGE_CURVE('',#6728,#6729,#4539,.T.);
#8522=EDGE_CURVE('',#6728,#6730,#4540,.T.);
#8523=EDGE_CURVE('',#6730,#6731,#1129,.T.);
#8524=EDGE_CURVE('',#6731,#6732,#1130,.T.);
#8525=EDGE_CURVE('',#6732,#6729,#4541,.T.);
#8526=EDGE_CURVE('',#6730,#6733,#1732,.T.);
#8527=EDGE_CURVE('',#6734,#6733,#1131,.T.);
#8528=EDGE_CURVE('',#6734,#6650,#479,.T.);
#8529=EDGE_CURVE('',#6731,#6649,#480,.T.);
#8530=EDGE_CURVE('',#6735,#6728,#1733,.T.);
#8531=EDGE_CURVE('',#6733,#6735,#4542,.T.);
#8532=EDGE_CURVE('',#6735,#6736,#4543,.F.);
#8533=EDGE_CURVE('',#6736,#6737,#4544,.T.);
#8534=EDGE_CURVE('',#6737,#6734,#1132,.T.);
#8535=EDGE_CURVE('',#6738,#6739,#4545,.T.);
#8536=EDGE_CURVE('',#6738,#6740,#4546,.T.);
#8537=EDGE_CURVE('',#6740,#6741,#1133,.T.);
#8538=EDGE_CURVE('',#6741,#6742,#1134,.T.);
#8539=EDGE_CURVE('',#6742,#6739,#4547,.T.);
#8540=EDGE_CURVE('',#6740,#6743,#1734,.T.);
#8541=EDGE_CURVE('',#6744,#6743,#1135,.T.);
#8542=EDGE_CURVE('',#6744,#6652,#481,.T.);
#8543=EDGE_CURVE('',#6741,#6651,#482,.T.);
#8544=EDGE_CURVE('',#6745,#6738,#1735,.T.);
#8545=EDGE_CURVE('',#6743,#6745,#4548,.T.);
#8546=EDGE_CURVE('',#6745,#6746,#4549,.F.);
#8547=EDGE_CURVE('',#6746,#6747,#4550,.T.);
#8548=EDGE_CURVE('',#6747,#6744,#1136,.T.);
#8549=EDGE_CURVE('',#6748,#6749,#4551,.T.);
#8550=EDGE_CURVE('',#6748,#6750,#4552,.T.);
#8551=EDGE_CURVE('',#6750,#6751,#1137,.T.);
#8552=EDGE_CURVE('',#6751,#6752,#1138,.T.);
#8553=EDGE_CURVE('',#6752,#6749,#4553,.T.);
#8554=EDGE_CURVE('',#6750,#6753,#1736,.T.);
#8555=EDGE_CURVE('',#6754,#6753,#1139,.T.);
#8556=EDGE_CURVE('',#6654,#6754,#483,.T.);
#8557=EDGE_CURVE('',#6751,#6653,#484,.T.);
#8558=EDGE_CURVE('',#6755,#6748,#1737,.T.);
#8559=EDGE_CURVE('',#6753,#6755,#4554,.T.);
#8560=EDGE_CURVE('',#6756,#6757,#4555,.T.);
#8561=EDGE_CURVE('',#6758,#6757,#4556,.T.);
#8562=EDGE_CURVE('',#6758,#6759,#4557,.T.);
#8563=EDGE_CURVE('',#6759,#6756,#485,.T.);
#8564=EDGE_CURVE('',#6655,#6756,#486,.T.);
#8565=EDGE_CURVE('',#6759,#6668,#1738,.T.);
#8566=EDGE_CURVE('',#6676,#6678,#1739,.T.);
#8567=EDGE_CURVE('',#6686,#6688,#1740,.T.);
#8568=EDGE_CURVE('',#6689,#6685,#1741,.T.);
#8569=EDGE_CURVE('',#6679,#6675,#1742,.T.);
#8570=EDGE_CURVE('',#6669,#6758,#1743,.T.);
#8571=EDGE_CURVE('',#6755,#6760,#4558,.F.);
#8572=EDGE_CURVE('',#6760,#6754,#4559,.T.);
#8573=EDGE_CURVE('',#6707,#6712,#1744,.T.);
#8574=EDGE_CURVE('',#6717,#6722,#1745,.T.);
#8575=EDGE_CURVE('',#6727,#6732,#1746,.T.);
#8576=EDGE_CURVE('',#6737,#6742,#1747,.T.);
#8577=EDGE_CURVE('',#6747,#6752,#1748,.T.);
#8578=EDGE_CURVE('',#6760,#6757,#1749,.T.);
#8579=EDGE_CURVE('',#6746,#6749,#1750,.T.);
#8580=EDGE_CURVE('',#6736,#6739,#1751,.T.);
#8581=EDGE_CURVE('',#6726,#6729,#1752,.T.);
#8582=EDGE_CURVE('',#6716,#6719,#1753,.T.);
#8583=EDGE_CURVE('',#6706,#6709,#1754,.T.);
#8584=EDGE_CURVE('',#6761,#6762,#1140,.T.);
#8585=EDGE_CURVE('',#6762,#6763,#4560,.T.);
#8586=EDGE_CURVE('',#6763,#6764,#4561,.F.);
#8587=EDGE_CURVE('',#6764,#6765,#4562,.T.);
#8588=EDGE_CURVE('',#6765,#6761,#1141,.T.);
#8589=EDGE_CURVE('',#6765,#6766,#1755,.T.);
#8590=EDGE_CURVE('',#6767,#6766,#1142,.T.);
#8591=EDGE_CURVE('',#6635,#6767,#487,.T.);
#8592=EDGE_CURVE('',#6761,#6634,#488,.T.);
#8593=EDGE_CURVE('',#6764,#6768,#1756,.T.);
#8594=EDGE_CURVE('',#6766,#6768,#4563,.T.);
#8595=EDGE_CURVE('',#6769,#6768,#4564,.T.);
#8596=EDGE_CURVE('',#6769,#6770,#4565,.T.);
#8597=EDGE_CURVE('',#6770,#6767,#1143,.T.);
#8598=EDGE_CURVE('',#6770,#6771,#1757,.T.);
#8599=EDGE_CURVE('',#6772,#6771,#1144,.T.);
#8600=EDGE_CURVE('',#6772,#6636,#489,.T.);
#8601=EDGE_CURVE('',#6771,#6773,#4566,.T.);
#8602=EDGE_CURVE('',#6773,#6774,#4567,.F.);
#8603=EDGE_CURVE('',#6774,#6775,#4568,.T.);
#8604=EDGE_CURVE('',#6775,#6772,#1145,.T.);
#8605=EDGE_CURVE('',#6775,#6776,#1758,.T.);
#8606=EDGE_CURVE('',#6777,#6776,#1146,.T.);
#8607=EDGE_CURVE('',#6777,#6637,#490,.T.);
#8608=EDGE_CURVE('',#6774,#6778,#1759,.T.);
#8609=EDGE_CURVE('',#6776,#6778,#4569,.T.);
#8610=EDGE_CURVE('',#6779,#6778,#4570,.T.);
#8611=EDGE_CURVE('',#6779,#6780,#4571,.T.);
#8612=EDGE_CURVE('',#6780,#6777,#1147,.T.);
#8613=EDGE_CURVE('',#6781,#6782,#1148,.T.);
#8614=EDGE_CURVE('',#6782,#6783,#4572,.T.);
#8615=EDGE_CURVE('',#6783,#6784,#4573,.F.);
#8616=EDGE_CURVE('',#6784,#6785,#4574,.T.);
#8617=EDGE_CURVE('',#6785,#6781,#1149,.T.);
#8618=EDGE_CURVE('',#6785,#6786,#1760,.T.);
#8619=EDGE_CURVE('',#6787,#6786,#1150,.T.);
#8620=EDGE_CURVE('',#6787,#6639,#491,.T.);
#8621=EDGE_CURVE('',#6781,#6638,#492,.T.);
#8622=EDGE_CURVE('',#6784,#6788,#1761,.T.);
#8623=EDGE_CURVE('',#6786,#6788,#4575,.T.);
#8624=EDGE_CURVE('',#6789,#6788,#4576,.T.);
#8625=EDGE_CURVE('',#6789,#6790,#4577,.T.);
#8626=EDGE_CURVE('',#6790,#6787,#1151,.T.);
#8627=EDGE_CURVE('',#6791,#6792,#1152,.T.);
#8628=EDGE_CURVE('',#6792,#6793,#4578,.T.);
#8629=EDGE_CURVE('',#6793,#6794,#4579,.F.);
#8630=EDGE_CURVE('',#6794,#6795,#4580,.T.);
#8631=EDGE_CURVE('',#6795,#6791,#1153,.T.);
#8632=EDGE_CURVE('',#6795,#6796,#1762,.T.);
#8633=EDGE_CURVE('',#6797,#6796,#1154,.T.);
#8634=EDGE_CURVE('',#6797,#6641,#493,.T.);
#8635=EDGE_CURVE('',#6791,#6640,#494,.T.);
#8636=EDGE_CURVE('',#6794,#6798,#1763,.T.);
#8637=EDGE_CURVE('',#6796,#6798,#4581,.T.);
#8638=EDGE_CURVE('',#6799,#6800,#1155,.T.);
#8639=EDGE_CURVE('',#6800,#6801,#4582,.T.);
#8640=EDGE_CURVE('',#6801,#6802,#4583,.F.);
#8641=EDGE_CURVE('',#6802,#6799,#4584,.T.);
#8642=EDGE_CURVE('',#6803,#6800,#1764,.T.);
#8643=EDGE_CURVE('',#6804,#6803,#4585,.T.);
#8644=EDGE_CURVE('',#6801,#6804,#1765,.T.);
#8645=EDGE_CURVE('',#6642,#6799,#495,.T.);
#8646=EDGE_CURVE('',#6803,#6797,#1156,.T.);
#8647=EDGE_CURVE('',#6804,#6798,#4586,.T.);
#8648=EDGE_CURVE('',#6805,#6806,#4587,.T.);
#8649=EDGE_CURVE('',#6805,#6807,#4588,.T.);
#8650=EDGE_CURVE('',#6807,#6808,#1157,.T.);
#8651=EDGE_CURVE('',#6808,#6806,#4589,.T.);
#8652=EDGE_CURVE('',#6807,#6809,#1766,.T.);
#8653=EDGE_CURVE('',#6810,#6809,#1158,.T.);
#8654=EDGE_CURVE('',#6810,#6624,#496,.T.);
#8655=EDGE_CURVE('',#6808,#6623,#497,.T.);
#8656=EDGE_CURVE('',#6811,#6805,#1767,.T.);
#8657=EDGE_CURVE('',#6809,#6811,#4590,.T.);
#8658=EDGE_CURVE('',#6811,#6812,#4591,.F.);
#8659=EDGE_CURVE('',#6812,#6813,#4592,.T.);
#8660=EDGE_CURVE('',#6813,#6810,#1159,.T.);
#8661=EDGE_CURVE('',#6814,#6815,#4593,.T.);
#8662=EDGE_CURVE('',#6814,#6816,#4594,.T.);
#8663=EDGE_CURVE('',#6816,#6817,#1160,.T.);
#8664=EDGE_CURVE('',#6817,#6818,#1161,.T.);
#8665=EDGE_CURVE('',#6818,#6815,#4595,.T.);
#8666=EDGE_CURVE('',#6816,#6819,#1768,.T.);
#8667=EDGE_CURVE('',#6820,#6819,#1162,.T.);
#8668=EDGE_CURVE('',#6820,#6626,#498,.T.);
#8669=EDGE_CURVE('',#6817,#6625,#499,.T.);
#8670=EDGE_CURVE('',#6821,#6814,#1769,.T.);
#8671=EDGE_CURVE('',#6819,#6821,#4596,.T.);
#8672=EDGE_CURVE('',#6821,#6822,#4597,.F.);
#8673=EDGE_CURVE('',#6822,#6823,#4598,.T.);
#8674=EDGE_CURVE('',#6823,#6820,#1163,.T.);
#8675=EDGE_CURVE('',#6824,#6825,#4599,.T.);
#8676=EDGE_CURVE('',#6824,#6826,#4600,.T.);
#8677=EDGE_CURVE('',#6826,#6827,#1164,.T.);
#8678=EDGE_CURVE('',#6827,#6828,#1165,.T.);
#8679=EDGE_CURVE('',#6828,#6825,#4601,.T.);
#8680=EDGE_CURVE('',#6826,#6829,#1770,.T.);
#8681=EDGE_CURVE('',#6830,#6829,#1166,.T.);
#8682=EDGE_CURVE('',#6830,#6628,#500,.T.);
#8683=EDGE_CURVE('',#6827,#6627,#501,.T.);
#8684=EDGE_CURVE('',#6831,#6824,#1771,.T.);
#8685=EDGE_CURVE('',#6829,#6831,#4602,.T.);
#8686=EDGE_CURVE('',#6831,#6832,#4603,.F.);
#8687=EDGE_CURVE('',#6832,#6833,#4604,.T.);
#8688=EDGE_CURVE('',#6833,#6830,#1167,.T.);
#8689=EDGE_CURVE('',#6834,#6835,#4605,.T.);
#8690=EDGE_CURVE('',#6834,#6836,#4606,.T.);
#8691=EDGE_CURVE('',#6836,#6837,#1168,.T.);
#8692=EDGE_CURVE('',#6837,#6838,#1169,.T.);
#8693=EDGE_CURVE('',#6838,#6835,#4607,.T.);
#8694=EDGE_CURVE('',#6836,#6839,#1772,.T.);
#8695=EDGE_CURVE('',#6840,#6839,#1170,.T.);
#8696=EDGE_CURVE('',#6840,#6630,#502,.T.);
#8697=EDGE_CURVE('',#6837,#6629,#503,.T.);
#8698=EDGE_CURVE('',#6841,#6834,#1773,.T.);
#8699=EDGE_CURVE('',#6839,#6841,#4608,.T.);
#8700=EDGE_CURVE('',#6841,#6842,#4609,.F.);
#8701=EDGE_CURVE('',#6842,#6843,#4610,.T.);
#8702=EDGE_CURVE('',#6843,#6840,#1171,.T.);
#8703=EDGE_CURVE('',#6844,#6845,#4611,.T.);
#8704=EDGE_CURVE('',#6844,#6846,#4612,.T.);
#8705=EDGE_CURVE('',#6846,#6847,#1172,.T.);
#8706=EDGE_CURVE('',#6847,#6848,#1173,.T.);
#8707=EDGE_CURVE('',#6848,#6845,#4613,.T.);
#8708=EDGE_CURVE('',#6846,#6849,#1774,.T.);
#8709=EDGE_CURVE('',#6850,#6849,#1174,.T.);
#8710=EDGE_CURVE('',#6632,#6850,#504,.T.);
#8711=EDGE_CURVE('',#6631,#6847,#505,.T.);
#8712=EDGE_CURVE('',#6851,#6844,#1775,.T.);
#8713=EDGE_CURVE('',#6849,#6851,#4614,.T.);
#8714=EDGE_CURVE('',#6852,#6853,#4615,.T.);
#8715=EDGE_CURVE('',#6854,#6853,#4616,.T.);
#8716=EDGE_CURVE('',#6854,#6855,#4617,.T.);
#8717=EDGE_CURVE('',#6855,#6852,#506,.T.);
#8718=EDGE_CURVE('',#6633,#6852,#507,.T.);
#8719=EDGE_CURVE('',#6855,#6762,#1776,.T.);
#8720=EDGE_CURVE('',#6780,#6782,#1777,.T.);
#8721=EDGE_CURVE('',#6790,#6792,#1778,.T.);
#8722=EDGE_CURVE('',#6793,#6789,#1779,.T.);
#8723=EDGE_CURVE('',#6783,#6779,#1780,.T.);
#8724=EDGE_CURVE('',#6773,#6769,#1781,.T.);
#8725=EDGE_CURVE('',#6763,#6854,#1782,.T.);
#8726=EDGE_CURVE('',#6851,#6856,#4618,.F.);
#8727=EDGE_CURVE('',#6856,#6850,#4619,.T.);
#8728=EDGE_CURVE('',#6813,#6818,#1783,.T.);
#8729=EDGE_CURVE('',#6823,#6828,#1784,.T.);
#8730=EDGE_CURVE('',#6833,#6838,#1785,.T.);
#8731=EDGE_CURVE('',#6843,#6848,#1786,.T.);
#8732=EDGE_CURVE('',#6856,#6853,#1787,.T.);
#8733=EDGE_CURVE('',#6842,#6845,#1788,.T.);
#8734=EDGE_CURVE('',#6832,#6835,#1789,.T.);
#8735=EDGE_CURVE('',#6822,#6825,#1790,.T.);
#8736=EDGE_CURVE('',#6812,#6815,#1791,.T.);
#8737=EDGE_CURVE('',#6857,#6858,#1175,.T.);
#8738=EDGE_CURVE('',#6858,#6859,#4620,.T.);
#8739=EDGE_CURVE('',#6859,#6860,#4621,.F.);
#8740=EDGE_CURVE('',#6860,#6861,#4622,.T.);
#8741=EDGE_CURVE('',#6861,#6857,#1176,.T.);
#8742=EDGE_CURVE('',#6861,#6862,#1792,.T.);
#8743=EDGE_CURVE('',#6863,#6862,#1177,.T.);
#8744=EDGE_CURVE('',#6863,#6613,#508,.T.);
#8745=EDGE_CURVE('',#6857,#6612,#509,.T.);
#8746=EDGE_CURVE('',#6860,#6864,#1793,.T.);
#8747=EDGE_CURVE('',#6862,#6864,#4623,.T.);
#8748=EDGE_CURVE('',#6865,#6864,#4624,.T.);
#8749=EDGE_CURVE('',#6865,#6866,#4625,.T.);
#8750=EDGE_CURVE('',#6866,#6863,#1178,.T.);
#8751=EDGE_CURVE('',#6867,#6868,#1179,.T.);
#8752=EDGE_CURVE('',#6868,#6869,#4626,.T.);
#8753=EDGE_CURVE('',#6869,#6870,#4627,.F.);
#8754=EDGE_CURVE('',#6870,#6871,#4628,.T.);
#8755=EDGE_CURVE('',#6871,#6867,#1180,.T.);
#8756=EDGE_CURVE('',#6871,#6872,#1794,.T.);
#8757=EDGE_CURVE('',#6873,#6872,#1181,.T.);
#8758=EDGE_CURVE('',#6873,#6615,#510,.T.);
#8759=EDGE_CURVE('',#6867,#6614,#511,.T.);
#8760=EDGE_CURVE('',#6870,#6874,#1795,.T.);
#8761=EDGE_CURVE('',#6872,#6874,#4629,.T.);
#8762=EDGE_CURVE('',#6875,#6874,#4630,.T.);
#8763=EDGE_CURVE('',#6875,#6876,#4631,.T.);
#8764=EDGE_CURVE('',#6876,#6873,#1182,.T.);
#8765=EDGE_CURVE('',#6877,#6878,#1183,.T.);
#8766=EDGE_CURVE('',#6878,#6879,#4632,.T.);
#8767=EDGE_CURVE('',#6879,#6880,#4633,.F.);
#8768=EDGE_CURVE('',#6880,#6881,#4634,.T.);
#8769=EDGE_CURVE('',#6881,#6877,#1184,.T.);
#8770=EDGE_CURVE('',#6881,#6882,#1796,.T.);
#8771=EDGE_CURVE('',#6883,#6882,#1185,.T.);
#8772=EDGE_CURVE('',#6883,#6617,#512,.T.);
#8773=EDGE_CURVE('',#6877,#6616,#513,.T.);
#8774=EDGE_CURVE('',#6880,#6884,#1797,.T.);
#8775=EDGE_CURVE('',#6882,#6884,#4635,.T.);
#8776=EDGE_CURVE('',#6885,#6884,#4636,.T.);
#8777=EDGE_CURVE('',#6885,#6886,#4637,.T.);
#8778=EDGE_CURVE('',#6886,#6883,#1186,.T.);
#8779=EDGE_CURVE('',#6887,#6888,#1187,.T.);
#8780=EDGE_CURVE('',#6888,#6889,#4638,.T.);
#8781=EDGE_CURVE('',#6889,#6890,#4639,.F.);
#8782=EDGE_CURVE('',#6890,#6891,#4640,.T.);
#8783=EDGE_CURVE('',#6891,#6887,#1188,.T.);
#8784=EDGE_CURVE('',#6891,#6892,#1798,.T.);
#8785=EDGE_CURVE('',#6893,#6892,#1189,.T.);
#8786=EDGE_CURVE('',#6893,#6619,#514,.T.);
#8787=EDGE_CURVE('',#6887,#6618,#515,.T.);
#8788=EDGE_CURVE('',#6890,#6894,#1799,.T.);
#8789=EDGE_CURVE('',#6892,#6894,#4641,.T.);
#8790=EDGE_CURVE('',#6895,#6894,#4642,.T.);
#8791=EDGE_CURVE('',#6895,#6896,#4643,.T.);
#8792=EDGE_CURVE('',#6896,#6893,#1190,.T.);
#8793=EDGE_CURVE('',#6897,#6898,#1191,.T.);
#8794=EDGE_CURVE('',#6898,#6899,#4644,.T.);
#8795=EDGE_CURVE('',#6899,#6900,#4645,.F.);
#8796=EDGE_CURVE('',#6900,#6901,#4646,.T.);
#8797=EDGE_CURVE('',#6901,#6897,#1192,.T.);
#8798=EDGE_CURVE('',#6901,#6902,#1800,.T.);
#8799=EDGE_CURVE('',#6903,#6902,#1193,.T.);
#8800=EDGE_CURVE('',#6903,#6621,#516,.T.);
#8801=EDGE_CURVE('',#6897,#6620,#517,.T.);
#8802=EDGE_CURVE('',#6900,#6904,#1801,.T.);
#8803=EDGE_CURVE('',#6902,#6904,#4647,.T.);
#8804=EDGE_CURVE('',#6905,#6906,#1194,.T.);
#8805=EDGE_CURVE('',#6906,#6907,#4648,.T.);
#8806=EDGE_CURVE('',#6907,#6908,#4649,.F.);
#8807=EDGE_CURVE('',#6908,#6905,#4650,.T.);
#8808=EDGE_CURVE('',#6909,#6906,#1802,.T.);
#8809=EDGE_CURVE('',#6910,#6909,#4651,.T.);
#8810=EDGE_CURVE('',#6907,#6910,#1803,.T.);
#8811=EDGE_CURVE('',#6622,#6905,#518,.T.);
#8812=EDGE_CURVE('',#6909,#6903,#1195,.T.);
#8813=EDGE_CURVE('',#6910,#6904,#4652,.T.);
#8814=EDGE_CURVE('',#6911,#6912,#4653,.T.);
#8815=EDGE_CURVE('',#6911,#6913,#4654,.T.);
#8816=EDGE_CURVE('',#6913,#6914,#1196,.T.);
#8817=EDGE_CURVE('',#6914,#6912,#4655,.T.);
#8818=EDGE_CURVE('',#6913,#6915,#1804,.T.);
#8819=EDGE_CURVE('',#6916,#6915,#1197,.T.);
#8820=EDGE_CURVE('',#6916,#6604,#519,.T.);
#8821=EDGE_CURVE('',#6914,#6603,#520,.T.);
#8822=EDGE_CURVE('',#6917,#6911,#1805,.T.);
#8823=EDGE_CURVE('',#6915,#6917,#4656,.T.);
#8824=EDGE_CURVE('',#6917,#6918,#4657,.F.);
#8825=EDGE_CURVE('',#6918,#6919,#4658,.T.);
#8826=EDGE_CURVE('',#6919,#6916,#1198,.T.);
#8827=EDGE_CURVE('',#6920,#6921,#4659,.T.);
#8828=EDGE_CURVE('',#6920,#6922,#4660,.T.);
#8829=EDGE_CURVE('',#6922,#6923,#1199,.T.);
#8830=EDGE_CURVE('',#6923,#6924,#1200,.T.);
#8831=EDGE_CURVE('',#6924,#6921,#4661,.T.);
#8832=EDGE_CURVE('',#6922,#6925,#1806,.T.);
#8833=EDGE_CURVE('',#6926,#6925,#1201,.T.);
#8834=EDGE_CURVE('',#6926,#6606,#521,.T.);
#8835=EDGE_CURVE('',#6923,#6605,#522,.T.);
#8836=EDGE_CURVE('',#6927,#6920,#1807,.T.);
#8837=EDGE_CURVE('',#6925,#6927,#4662,.T.);
#8838=EDGE_CURVE('',#6927,#6928,#4663,.F.);
#8839=EDGE_CURVE('',#6928,#6929,#4664,.T.);
#8840=EDGE_CURVE('',#6929,#6926,#1202,.T.);
#8841=EDGE_CURVE('',#6930,#6931,#4665,.T.);
#8842=EDGE_CURVE('',#6930,#6932,#4666,.T.);
#8843=EDGE_CURVE('',#6932,#6933,#1203,.T.);
#8844=EDGE_CURVE('',#6933,#6934,#1204,.T.);
#8845=EDGE_CURVE('',#6934,#6931,#4667,.T.);
#8846=EDGE_CURVE('',#6932,#6935,#1808,.T.);
#8847=EDGE_CURVE('',#6936,#6935,#1205,.T.);
#8848=EDGE_CURVE('',#6936,#6608,#523,.T.);
#8849=EDGE_CURVE('',#6933,#6607,#524,.T.);
#8850=EDGE_CURVE('',#6937,#6930,#1809,.T.);
#8851=EDGE_CURVE('',#6935,#6937,#4668,.T.);
#8852=EDGE_CURVE('',#6937,#6938,#4669,.F.);
#8853=EDGE_CURVE('',#6938,#6939,#4670,.T.);
#8854=EDGE_CURVE('',#6939,#6936,#1206,.T.);
#8855=EDGE_CURVE('',#6940,#6941,#4671,.T.);
#8856=EDGE_CURVE('',#6940,#6942,#4672,.T.);
#8857=EDGE_CURVE('',#6942,#6943,#1207,.T.);
#8858=EDGE_CURVE('',#6943,#6944,#1208,.T.);
#8859=EDGE_CURVE('',#6944,#6941,#4673,.T.);
#8860=EDGE_CURVE('',#6942,#6945,#1810,.T.);
#8861=EDGE_CURVE('',#6946,#6945,#1209,.T.);
#8862=EDGE_CURVE('',#6610,#6946,#525,.T.);
#8863=EDGE_CURVE('',#6943,#6609,#526,.T.);
#8864=EDGE_CURVE('',#6947,#6940,#1811,.T.);
#8865=EDGE_CURVE('',#6945,#6947,#4674,.T.);
#8866=EDGE_CURVE('',#6948,#6949,#4675,.T.);
#8867=EDGE_CURVE('',#6950,#6949,#4676,.T.);
#8868=EDGE_CURVE('',#6950,#6951,#4677,.T.);
#8869=EDGE_CURVE('',#6951,#6948,#527,.T.);
#8870=EDGE_CURVE('',#6611,#6948,#528,.T.);
#8871=EDGE_CURVE('',#6951,#6858,#1812,.T.);
#8872=EDGE_CURVE('',#6866,#6868,#1813,.T.);
#8873=EDGE_CURVE('',#6876,#6878,#1814,.T.);
#8874=EDGE_CURVE('',#6886,#6888,#1815,.T.);
#8875=EDGE_CURVE('',#6896,#6898,#1816,.T.);
#8876=EDGE_CURVE('',#6899,#6895,#1817,.T.);
#8877=EDGE_CURVE('',#6889,#6885,#1818,.T.);
#8878=EDGE_CURVE('',#6879,#6875,#1819,.T.);
#8879=EDGE_CURVE('',#6869,#6865,#1820,.T.);
#8880=EDGE_CURVE('',#6859,#6950,#1821,.T.);
#8881=EDGE_CURVE('',#6947,#6952,#4678,.F.);
#8882=EDGE_CURVE('',#6952,#6946,#4679,.T.);
#8883=EDGE_CURVE('',#6919,#6924,#1822,.T.);
#8884=EDGE_CURVE('',#6929,#6934,#1823,.T.);
#8885=EDGE_CURVE('',#6939,#6944,#1824,.T.);
#8886=EDGE_CURVE('',#6952,#6949,#1825,.T.);
#8887=EDGE_CURVE('',#6938,#6941,#1826,.T.);
#8888=EDGE_CURVE('',#6928,#6931,#1827,.T.);
#8889=EDGE_CURVE('',#6918,#6921,#1828,.T.);
#8890=EDGE_CURVE('',#6953,#6954,#1210,.T.);
#8891=EDGE_CURVE('',#6954,#6955,#4680,.T.);
#8892=EDGE_CURVE('',#6955,#6956,#4681,.F.);
#8893=EDGE_CURVE('',#6956,#6957,#4682,.T.);
#8894=EDGE_CURVE('',#6957,#6953,#1211,.T.);
#8895=EDGE_CURVE('',#6957,#6958,#1829,.T.);
#8896=EDGE_CURVE('',#6959,#6958,#1212,.T.);
#8897=EDGE_CURVE('',#6591,#6959,#529,.T.);
#8898=EDGE_CURVE('',#6953,#6590,#530,.T.);
#8899=EDGE_CURVE('',#6956,#6960,#1830,.T.);
#8900=EDGE_CURVE('',#6958,#6960,#4683,.T.);
#8901=EDGE_CURVE('',#6961,#6960,#4684,.T.);
#8902=EDGE_CURVE('',#6961,#6962,#4685,.T.);
#8903=EDGE_CURVE('',#6962,#6959,#1213,.T.);
#8904=EDGE_CURVE('',#6962,#6963,#1831,.T.);
#8905=EDGE_CURVE('',#6964,#6963,#1214,.T.);
#8906=EDGE_CURVE('',#6964,#6592,#531,.T.);
#8907=EDGE_CURVE('',#6963,#6965,#4686,.T.);
#8908=EDGE_CURVE('',#6965,#6966,#4687,.F.);
#8909=EDGE_CURVE('',#6966,#6967,#4688,.T.);
#8910=EDGE_CURVE('',#6967,#6964,#1215,.T.);
#8911=EDGE_CURVE('',#6967,#6968,#1832,.T.);
#8912=EDGE_CURVE('',#6969,#6968,#1216,.T.);
#8913=EDGE_CURVE('',#6969,#6593,#532,.T.);
#8914=EDGE_CURVE('',#6966,#6970,#1833,.T.);
#8915=EDGE_CURVE('',#6968,#6970,#4689,.T.);
#8916=EDGE_CURVE('',#6971,#6970,#4690,.T.);
#8917=EDGE_CURVE('',#6971,#6972,#4691,.T.);
#8918=EDGE_CURVE('',#6972,#6969,#1217,.T.);
#8919=EDGE_CURVE('',#6973,#6974,#1218,.T.);
#8920=EDGE_CURVE('',#6974,#6975,#4692,.T.);
#8921=EDGE_CURVE('',#6975,#6976,#4693,.F.);
#8922=EDGE_CURVE('',#6976,#6977,#4694,.T.);
#8923=EDGE_CURVE('',#6977,#6973,#1219,.T.);
#8924=EDGE_CURVE('',#6977,#6978,#1834,.T.);
#8925=EDGE_CURVE('',#6979,#6978,#1220,.T.);
#8926=EDGE_CURVE('',#6979,#6595,#533,.T.);
#8927=EDGE_CURVE('',#6973,#6594,#534,.T.);
#8928=EDGE_CURVE('',#6976,#6980,#1835,.T.);
#8929=EDGE_CURVE('',#6978,#6980,#4695,.T.);
#8930=EDGE_CURVE('',#6981,#6980,#4696,.T.);
#8931=EDGE_CURVE('',#6981,#6982,#4697,.T.);
#8932=EDGE_CURVE('',#6982,#6979,#1221,.T.);
#8933=EDGE_CURVE('',#6983,#6984,#1222,.T.);
#8934=EDGE_CURVE('',#6984,#6985,#4698,.T.);
#8935=EDGE_CURVE('',#6985,#6986,#4699,.F.);
#8936=EDGE_CURVE('',#6986,#6987,#4700,.T.);
#8937=EDGE_CURVE('',#6987,#6983,#1223,.T.);
#8938=EDGE_CURVE('',#6987,#6988,#1836,.T.);
#8939=EDGE_CURVE('',#6989,#6988,#1224,.T.);
#8940=EDGE_CURVE('',#6989,#6597,#535,.T.);
#8941=EDGE_CURVE('',#6983,#6596,#536,.T.);
#8942=EDGE_CURVE('',#6986,#6990,#1837,.T.);
#8943=EDGE_CURVE('',#6988,#6990,#4701,.T.);
#8944=EDGE_CURVE('',#6991,#6990,#4702,.T.);
#8945=EDGE_CURVE('',#6991,#6992,#4703,.T.);
#8946=EDGE_CURVE('',#6992,#6989,#1225,.T.);
#8947=EDGE_CURVE('',#6993,#6994,#1226,.T.);
#8948=EDGE_CURVE('',#6994,#6995,#4704,.T.);
#8949=EDGE_CURVE('',#6995,#6996,#4705,.F.);
#8950=EDGE_CURVE('',#6996,#6997,#4706,.T.);
#8951=EDGE_CURVE('',#6997,#6993,#1227,.T.);
#8952=EDGE_CURVE('',#6997,#6998,#1838,.T.);
#8953=EDGE_CURVE('',#6999,#6998,#1228,.T.);
#8954=EDGE_CURVE('',#6999,#6599,#537,.T.);
#8955=EDGE_CURVE('',#6993,#6598,#538,.T.);
#8956=EDGE_CURVE('',#6996,#7000,#1839,.T.);
#8957=EDGE_CURVE('',#6998,#7000,#4707,.T.);
#8958=EDGE_CURVE('',#7001,#7000,#4708,.T.);
#8959=EDGE_CURVE('',#7001,#7002,#4709,.T.);
#8960=EDGE_CURVE('',#7002,#6999,#1229,.T.);
#8961=EDGE_CURVE('',#7003,#7004,#1230,.T.);
#8962=EDGE_CURVE('',#7004,#7005,#4710,.T.);
#8963=EDGE_CURVE('',#7005,#7006,#4711,.F.);
#8964=EDGE_CURVE('',#7006,#7007,#4712,.T.);
#8965=EDGE_CURVE('',#7007,#7003,#1231,.T.);
#8966=EDGE_CURVE('',#7007,#7008,#1840,.T.);
#8967=EDGE_CURVE('',#7009,#7008,#1232,.T.);
#8968=EDGE_CURVE('',#7009,#6601,#539,.T.);
#8969=EDGE_CURVE('',#7003,#6600,#540,.T.);
#8970=EDGE_CURVE('',#7006,#7010,#1841,.T.);
#8971=EDGE_CURVE('',#7008,#7010,#4713,.T.);
#8972=EDGE_CURVE('',#7011,#7012,#1233,.T.);
#8973=EDGE_CURVE('',#7012,#7013,#4714,.T.);
#8974=EDGE_CURVE('',#7013,#7014,#4715,.F.);
#8975=EDGE_CURVE('',#7014,#7011,#4716,.T.);
#8976=EDGE_CURVE('',#7015,#7012,#1842,.T.);
#8977=EDGE_CURVE('',#7016,#7015,#4717,.T.);
#8978=EDGE_CURVE('',#7013,#7016,#1843,.T.);
#8979=EDGE_CURVE('',#6602,#7011,#541,.T.);
#8980=EDGE_CURVE('',#7015,#7009,#1234,.T.);
#8981=EDGE_CURVE('',#7016,#7010,#4718,.T.);
#8982=EDGE_CURVE('',#7017,#7018,#4719,.T.);
#8983=EDGE_CURVE('',#7017,#7019,#4720,.T.);
#8984=EDGE_CURVE('',#7019,#7020,#1235,.T.);
#8985=EDGE_CURVE('',#7020,#7018,#4721,.T.);
#8986=EDGE_CURVE('',#7019,#7021,#1844,.T.);
#8987=EDGE_CURVE('',#7022,#7021,#1236,.T.);
#8988=EDGE_CURVE('',#7022,#6584,#542,.T.);
#8989=EDGE_CURVE('',#7020,#6583,#543,.T.);
#8990=EDGE_CURVE('',#7023,#7017,#1845,.T.);
#8991=EDGE_CURVE('',#7021,#7023,#4722,.T.);
#8992=EDGE_CURVE('',#7023,#7024,#4723,.F.);
#8993=EDGE_CURVE('',#7024,#7025,#4724,.T.);
#8994=EDGE_CURVE('',#7025,#7022,#1237,.T.);
#8995=EDGE_CURVE('',#7026,#7027,#4725,.T.);
#8996=EDGE_CURVE('',#7026,#7028,#4726,.T.);
#8997=EDGE_CURVE('',#7028,#7029,#1238,.T.);
#8998=EDGE_CURVE('',#7029,#7030,#1239,.T.);
#8999=EDGE_CURVE('',#7030,#7027,#4727,.T.);
#9000=EDGE_CURVE('',#7028,#7031,#1846,.T.);
#9001=EDGE_CURVE('',#7032,#7031,#1240,.T.);
#9002=EDGE_CURVE('',#7032,#6586,#544,.T.);
#9003=EDGE_CURVE('',#7029,#6585,#545,.T.);
#9004=EDGE_CURVE('',#7033,#7026,#1847,.T.);
#9005=EDGE_CURVE('',#7031,#7033,#4728,.T.);
#9006=EDGE_CURVE('',#7033,#7034,#4729,.F.);
#9007=EDGE_CURVE('',#7034,#7035,#4730,.T.);
#9008=EDGE_CURVE('',#7035,#7032,#1241,.T.);
#9009=EDGE_CURVE('',#7036,#7037,#4731,.T.);
#9010=EDGE_CURVE('',#7036,#7038,#4732,.T.);
#9011=EDGE_CURVE('',#7038,#7039,#1242,.T.);
#9012=EDGE_CURVE('',#7039,#7040,#1243,.T.);
#9013=EDGE_CURVE('',#7040,#7037,#4733,.T.);
#9014=EDGE_CURVE('',#7038,#7041,#1848,.T.);
#9015=EDGE_CURVE('',#7042,#7041,#1244,.T.);
#9016=EDGE_CURVE('',#6588,#7042,#546,.T.);
#9017=EDGE_CURVE('',#6587,#7039,#547,.T.);
#9018=EDGE_CURVE('',#7043,#7036,#1849,.T.);
#9019=EDGE_CURVE('',#7041,#7043,#4734,.T.);
#9020=EDGE_CURVE('',#7044,#7045,#4735,.T.);
#9021=EDGE_CURVE('',#7046,#7045,#4736,.T.);
#9022=EDGE_CURVE('',#7046,#7047,#4737,.T.);
#9023=EDGE_CURVE('',#7047,#7044,#548,.T.);
#9024=EDGE_CURVE('',#6589,#7044,#549,.T.);
#9025=EDGE_CURVE('',#7047,#6954,#1850,.T.);
#9026=EDGE_CURVE('',#6972,#6974,#1851,.T.);
#9027=EDGE_CURVE('',#6982,#6984,#1852,.T.);
#9028=EDGE_CURVE('',#6992,#6994,#1853,.T.);
#9029=EDGE_CURVE('',#7002,#7004,#1854,.T.);
#9030=EDGE_CURVE('',#7005,#7001,#1855,.T.);
#9031=EDGE_CURVE('',#6995,#6991,#1856,.T.);
#9032=EDGE_CURVE('',#6985,#6981,#1857,.T.);
#9033=EDGE_CURVE('',#6975,#6971,#1858,.T.);
#9034=EDGE_CURVE('',#6965,#6961,#1859,.T.);
#9035=EDGE_CURVE('',#6955,#7046,#1860,.T.);
#9036=EDGE_CURVE('',#7043,#7048,#4738,.F.);
#9037=EDGE_CURVE('',#7048,#7042,#4739,.T.);
#9038=EDGE_CURVE('',#7025,#7030,#1861,.T.);
#9039=EDGE_CURVE('',#7035,#7040,#1862,.T.);
#9040=EDGE_CURVE('',#7048,#7045,#1863,.T.);
#9041=EDGE_CURVE('',#7034,#7037,#1864,.T.);
#9042=EDGE_CURVE('',#7024,#7027,#1865,.T.);
#9043=EDGE_CURVE('',#7049,#7050,#1245,.T.);
#9044=EDGE_CURVE('',#7050,#7051,#4740,.T.);
#9045=EDGE_CURVE('',#7051,#7052,#4741,.F.);
#9046=EDGE_CURVE('',#7052,#7053,#4742,.T.);
#9047=EDGE_CURVE('',#7053,#7049,#1246,.T.);
#9048=EDGE_CURVE('',#7053,#7054,#1866,.T.);
#9049=EDGE_CURVE('',#7055,#7054,#1247,.T.);
#9050=EDGE_CURVE('',#7055,#6569,#550,.T.);
#9051=EDGE_CURVE('',#7049,#6568,#551,.T.);
#9052=EDGE_CURVE('',#7052,#7056,#1867,.T.);
#9053=EDGE_CURVE('',#7054,#7056,#4743,.T.);
#9054=EDGE_CURVE('',#7057,#7056,#4744,.T.);
#9055=EDGE_CURVE('',#7057,#7058,#4745,.T.);
#9056=EDGE_CURVE('',#7058,#7055,#1248,.T.);
#9057=EDGE_CURVE('',#7059,#7060,#1249,.T.);
#9058=EDGE_CURVE('',#7060,#7061,#4746,.T.);
#9059=EDGE_CURVE('',#7061,#7062,#4747,.F.);
#9060=EDGE_CURVE('',#7062,#7063,#4748,.T.);
#9061=EDGE_CURVE('',#7063,#7059,#1250,.T.);
#9062=EDGE_CURVE('',#7063,#7064,#1868,.T.);
#9063=EDGE_CURVE('',#7065,#7064,#1251,.T.);
#9064=EDGE_CURVE('',#7065,#6571,#552,.T.);
#9065=EDGE_CURVE('',#7059,#6570,#553,.T.);
#9066=EDGE_CURVE('',#7062,#7066,#1869,.T.);
#9067=EDGE_CURVE('',#7064,#7066,#4749,.T.);
#9068=EDGE_CURVE('',#7067,#7066,#4750,.T.);
#9069=EDGE_CURVE('',#7067,#7068,#4751,.T.);
#9070=EDGE_CURVE('',#7068,#7065,#1252,.T.);
#9071=EDGE_CURVE('',#7069,#7070,#1253,.T.);
#9072=EDGE_CURVE('',#7070,#7071,#4752,.T.);
#9073=EDGE_CURVE('',#7071,#7072,#4753,.F.);
#9074=EDGE_CURVE('',#7072,#7073,#4754,.T.);
#9075=EDGE_CURVE('',#7073,#7069,#1254,.T.);
#9076=EDGE_CURVE('',#7073,#7074,#1870,.T.);
#9077=EDGE_CURVE('',#7075,#7074,#1255,.T.);
#9078=EDGE_CURVE('',#7075,#6573,#554,.T.);
#9079=EDGE_CURVE('',#7069,#6572,#555,.T.);
#9080=EDGE_CURVE('',#7072,#7076,#1871,.T.);
#9081=EDGE_CURVE('',#7074,#7076,#4755,.T.);
#9082=EDGE_CURVE('',#7077,#7076,#4756,.T.);
#9083=EDGE_CURVE('',#7077,#7078,#4757,.T.);
#9084=EDGE_CURVE('',#7078,#7075,#1256,.T.);
#9085=EDGE_CURVE('',#7079,#7080,#1257,.T.);
#9086=EDGE_CURVE('',#7080,#7081,#4758,.T.);
#9087=EDGE_CURVE('',#7081,#7082,#4759,.F.);
#9088=EDGE_CURVE('',#7082,#7083,#4760,.T.);
#9089=EDGE_CURVE('',#7083,#7079,#1258,.T.);
#9090=EDGE_CURVE('',#7083,#7084,#1872,.T.);
#9091=EDGE_CURVE('',#7085,#7084,#1259,.T.);
#9092=EDGE_CURVE('',#7085,#6575,#556,.T.);
#9093=EDGE_CURVE('',#7079,#6574,#557,.T.);
#9094=EDGE_CURVE('',#7082,#7086,#1873,.T.);
#9095=EDGE_CURVE('',#7084,#7086,#4761,.T.);
#9096=EDGE_CURVE('',#7087,#7086,#4762,.T.);
#9097=EDGE_CURVE('',#7087,#7088,#4763,.T.);
#9098=EDGE_CURVE('',#7088,#7085,#1260,.T.);
#9099=EDGE_CURVE('',#7089,#7090,#1261,.T.);
#9100=EDGE_CURVE('',#7090,#7091,#4764,.T.);
#9101=EDGE_CURVE('',#7091,#7092,#4765,.F.);
#9102=EDGE_CURVE('',#7092,#7093,#4766,.T.);
#9103=EDGE_CURVE('',#7093,#7089,#1262,.T.);
#9104=EDGE_CURVE('',#7093,#7094,#1874,.T.);
#9105=EDGE_CURVE('',#7095,#7094,#1263,.T.);
#9106=EDGE_CURVE('',#7095,#6577,#558,.T.);
#9107=EDGE_CURVE('',#7089,#6576,#559,.T.);
#9108=EDGE_CURVE('',#7092,#7096,#1875,.T.);
#9109=EDGE_CURVE('',#7094,#7096,#4767,.T.);
#9110=EDGE_CURVE('',#7097,#7096,#4768,.T.);
#9111=EDGE_CURVE('',#7097,#7098,#4769,.T.);
#9112=EDGE_CURVE('',#7098,#7095,#1264,.T.);
#9113=EDGE_CURVE('',#7099,#7100,#1265,.T.);
#9114=EDGE_CURVE('',#7100,#7101,#4770,.T.);
#9115=EDGE_CURVE('',#7101,#7102,#4771,.F.);
#9116=EDGE_CURVE('',#7102,#7103,#4772,.T.);
#9117=EDGE_CURVE('',#7103,#7099,#1266,.T.);
#9118=EDGE_CURVE('',#7103,#7104,#1876,.T.);
#9119=EDGE_CURVE('',#7105,#7104,#1267,.T.);
#9120=EDGE_CURVE('',#7105,#6579,#560,.T.);
#9121=EDGE_CURVE('',#7099,#6578,#561,.T.);
#9122=EDGE_CURVE('',#7102,#7106,#1877,.T.);
#9123=EDGE_CURVE('',#7104,#7106,#4773,.T.);
#9124=EDGE_CURVE('',#7107,#7106,#4774,.T.);
#9125=EDGE_CURVE('',#7107,#7108,#4775,.T.);
#9126=EDGE_CURVE('',#7108,#7105,#1268,.T.);
#9127=EDGE_CURVE('',#7109,#7110,#1269,.T.);
#9128=EDGE_CURVE('',#7110,#7111,#4776,.T.);
#9129=EDGE_CURVE('',#7111,#7112,#4777,.F.);
#9130=EDGE_CURVE('',#7112,#7113,#4778,.T.);
#9131=EDGE_CURVE('',#7113,#7109,#1270,.T.);
#9132=EDGE_CURVE('',#7113,#7114,#1878,.T.);
#9133=EDGE_CURVE('',#7115,#7114,#1271,.T.);
#9134=EDGE_CURVE('',#7115,#6581,#562,.T.);
#9135=EDGE_CURVE('',#7109,#6580,#563,.T.);
#9136=EDGE_CURVE('',#7112,#7116,#1879,.T.);
#9137=EDGE_CURVE('',#7114,#7116,#4779,.T.);
#9138=EDGE_CURVE('',#7117,#7118,#1272,.T.);
#9139=EDGE_CURVE('',#7118,#7119,#4780,.T.);
#9140=EDGE_CURVE('',#7119,#7120,#4781,.F.);
#9141=EDGE_CURVE('',#7120,#7117,#4782,.T.);
#9142=EDGE_CURVE('',#7121,#7118,#1880,.T.);
#9143=EDGE_CURVE('',#7122,#7121,#4783,.T.);
#9144=EDGE_CURVE('',#7119,#7122,#1881,.T.);
#9145=EDGE_CURVE('',#6582,#7117,#564,.T.);
#9146=EDGE_CURVE('',#7121,#7115,#1273,.T.);
#9147=EDGE_CURVE('',#7122,#7116,#4784,.T.);
#9148=EDGE_CURVE('',#7123,#7124,#4785,.T.);
#9149=EDGE_CURVE('',#7123,#7125,#4786,.T.);
#9150=EDGE_CURVE('',#7125,#7126,#1274,.T.);
#9151=EDGE_CURVE('',#7126,#7124,#4787,.T.);
#9152=EDGE_CURVE('',#7125,#7127,#1882,.T.);
#9153=EDGE_CURVE('',#7128,#7127,#1275,.T.);
#9154=EDGE_CURVE('',#7128,#6564,#565,.T.);
#9155=EDGE_CURVE('',#7126,#6563,#566,.T.);
#9156=EDGE_CURVE('',#7129,#7123,#1883,.T.);
#9157=EDGE_CURVE('',#7127,#7129,#4788,.T.);
#9158=EDGE_CURVE('',#7129,#7130,#4789,.F.);
#9159=EDGE_CURVE('',#7130,#7131,#4790,.T.);
#9160=EDGE_CURVE('',#7131,#7128,#1276,.T.);
#9161=EDGE_CURVE('',#7132,#7133,#4791,.T.);
#9162=EDGE_CURVE('',#7132,#7134,#4792,.T.);
#9163=EDGE_CURVE('',#7134,#7135,#1277,.T.);
#9164=EDGE_CURVE('',#7135,#7136,#1278,.T.);
#9165=EDGE_CURVE('',#7136,#7133,#4793,.T.);
#9166=EDGE_CURVE('',#7134,#7137,#1884,.T.);
#9167=EDGE_CURVE('',#7138,#7137,#1279,.T.);
#9168=EDGE_CURVE('',#6566,#7138,#567,.T.);
#9169=EDGE_CURVE('',#7135,#6565,#568,.T.);
#9170=EDGE_CURVE('',#7139,#7132,#1885,.T.);
#9171=EDGE_CURVE('',#7137,#7139,#4794,.T.);
#9172=EDGE_CURVE('',#7140,#7141,#4795,.T.);
#9173=EDGE_CURVE('',#7142,#7141,#4796,.T.);
#9174=EDGE_CURVE('',#7142,#7143,#4797,.T.);
#9175=EDGE_CURVE('',#7143,#7140,#569,.T.);
#9176=EDGE_CURVE('',#6567,#7140,#570,.T.);
#9177=EDGE_CURVE('',#7143,#7050,#1886,.T.);
#9178=EDGE_CURVE('',#7058,#7060,#1887,.T.);
#9179=EDGE_CURVE('',#7068,#7070,#1888,.T.);
#9180=EDGE_CURVE('',#7078,#7080,#1889,.T.);
#9181=EDGE_CURVE('',#7088,#7090,#1890,.T.);
#9182=EDGE_CURVE('',#7098,#7100,#1891,.T.);
#9183=EDGE_CURVE('',#7108,#7110,#1892,.T.);
#9184=EDGE_CURVE('',#7111,#7107,#1893,.T.);
#9185=EDGE_CURVE('',#7101,#7097,#1894,.T.);
#9186=EDGE_CURVE('',#7091,#7087,#1895,.T.);
#9187=EDGE_CURVE('',#7081,#7077,#1896,.T.);
#9188=EDGE_CURVE('',#7071,#7067,#1897,.T.);
#9189=EDGE_CURVE('',#7061,#7057,#1898,.T.);
#9190=EDGE_CURVE('',#7051,#7142,#1899,.T.);
#9191=EDGE_CURVE('',#7139,#7144,#4798,.F.);
#9192=EDGE_CURVE('',#7144,#7138,#4799,.T.);
#9193=EDGE_CURVE('',#7131,#7136,#1900,.T.);
#9194=EDGE_CURVE('',#7144,#7141,#1901,.T.);
#9195=EDGE_CURVE('',#7130,#7133,#1902,.T.);
#9196=EDGE_CURVE('',#7145,#7146,#1280,.T.);
#9197=EDGE_CURVE('',#7146,#7147,#4800,.T.);
#9198=EDGE_CURVE('',#7147,#7148,#4801,.F.);
#9199=EDGE_CURVE('',#7148,#7149,#4802,.T.);
#9200=EDGE_CURVE('',#7149,#7145,#1281,.T.);
#9201=EDGE_CURVE('',#7149,#7150,#1903,.T.);
#9202=EDGE_CURVE('',#7151,#7150,#1282,.T.);
#9203=EDGE_CURVE('',#7151,#6547,#571,.T.);
#9204=EDGE_CURVE('',#7145,#6546,#572,.T.);
#9205=EDGE_CURVE('',#7148,#7152,#1904,.T.);
#9206=EDGE_CURVE('',#7150,#7152,#4803,.T.);
#9207=EDGE_CURVE('',#7153,#7152,#4804,.T.);
#9208=EDGE_CURVE('',#7153,#7154,#4805,.T.);
#9209=EDGE_CURVE('',#7154,#7151,#1283,.T.);
#9210=EDGE_CURVE('',#7155,#7156,#1284,.T.);
#9211=EDGE_CURVE('',#7156,#7157,#4806,.T.);
#9212=EDGE_CURVE('',#7157,#7158,#4807,.F.);
#9213=EDGE_CURVE('',#7158,#7159,#4808,.T.);
#9214=EDGE_CURVE('',#7159,#7155,#1285,.T.);
#9215=EDGE_CURVE('',#7159,#7160,#1905,.T.);
#9216=EDGE_CURVE('',#7161,#7160,#1286,.T.);
#9217=EDGE_CURVE('',#7161,#6549,#573,.T.);
#9218=EDGE_CURVE('',#7155,#6548,#574,.T.);
#9219=EDGE_CURVE('',#7158,#7162,#1906,.T.);
#9220=EDGE_CURVE('',#7160,#7162,#4809,.T.);
#9221=EDGE_CURVE('',#7163,#7162,#4810,.T.);
#9222=EDGE_CURVE('',#7163,#7164,#4811,.T.);
#9223=EDGE_CURVE('',#7164,#7161,#1287,.T.);
#9224=EDGE_CURVE('',#7165,#7166,#1288,.T.);
#9225=EDGE_CURVE('',#7166,#7167,#4812,.T.);
#9226=EDGE_CURVE('',#7167,#7168,#4813,.F.);
#9227=EDGE_CURVE('',#7168,#7169,#4814,.T.);
#9228=EDGE_CURVE('',#7169,#7165,#1289,.T.);
#9229=EDGE_CURVE('',#7169,#7170,#1907,.T.);
#9230=EDGE_CURVE('',#7171,#7170,#1290,.T.);
#9231=EDGE_CURVE('',#7171,#6551,#575,.T.);
#9232=EDGE_CURVE('',#7165,#6550,#576,.T.);
#9233=EDGE_CURVE('',#7168,#7172,#1908,.T.);
#9234=EDGE_CURVE('',#7170,#7172,#4815,.T.);
#9235=EDGE_CURVE('',#7173,#7172,#4816,.T.);
#9236=EDGE_CURVE('',#7173,#7174,#4817,.T.);
#9237=EDGE_CURVE('',#7174,#7171,#1291,.T.);
#9238=EDGE_CURVE('',#7175,#7176,#1292,.T.);
#9239=EDGE_CURVE('',#7176,#7177,#4818,.T.);
#9240=EDGE_CURVE('',#7177,#7178,#4819,.F.);
#9241=EDGE_CURVE('',#7178,#7179,#4820,.T.);
#9242=EDGE_CURVE('',#7179,#7175,#1293,.T.);
#9243=EDGE_CURVE('',#7179,#7180,#1909,.T.);
#9244=EDGE_CURVE('',#7181,#7180,#1294,.T.);
#9245=EDGE_CURVE('',#7181,#6553,#577,.T.);
#9246=EDGE_CURVE('',#7175,#6552,#578,.T.);
#9247=EDGE_CURVE('',#7178,#7182,#1910,.T.);
#9248=EDGE_CURVE('',#7180,#7182,#4821,.T.);
#9249=EDGE_CURVE('',#7183,#7182,#4822,.T.);
#9250=EDGE_CURVE('',#7183,#7184,#4823,.T.);
#9251=EDGE_CURVE('',#7184,#7181,#1295,.T.);
#9252=EDGE_CURVE('',#7185,#7186,#1296,.T.);
#9253=EDGE_CURVE('',#7186,#7187,#4824,.T.);
#9254=EDGE_CURVE('',#7187,#7188,#4825,.F.);
#9255=EDGE_CURVE('',#7188,#7189,#4826,.T.);
#9256=EDGE_CURVE('',#7189,#7185,#1297,.T.);
#9257=EDGE_CURVE('',#7189,#7190,#1911,.T.);
#9258=EDGE_CURVE('',#7191,#7190,#1298,.T.);
#9259=EDGE_CURVE('',#7191,#6555,#579,.T.);
#9260=EDGE_CURVE('',#7185,#6554,#580,.T.);
#9261=EDGE_CURVE('',#7188,#7192,#1912,.T.);
#9262=EDGE_CURVE('',#7190,#7192,#4827,.T.);
#9263=EDGE_CURVE('',#7193,#7192,#4828,.T.);
#9264=EDGE_CURVE('',#7193,#7194,#4829,.T.);
#9265=EDGE_CURVE('',#7194,#7191,#1299,.T.);
#9266=EDGE_CURVE('',#7195,#7196,#1300,.T.);
#9267=EDGE_CURVE('',#7196,#7197,#4830,.T.);
#9268=EDGE_CURVE('',#7197,#7198,#4831,.F.);
#9269=EDGE_CURVE('',#7198,#7199,#4832,.T.);
#9270=EDGE_CURVE('',#7199,#7195,#1301,.T.);
#9271=EDGE_CURVE('',#7199,#7200,#1913,.T.);
#9272=EDGE_CURVE('',#7201,#7200,#1302,.T.);
#9273=EDGE_CURVE('',#7201,#6557,#581,.T.);
#9274=EDGE_CURVE('',#7195,#6556,#582,.T.);
#9275=EDGE_CURVE('',#7198,#7202,#1914,.T.);
#9276=EDGE_CURVE('',#7200,#7202,#4833,.T.);
#9277=EDGE_CURVE('',#7203,#7202,#4834,.T.);
#9278=EDGE_CURVE('',#7203,#7204,#4835,.T.);
#9279=EDGE_CURVE('',#7204,#7201,#1303,.T.);
#9280=EDGE_CURVE('',#7205,#7206,#1304,.T.);
#9281=EDGE_CURVE('',#7206,#7207,#4836,.T.);
#9282=EDGE_CURVE('',#7207,#7208,#4837,.F.);
#9283=EDGE_CURVE('',#7208,#7209,#4838,.T.);
#9284=EDGE_CURVE('',#7209,#7205,#1305,.T.);
#9285=EDGE_CURVE('',#7209,#7210,#1915,.T.);
#9286=EDGE_CURVE('',#7211,#7210,#1306,.T.);
#9287=EDGE_CURVE('',#7211,#6559,#583,.T.);
#9288=EDGE_CURVE('',#7205,#6558,#584,.T.);
#9289=EDGE_CURVE('',#7208,#7212,#1916,.T.);
#9290=EDGE_CURVE('',#7210,#7212,#4839,.T.);
#9291=EDGE_CURVE('',#7213,#7212,#4840,.T.);
#9292=EDGE_CURVE('',#7213,#7214,#4841,.T.);
#9293=EDGE_CURVE('',#7214,#7211,#1307,.T.);
#9294=EDGE_CURVE('',#7215,#7216,#1308,.T.);
#9295=EDGE_CURVE('',#7216,#7217,#4842,.T.);
#9296=EDGE_CURVE('',#7217,#7218,#4843,.F.);
#9297=EDGE_CURVE('',#7218,#7219,#4844,.T.);
#9298=EDGE_CURVE('',#7219,#7215,#1309,.T.);
#9299=EDGE_CURVE('',#7219,#7220,#1917,.T.);
#9300=EDGE_CURVE('',#7221,#7220,#1310,.T.);
#9301=EDGE_CURVE('',#7221,#6561,#585,.T.);
#9302=EDGE_CURVE('',#7215,#6560,#586,.T.);
#9303=EDGE_CURVE('',#7218,#7222,#1918,.T.);
#9304=EDGE_CURVE('',#7220,#7222,#4845,.T.);
#9305=EDGE_CURVE('',#7223,#7224,#1311,.T.);
#9306=EDGE_CURVE('',#7224,#7225,#4846,.T.);
#9307=EDGE_CURVE('',#7225,#7226,#4847,.F.);
#9308=EDGE_CURVE('',#7226,#7223,#4848,.T.);
#9309=EDGE_CURVE('',#7227,#7224,#1919,.T.);
#9310=EDGE_CURVE('',#7228,#7227,#4849,.T.);
#9311=EDGE_CURVE('',#7225,#7228,#1920,.T.);
#9312=EDGE_CURVE('',#6562,#7223,#587,.T.);
#9313=EDGE_CURVE('',#7227,#7221,#1312,.T.);
#9314=EDGE_CURVE('',#7228,#7222,#4850,.T.);
#9315=EDGE_CURVE('',#7229,#7230,#4851,.T.);
#9316=EDGE_CURVE('',#7229,#7231,#4852,.T.);
#9317=EDGE_CURVE('',#7231,#7232,#1313,.T.);
#9318=EDGE_CURVE('',#7232,#7230,#4853,.T.);
#9319=EDGE_CURVE('',#7231,#7233,#1921,.T.);
#9320=EDGE_CURVE('',#7234,#7233,#1314,.T.);
#9321=EDGE_CURVE('',#6544,#7234,#588,.T.);
#9322=EDGE_CURVE('',#7232,#6543,#589,.T.);
#9323=EDGE_CURVE('',#7235,#7229,#1922,.T.);
#9324=EDGE_CURVE('',#7233,#7235,#4854,.T.);
#9325=EDGE_CURVE('',#7236,#7237,#4855,.T.);
#9326=EDGE_CURVE('',#7238,#7237,#4856,.T.);
#9327=EDGE_CURVE('',#7238,#7239,#4857,.T.);
#9328=EDGE_CURVE('',#7239,#7236,#590,.T.);
#9329=EDGE_CURVE('',#6545,#7236,#591,.T.);
#9330=EDGE_CURVE('',#7239,#7146,#1923,.T.);
#9331=EDGE_CURVE('',#7154,#7156,#1924,.T.);
#9332=EDGE_CURVE('',#7164,#7166,#1925,.T.);
#9333=EDGE_CURVE('',#7174,#7176,#1926,.T.);
#9334=EDGE_CURVE('',#7184,#7186,#1927,.T.);
#9335=EDGE_CURVE('',#7194,#7196,#1928,.T.);
#9336=EDGE_CURVE('',#7204,#7206,#1929,.T.);
#9337=EDGE_CURVE('',#7214,#7216,#1930,.T.);
#9338=EDGE_CURVE('',#7217,#7213,#1931,.T.);
#9339=EDGE_CURVE('',#7207,#7203,#1932,.T.);
#9340=EDGE_CURVE('',#7197,#7193,#1933,.T.);
#9341=EDGE_CURVE('',#7187,#7183,#1934,.T.);
#9342=EDGE_CURVE('',#7177,#7173,#1935,.T.);
#9343=EDGE_CURVE('',#7167,#7163,#1936,.T.);
#9344=EDGE_CURVE('',#7157,#7153,#1937,.T.);
#9345=EDGE_CURVE('',#7147,#7238,#1938,.T.);
#9346=EDGE_CURVE('',#7235,#7240,#4858,.F.);
#9347=EDGE_CURVE('',#7240,#7234,#4859,.T.);
#9348=EDGE_CURVE('',#7240,#7237,#1939,.T.);
#9349=EDGE_CURVE('',#7241,#7242,#4860,.T.);
#9350=EDGE_CURVE('',#7241,#7243,#4861,.T.);
#9351=EDGE_CURVE('',#7243,#6510,#1315,.T.);
#9352=EDGE_CURVE('',#6509,#7242,#4862,.T.);
#9353=EDGE_CURVE('',#7243,#7244,#1940,.T.);
#9354=EDGE_CURVE('',#7245,#7244,#1316,.T.);
#9355=EDGE_CURVE('',#7245,#6526,#592,.T.);
#9356=EDGE_CURVE('',#7246,#7241,#1941,.T.);
#9357=EDGE_CURVE('',#7244,#7246,#4863,.T.);
#9358=EDGE_CURVE('',#7246,#7247,#4864,.F.);
#9359=EDGE_CURVE('',#7247,#7248,#4865,.T.);
#9360=EDGE_CURVE('',#7248,#7245,#1317,.T.);
#9361=EDGE_CURVE('',#7249,#7250,#4866,.T.);
#9362=EDGE_CURVE('',#7249,#7251,#4867,.T.);
#9363=EDGE_CURVE('',#7251,#7252,#1318,.T.);
#9364=EDGE_CURVE('',#7252,#7253,#1319,.T.);
#9365=EDGE_CURVE('',#7253,#7250,#4868,.T.);
#9366=EDGE_CURVE('',#7251,#7254,#1942,.T.);
#9367=EDGE_CURVE('',#7255,#7254,#1320,.T.);
#9368=EDGE_CURVE('',#7255,#6528,#593,.T.);
#9369=EDGE_CURVE('',#7252,#6527,#594,.T.);
#9370=EDGE_CURVE('',#7256,#7249,#1943,.T.);
#9371=EDGE_CURVE('',#7254,#7256,#4869,.T.);
#9372=EDGE_CURVE('',#7256,#7257,#4870,.F.);
#9373=EDGE_CURVE('',#7257,#7258,#4871,.T.);
#9374=EDGE_CURVE('',#7258,#7255,#1321,.T.);
#9375=EDGE_CURVE('',#7259,#7260,#4872,.T.);
#9376=EDGE_CURVE('',#7259,#7261,#4873,.T.);
#9377=EDGE_CURVE('',#7261,#7262,#1322,.T.);
#9378=EDGE_CURVE('',#7262,#7263,#1323,.T.);
#9379=EDGE_CURVE('',#7263,#7260,#4874,.T.);
#9380=EDGE_CURVE('',#7261,#7264,#1944,.T.);
#9381=EDGE_CURVE('',#7265,#7264,#1324,.T.);
#9382=EDGE_CURVE('',#7265,#6530,#595,.T.);
#9383=EDGE_CURVE('',#7262,#6529,#596,.T.);
#9384=EDGE_CURVE('',#7266,#7259,#1945,.T.);
#9385=EDGE_CURVE('',#7264,#7266,#4875,.T.);
#9386=EDGE_CURVE('',#7266,#7267,#4876,.F.);
#9387=EDGE_CURVE('',#7267,#7268,#4877,.T.);
#9388=EDGE_CURVE('',#7268,#7265,#1325,.T.);
#9389=EDGE_CURVE('',#7269,#7270,#4878,.T.);
#9390=EDGE_CURVE('',#7269,#7271,#4879,.T.);
#9391=EDGE_CURVE('',#7271,#7272,#1326,.T.);
#9392=EDGE_CURVE('',#7272,#7273,#1327,.T.);
#9393=EDGE_CURVE('',#7273,#7270,#4880,.T.);
#9394=EDGE_CURVE('',#7271,#7274,#1946,.T.);
#9395=EDGE_CURVE('',#7275,#7274,#1328,.T.);
#9396=EDGE_CURVE('',#7275,#6532,#597,.T.);
#9397=EDGE_CURVE('',#7272,#6531,#598,.T.);
#9398=EDGE_CURVE('',#7276,#7269,#1947,.T.);
#9399=EDGE_CURVE('',#7274,#7276,#4881,.T.);
#9400=EDGE_CURVE('',#7276,#7277,#4882,.F.);
#9401=EDGE_CURVE('',#7277,#7278,#4883,.T.);
#9402=EDGE_CURVE('',#7278,#7275,#1329,.T.);
#9403=EDGE_CURVE('',#7279,#7280,#4884,.T.);
#9404=EDGE_CURVE('',#7279,#7281,#4885,.T.);
#9405=EDGE_CURVE('',#7281,#7282,#1330,.T.);
#9406=EDGE_CURVE('',#7282,#7283,#1331,.T.);
#9407=EDGE_CURVE('',#7283,#7280,#4886,.T.);
#9408=EDGE_CURVE('',#7281,#7284,#1948,.T.);
#9409=EDGE_CURVE('',#7285,#7284,#1332,.T.);
#9410=EDGE_CURVE('',#7285,#6534,#599,.T.);
#9411=EDGE_CURVE('',#7282,#6533,#600,.T.);
#9412=EDGE_CURVE('',#7286,#7279,#1949,.T.);
#9413=EDGE_CURVE('',#7284,#7286,#4887,.T.);
#9414=EDGE_CURVE('',#7286,#7287,#4888,.F.);
#9415=EDGE_CURVE('',#7287,#7288,#4889,.T.);
#9416=EDGE_CURVE('',#7288,#7285,#1333,.T.);
#9417=EDGE_CURVE('',#7289,#7290,#4890,.T.);
#9418=EDGE_CURVE('',#7289,#7291,#4891,.T.);
#9419=EDGE_CURVE('',#7291,#7292,#1334,.T.);
#9420=EDGE_CURVE('',#7292,#7293,#1335,.T.);
#9421=EDGE_CURVE('',#7293,#7290,#4892,.T.);
#9422=EDGE_CURVE('',#7291,#7294,#1950,.T.);
#9423=EDGE_CURVE('',#7295,#7294,#1336,.T.);
#9424=EDGE_CURVE('',#7295,#6536,#601,.T.);
#9425=EDGE_CURVE('',#7292,#6535,#602,.T.);
#9426=EDGE_CURVE('',#7296,#7289,#1951,.T.);
#9427=EDGE_CURVE('',#7294,#7296,#4893,.T.);
#9428=EDGE_CURVE('',#7296,#7297,#4894,.F.);
#9429=EDGE_CURVE('',#7297,#7298,#4895,.T.);
#9430=EDGE_CURVE('',#7298,#7295,#1337,.T.);
#9431=EDGE_CURVE('',#7299,#7300,#4896,.T.);
#9432=EDGE_CURVE('',#7299,#7301,#4897,.T.);
#9433=EDGE_CURVE('',#7301,#7302,#1338,.T.);
#9434=EDGE_CURVE('',#7302,#7303,#1339,.T.);
#9435=EDGE_CURVE('',#7303,#7300,#4898,.T.);
#9436=EDGE_CURVE('',#7301,#7304,#1952,.T.);
#9437=EDGE_CURVE('',#7305,#7304,#1340,.T.);
#9438=EDGE_CURVE('',#7305,#6538,#603,.T.);
#9439=EDGE_CURVE('',#7302,#6537,#604,.T.);
#9440=EDGE_CURVE('',#7306,#7299,#1953,.T.);
#9441=EDGE_CURVE('',#7304,#7306,#4899,.T.);
#9442=EDGE_CURVE('',#7306,#7307,#4900,.F.);
#9443=EDGE_CURVE('',#7307,#7308,#4901,.T.);
#9444=EDGE_CURVE('',#7308,#7305,#1341,.T.);
#9445=EDGE_CURVE('',#7309,#7310,#4902,.T.);
#9446=EDGE_CURVE('',#7309,#7311,#4903,.T.);
#9447=EDGE_CURVE('',#7311,#7312,#1342,.T.);
#9448=EDGE_CURVE('',#7312,#7313,#1343,.T.);
#9449=EDGE_CURVE('',#7313,#7310,#4904,.T.);
#9450=EDGE_CURVE('',#7311,#7314,#1954,.T.);
#9451=EDGE_CURVE('',#7315,#7314,#1344,.T.);
#9452=EDGE_CURVE('',#7315,#6540,#605,.T.);
#9453=EDGE_CURVE('',#7312,#6539,#606,.T.);
#9454=EDGE_CURVE('',#7316,#7309,#1955,.T.);
#9455=EDGE_CURVE('',#7314,#7316,#4905,.T.);
#9456=EDGE_CURVE('',#7316,#7317,#4906,.F.);
#9457=EDGE_CURVE('',#7317,#7318,#4907,.T.);
#9458=EDGE_CURVE('',#7318,#7315,#1345,.T.);
#9459=EDGE_CURVE('',#7319,#7320,#4908,.T.);
#9460=EDGE_CURVE('',#7319,#7321,#4909,.T.);
#9461=EDGE_CURVE('',#7321,#7322,#1346,.T.);
#9462=EDGE_CURVE('',#7322,#7323,#1347,.T.);
#9463=EDGE_CURVE('',#7323,#7320,#4910,.T.);
#9464=EDGE_CURVE('',#7321,#7324,#1956,.T.);
#9465=EDGE_CURVE('',#7325,#7324,#1348,.T.);
#9466=EDGE_CURVE('',#7325,#6542,#607,.T.);
#9467=EDGE_CURVE('',#7322,#6541,#608,.T.);
#9468=EDGE_CURVE('',#7326,#7319,#1957,.T.);
#9469=EDGE_CURVE('',#7324,#7326,#4911,.T.);
#9470=EDGE_CURVE('',#6344,#7327,#4912,.T.);
#9471=EDGE_CURVE('',#6347,#7328,#1349,.T.);
#9472=EDGE_CURVE('',#7328,#7327,#4913,.T.);
#9473=EDGE_CURVE('',#7329,#7328,#1958,.T.);
#9474=EDGE_CURVE('',#7330,#7329,#4914,.T.);
#9475=EDGE_CURVE('',#7330,#7327,#1959,.T.);
#9476=EDGE_CURVE('',#7329,#7325,#1350,.T.);
#9477=EDGE_CURVE('',#7326,#7330,#4915,.F.);
#9478=EDGE_CURVE('',#7248,#7253,#1960,.T.);
#9479=EDGE_CURVE('',#7258,#7263,#1961,.T.);
#9480=EDGE_CURVE('',#7268,#7273,#1962,.T.);
#9481=EDGE_CURVE('',#7278,#7283,#1963,.T.);
#9482=EDGE_CURVE('',#7288,#7293,#1964,.T.);
#9483=EDGE_CURVE('',#7298,#7303,#1965,.T.);
#9484=EDGE_CURVE('',#7308,#7313,#1966,.T.);
#9485=EDGE_CURVE('',#7318,#7323,#1967,.T.);
#9486=EDGE_CURVE('',#7317,#7320,#1968,.T.);
#9487=EDGE_CURVE('',#7307,#7310,#1969,.T.);
#9488=EDGE_CURVE('',#7297,#7300,#1970,.T.);
#9489=EDGE_CURVE('',#7287,#7290,#1971,.T.);
#9490=EDGE_CURVE('',#7277,#7280,#1972,.T.);
#9491=EDGE_CURVE('',#7267,#7270,#1973,.T.);
#9492=EDGE_CURVE('',#7257,#7260,#1974,.T.);
#9493=EDGE_CURVE('',#7247,#7250,#1975,.T.);
#9494=EDGE_CURVE('',#7331,#7331,#1976,.T.);
#9495=EDGE_CURVE('',#7331,#6662,#4916,.T.);
#9496=EDGE_CURVE('',#7332,#7332,#1977,.T.);
#9497=EDGE_CURVE('',#7332,#7331,#4917,.T.);
#9498=EDGE_CURVE('',#6412,#7333,#4918,.T.);
#9499=EDGE_CURVE('',#6409,#7333,#4919,.T.);
#9500=EDGE_CURVE('',#6407,#6417,#1978,.T.);
#9501=EDGE_CURVE('',#6424,#6429,#1979,.T.);
#9502=EDGE_CURVE('',#6436,#6441,#1980,.T.);
#9503=EDGE_CURVE('',#6448,#6453,#1981,.T.);
#9504=EDGE_CURVE('',#6460,#6465,#1982,.T.);
#9505=EDGE_CURVE('',#6472,#6477,#1983,.T.);
#9506=EDGE_CURVE('',#6484,#6489,#1984,.T.);
#9507=EDGE_CURVE('',#6496,#6501,#1985,.T.);
#9508=EDGE_CURVE('',#6507,#7242,#1986,.T.);
#9509=EDGE_CURVE('',#6495,#6498,#1987,.T.);
#9510=EDGE_CURVE('',#6483,#6486,#1988,.T.);
#9511=EDGE_CURVE('',#6471,#6474,#1989,.T.);
#9512=EDGE_CURVE('',#6459,#6462,#1990,.T.);
#9513=EDGE_CURVE('',#6447,#6450,#1991,.T.);
#9514=EDGE_CURVE('',#6435,#6438,#1992,.T.);
#9515=EDGE_CURVE('',#6423,#6426,#1993,.T.);
#9516=EDGE_CURVE('',#6406,#6414,#1994,.T.);
#9517=EDGE_CURVE('',#6400,#7334,#4920,.T.);
#9518=EDGE_CURVE('',#7334,#7335,#4921,.F.);
#9519=EDGE_CURVE('',#7335,#6401,#4922,.T.);
#9520=EDGE_CURVE('',#7335,#7333,#1995,.T.);
#9521=EDGE_CURVE('',#7336,#6664,#4923,.T.);
#9522=EDGE_CURVE('',#7336,#7337,#4924,.T.);
#9523=EDGE_CURVE('',#7337,#6665,#609,.T.);
#9524=EDGE_CURVE('',#7337,#7338,#1996,.T.);
#9525=EDGE_CURVE('',#7338,#7339,#610,.T.);
#9526=EDGE_CURVE('',#7339,#6516,#611,.T.);
#9527=EDGE_CURVE('',#7338,#7340,#4925,.T.);
#9528=EDGE_CURVE('',#7340,#7341,#4926,.F.);
#9529=EDGE_CURVE('',#7341,#7339,#4927,.T.);
#9530=EDGE_CURVE('',#7341,#7342,#1997,.T.);
#9531=EDGE_CURVE('',#7343,#7342,#4928,.T.);
#9532=EDGE_CURVE('',#6517,#7343,#612,.T.);
#9533=EDGE_CURVE('',#7344,#7345,#4929,.T.);
#9534=EDGE_CURVE('',#7346,#7345,#4930,.T.);
#9535=EDGE_CURVE('',#7346,#7347,#4931,.T.);
#9536=EDGE_CURVE('',#7347,#7344,#613,.T.);
#9537=EDGE_CURVE('',#7347,#7348,#1998,.T.);
#9538=EDGE_CURVE('',#7348,#6398,#614,.T.);
#9539=EDGE_CURVE('',#6525,#7344,#615,.T.);
#9540=EDGE_CURVE('',#7348,#7349,#4932,.T.);
#9541=EDGE_CURVE('',#7349,#6399,#4933,.F.);
#9542=EDGE_CURVE('',#7350,#6524,#616,.T.);
#9543=EDGE_CURVE('',#7351,#7350,#4934,.T.);
#9544=EDGE_CURVE('',#7351,#7345,#1999,.T.);
#9545=EDGE_CURVE('',#7352,#7342,#4935,.T.);
#9546=EDGE_CURVE('',#7352,#7353,#4936,.T.);
#9547=EDGE_CURVE('',#7353,#7343,#617,.T.);
#9548=EDGE_CURVE('',#7353,#7354,#2000,.T.);
#9549=EDGE_CURVE('',#7354,#7355,#618,.T.);
#9550=EDGE_CURVE('',#7355,#6518,#619,.T.);
#9551=EDGE_CURVE('',#7354,#7356,#4937,.T.);
#9552=EDGE_CURVE('',#7356,#7357,#4938,.F.);
#9553=EDGE_CURVE('',#7357,#7355,#4939,.T.);
#9554=EDGE_CURVE('',#7357,#7358,#2001,.T.);
#9555=EDGE_CURVE('',#7359,#7358,#4940,.T.);
#9556=EDGE_CURVE('',#6519,#7359,#620,.T.);
#9557=EDGE_CURVE('',#7360,#7361,#4941,.T.);
#9558=EDGE_CURVE('',#7362,#7361,#4942,.T.);
#9559=EDGE_CURVE('',#7362,#7363,#4943,.T.);
#9560=EDGE_CURVE('',#7363,#7360,#621,.T.);
#9561=EDGE_CURVE('',#7363,#7364,#2002,.T.);
#9562=EDGE_CURVE('',#7364,#7350,#622,.T.);
#9563=EDGE_CURVE('',#6523,#7360,#623,.T.);
#9564=EDGE_CURVE('',#7364,#7365,#4944,.T.);
#9565=EDGE_CURVE('',#7365,#7351,#4945,.F.);
#9566=EDGE_CURVE('',#7366,#6522,#624,.T.);
#9567=EDGE_CURVE('',#7367,#7366,#4946,.T.);
#9568=EDGE_CURVE('',#7367,#7361,#2003,.T.);
#9569=EDGE_CURVE('',#7368,#7358,#4947,.T.);
#9570=EDGE_CURVE('',#7368,#7369,#4948,.T.);
#9571=EDGE_CURVE('',#7369,#7359,#625,.T.);
#9572=EDGE_CURVE('',#7369,#7370,#2004,.T.);
#9573=EDGE_CURVE('',#7370,#7371,#626,.T.);
#9574=EDGE_CURVE('',#7371,#6520,#627,.T.);
#9575=EDGE_CURVE('',#7370,#7372,#4949,.T.);
#9576=EDGE_CURVE('',#7372,#7373,#4950,.F.);
#9577=EDGE_CURVE('',#7373,#7371,#4951,.T.);
#9578=EDGE_CURVE('',#7373,#7374,#2005,.T.);
#9579=EDGE_CURVE('',#7375,#7374,#4952,.T.);
#9580=EDGE_CURVE('',#6521,#7375,#628,.T.);
#9581=EDGE_CURVE('',#7376,#7374,#4953,.T.);
#9582=EDGE_CURVE('',#7376,#7377,#4954,.T.);
#9583=EDGE_CURVE('',#7377,#7375,#629,.T.);
#9584=EDGE_CURVE('',#7377,#7378,#2006,.T.);
#9585=EDGE_CURVE('',#7378,#7366,#630,.T.);
#9586=EDGE_CURVE('',#7378,#7379,#4955,.T.);
#9587=EDGE_CURVE('',#7379,#7367,#4956,.F.);
#9588=EDGE_CURVE('',#7380,#7380,#2007,.T.);
#9589=EDGE_CURVE('',#7380,#7381,#4957,.T.);
#9590=EDGE_CURVE('',#7381,#7381,#2008,.T.);
#9591=EDGE_CURVE('',#7382,#7382,#2009,.T.);
#9592=EDGE_CURVE('',#7380,#7383,#4958,.T.);
#9593=EDGE_CURVE('',#7383,#7379,#2010,.T.);
#9594=EDGE_CURVE('',#7379,#7376,#2011,.T.);
#9595=EDGE_CURVE('',#7376,#7372,#2012,.T.);
#9596=EDGE_CURVE('',#7372,#7368,#2013,.T.);
#9597=EDGE_CURVE('',#7368,#7356,#2014,.T.);
#9598=EDGE_CURVE('',#7356,#7352,#2015,.T.);
#9599=EDGE_CURVE('',#7352,#7340,#2016,.T.);
#9600=EDGE_CURVE('',#7340,#7336,#2017,.T.);
#9601=EDGE_CURVE('',#7336,#6666,#2018,.T.);
#9602=EDGE_CURVE('',#6666,#6390,#2019,.T.);
#9603=EDGE_CURVE('',#6390,#6380,#2020,.T.);
#9604=EDGE_CURVE('',#6380,#6388,#2021,.T.);
#9605=EDGE_CURVE('',#6388,#6364,#2022,.T.);
#9606=EDGE_CURVE('',#6364,#6372,#2023,.T.);
#9607=EDGE_CURVE('',#6372,#6350,#2024,.T.);
#9608=EDGE_CURVE('',#6354,#6696,#2025,.T.);
#9609=EDGE_CURVE('',#6698,#6689,#2026,.T.);
#9610=EDGE_CURVE('',#6685,#6679,#2027,.T.);
#9611=EDGE_CURVE('',#6675,#6669,#2028,.T.);
#9612=EDGE_CURVE('',#6758,#6755,#2029,.T.);
#9613=EDGE_CURVE('',#6748,#6745,#2030,.T.);
#9614=EDGE_CURVE('',#6738,#6735,#2031,.T.);
#9615=EDGE_CURVE('',#6728,#6725,#2032,.T.);
#9616=EDGE_CURVE('',#6718,#6715,#2033,.T.);
#9617=EDGE_CURVE('',#6708,#6705,#2034,.T.);
#9618=EDGE_CURVE('',#6699,#6801,#2035,.T.);
#9619=EDGE_CURVE('',#6804,#6793,#2036,.T.);
#9620=EDGE_CURVE('',#6789,#6783,#2037,.T.);
#9621=EDGE_CURVE('',#6779,#6773,#2038,.T.);
#9622=EDGE_CURVE('',#6769,#6763,#2039,.T.);
#9623=EDGE_CURVE('',#6854,#6851,#2040,.T.);
#9624=EDGE_CURVE('',#6844,#6841,#2041,.T.);
#9625=EDGE_CURVE('',#6834,#6831,#2042,.T.);
#9626=EDGE_CURVE('',#6824,#6821,#2043,.T.);
#9627=EDGE_CURVE('',#6814,#6811,#2044,.T.);
#9628=EDGE_CURVE('',#6805,#6907,#2045,.T.);
#9629=EDGE_CURVE('',#6910,#6899,#2046,.T.);
#9630=EDGE_CURVE('',#6895,#6889,#2047,.T.);
#9631=EDGE_CURVE('',#6885,#6879,#2048,.T.);
#9632=EDGE_CURVE('',#6875,#6869,#2049,.T.);
#9633=EDGE_CURVE('',#6865,#6859,#2050,.T.);
#9634=EDGE_CURVE('',#6950,#6947,#2051,.T.);
#9635=EDGE_CURVE('',#6940,#6937,#2052,.T.);
#9636=EDGE_CURVE('',#6930,#6927,#2053,.T.);
#9637=EDGE_CURVE('',#6920,#6917,#2054,.T.);
#9638=EDGE_CURVE('',#6911,#7013,#2055,.T.);
#9639=EDGE_CURVE('',#7016,#7005,#2056,.T.);
#9640=EDGE_CURVE('',#7001,#6995,#2057,.T.);
#9641=EDGE_CURVE('',#6991,#6985,#2058,.T.);
#9642=EDGE_CURVE('',#6981,#6975,#2059,.T.);
#9643=EDGE_CURVE('',#6971,#6965,#2060,.T.);
#9644=EDGE_CURVE('',#6961,#6955,#2061,.T.);
#9645=EDGE_CURVE('',#7046,#7043,#2062,.T.);
#9646=EDGE_CURVE('',#7036,#7033,#2063,.T.);
#9647=EDGE_CURVE('',#7026,#7023,#2064,.T.);
#9648=EDGE_CURVE('',#7017,#7119,#2065,.T.);
#9649=EDGE_CURVE('',#7122,#7111,#2066,.T.);
#9650=EDGE_CURVE('',#7107,#7101,#2067,.T.);
#9651=EDGE_CURVE('',#7097,#7091,#2068,.T.);
#9652=EDGE_CURVE('',#7087,#7081,#2069,.T.);
#9653=EDGE_CURVE('',#7077,#7071,#2070,.T.);
#9654=EDGE_CURVE('',#7067,#7061,#2071,.T.);
#9655=EDGE_CURVE('',#7057,#7051,#2072,.T.);
#9656=EDGE_CURVE('',#7142,#7139,#2073,.T.);
#9657=EDGE_CURVE('',#7132,#7129,#2074,.T.);
#9658=EDGE_CURVE('',#7123,#7225,#2075,.T.);
#9659=EDGE_CURVE('',#7228,#7217,#2076,.T.);
#9660=EDGE_CURVE('',#7213,#7207,#2077,.T.);
#9661=EDGE_CURVE('',#7203,#7197,#2078,.T.);
#9662=EDGE_CURVE('',#7193,#7187,#2079,.T.);
#9663=EDGE_CURVE('',#7183,#7177,#2080,.T.);
#9664=EDGE_CURVE('',#7173,#7167,#2081,.T.);
#9665=EDGE_CURVE('',#7163,#7157,#2082,.T.);
#9666=EDGE_CURVE('',#7153,#7147,#2083,.T.);
#9667=EDGE_CURVE('',#7238,#7235,#2084,.T.);
#9668=EDGE_CURVE('',#7229,#6341,#2085,.T.);
#9669=EDGE_CURVE('',#6344,#7326,#2086,.T.);
#9670=EDGE_CURVE('',#7319,#7316,#2087,.T.);
#9671=EDGE_CURVE('',#7309,#7306,#2088,.T.);
#9672=EDGE_CURVE('',#7299,#7296,#2089,.T.);
#9673=EDGE_CURVE('',#7289,#7286,#2090,.T.);
#9674=EDGE_CURVE('',#7279,#7276,#2091,.T.);
#9675=EDGE_CURVE('',#7269,#7266,#2092,.T.);
#9676=EDGE_CURVE('',#7259,#7256,#2093,.T.);
#9677=EDGE_CURVE('',#7249,#7246,#2094,.T.);
#9678=EDGE_CURVE('',#7241,#6506,#2095,.T.);
#9679=EDGE_CURVE('',#6497,#6494,#2096,.T.);
#9680=EDGE_CURVE('',#6485,#6482,#2097,.T.);
#9681=EDGE_CURVE('',#6473,#6470,#2098,.T.);
#9682=EDGE_CURVE('',#6461,#6458,#2099,.T.);
#9683=EDGE_CURVE('',#6449,#6446,#2100,.T.);
#9684=EDGE_CURVE('',#6437,#6434,#2101,.T.);
#9685=EDGE_CURVE('',#6425,#6422,#2102,.T.);
#9686=EDGE_CURVE('',#6413,#6405,#2103,.T.);
#9687=EDGE_CURVE('',#6409,#7334,#2104,.T.);
#9688=EDGE_CURVE('',#7334,#6392,#2105,.T.);
#9689=EDGE_CURVE('',#6392,#7349,#2106,.T.);
#9690=EDGE_CURVE('',#7349,#7346,#2107,.T.);
#9691=EDGE_CURVE('',#7346,#7365,#2108,.T.);
#9692=EDGE_CURVE('',#7365,#7362,#2109,.T.);
#9693=EDGE_CURVE('',#7362,#7383,#2110,.T.);
#9694=EDGE_CURVE('',#7384,#7384,#2111,.T.);
#9695=EDGE_CURVE('',#7384,#7385,#4959,.T.);
#9696=EDGE_CURVE('',#7385,#7385,#2112,.T.);
#9697=EDGE_CURVE('',#7386,#7386,#2113,.T.);
#9698=EDGE_CURVE('',#7387,#7387,#2114,.T.);
#9699=EDGE_CURVE('',#7388,#7388,#2115,.T.);
#9700=EDGE_CURVE('',#7389,#7389,#2116,.T.);
#9701=EDGE_CURVE('',#7390,#7390,#2117,.T.);
#9702=EDGE_CURVE('',#7391,#7391,#2118,.T.);
#9703=EDGE_CURVE('',#7385,#7392,#4960,.T.);
#9704=EDGE_CURVE('',#7392,#7392,#2119,.T.);
#9705=EDGE_CURVE('',#7387,#7393,#4961,.T.);
#9706=EDGE_CURVE('',#7393,#7393,#2120,.T.);
#9707=EDGE_CURVE('',#7393,#7394,#4962,.T.);
#9708=EDGE_CURVE('',#7394,#7394,#2121,.T.);
#9709=EDGE_CURVE('',#7391,#7395,#4963,.T.);
#9710=EDGE_CURVE('',#7395,#7395,#2122,.T.);
#9711=EDGE_CURVE('',#7395,#7396,#4964,.T.);
#9712=EDGE_CURVE('',#7396,#7396,#2123,.T.);
#9713=EDGE_CURVE('',#7388,#7397,#4965,.T.);
#9714=EDGE_CURVE('',#7397,#7397,#2124,.T.);
#9715=EDGE_CURVE('',#7397,#7398,#4966,.T.);
#9716=EDGE_CURVE('',#7398,#7398,#2125,.T.);
#9717=EDGE_CURVE('',#7390,#7399,#4967,.T.);
#9718=EDGE_CURVE('',#7399,#7399,#2126,.T.);
#9719=EDGE_CURVE('',#7399,#7400,#4968,.T.);
#9720=EDGE_CURVE('',#7400,#7400,#2127,.T.);
#9721=EDGE_CURVE('',#7382,#7401,#4969,.T.);
#9722=EDGE_CURVE('',#7401,#7401,#2128,.T.);
#9723=EDGE_CURVE('',#7401,#7386,#4970,.T.);
#9724=EDGE_CURVE('',#7014,#6912,#2129,.T.);
#9725=EDGE_CURVE('',#6908,#6806,#2130,.T.);
#9726=EDGE_CURVE('',#6802,#6700,#2131,.T.);
#9727=EDGE_CURVE('',#6342,#7230,#2132,.T.);
#9728=EDGE_CURVE('',#7226,#7124,#2133,.T.);
#9729=EDGE_CURVE('',#7120,#7018,#2134,.T.);
#9730=EDGE_CURVE('',#7402,#7402,#2135,.T.);
#9731=EDGE_CURVE('',#7402,#7403,#4971,.T.);
#9732=EDGE_CURVE('',#7404,#7404,#2136,.T.);
#9733=EDGE_CURVE('',#7404,#7405,#4972,.T.);
#9734=EDGE_CURVE('',#7406,#7406,#2137,.T.);
#9735=EDGE_CURVE('',#7406,#7407,#4973,.T.);
#9736=EDGE_CURVE('',#7408,#7408,#2138,.T.);
#9737=EDGE_CURVE('',#7408,#7409,#4974,.T.);
#9738=EDGE_CURVE('',#7410,#7410,#2139,.T.);
#9739=EDGE_CURVE('',#7410,#7411,#4975,.T.);
#9740=EDGE_CURVE('',#7389,#7412,#4976,.T.);
#9741=EDGE_CURVE('',#7412,#7412,#2140,.T.);
#10781=ORIENTED_EDGE('',*,*,#8042,.T.);
#10782=ORIENTED_EDGE('',*,*,#8043,.T.);
#10783=ORIENTED_EDGE('',*,*,#8044,.T.);
#10784=ORIENTED_EDGE('',*,*,#8045,.T.);
#10785=ORIENTED_EDGE('',*,*,#8043,.F.);
#10786=ORIENTED_EDGE('',*,*,#8046,.F.);
#10787=ORIENTED_EDGE('',*,*,#8047,.F.);
#10788=ORIENTED_EDGE('',*,*,#8048,.F.);
#10789=ORIENTED_EDGE('',*,*,#8042,.F.);
#10790=ORIENTED_EDGE('',*,*,#8049,.F.);
#10791=ORIENTED_EDGE('',*,*,#8050,.T.);
#10792=ORIENTED_EDGE('',*,*,#8051,.T.);
#10793=ORIENTED_EDGE('',*,*,#8052,.F.);
#10794=ORIENTED_EDGE('',*,*,#8046,.T.);
#10795=ORIENTED_EDGE('',*,*,#8053,.T.);
#10796=ORIENTED_EDGE('',*,*,#8054,.T.);
#10797=ORIENTED_EDGE('',*,*,#8055,.T.);
#10798=ORIENTED_EDGE('',*,*,#8056,.T.);
#10799=ORIENTED_EDGE('',*,*,#8057,.T.);
#10800=ORIENTED_EDGE('',*,*,#8054,.F.);
#10801=ORIENTED_EDGE('',*,*,#8058,.F.);
#10802=ORIENTED_EDGE('',*,*,#8059,.F.);
#10803=ORIENTED_EDGE('',*,*,#8060,.F.);
#10804=ORIENTED_EDGE('',*,*,#8053,.F.);
#10805=ORIENTED_EDGE('',*,*,#8061,.T.);
#10806=ORIENTED_EDGE('',*,*,#8062,.T.);
#10807=ORIENTED_EDGE('',*,*,#8063,.F.);
#10808=ORIENTED_EDGE('',*,*,#8064,.F.);
#10809=ORIENTED_EDGE('',*,*,#8058,.T.);
#10810=ORIENTED_EDGE('',*,*,#8065,.F.);
#10811=ORIENTED_EDGE('',*,*,#8059,.T.);
#10812=ORIENTED_EDGE('',*,*,#8064,.T.);
#10813=ORIENTED_EDGE('',*,*,#8066,.T.);
#10814=ORIENTED_EDGE('',*,*,#8066,.F.);
#10815=ORIENTED_EDGE('',*,*,#8063,.T.);
#10816=ORIENTED_EDGE('',*,*,#8067,.F.);
#10817=ORIENTED_EDGE('',*,*,#8068,.T.);
#10818=ORIENTED_EDGE('',*,*,#8069,.F.);
#10819=ORIENTED_EDGE('',*,*,#8070,.T.);
#10820=ORIENTED_EDGE('',*,*,#8071,.T.);
#10821=ORIENTED_EDGE('',*,*,#8072,.T.);
#10822=ORIENTED_EDGE('',*,*,#8073,.T.);
#10823=ORIENTED_EDGE('',*,*,#8074,.T.);
#10824=ORIENTED_EDGE('',*,*,#8075,.T.);
#10825=ORIENTED_EDGE('',*,*,#8075,.F.);
#10826=ORIENTED_EDGE('',*,*,#8076,.T.);
#10827=ORIENTED_EDGE('',*,*,#8077,.F.);
#10828=ORIENTED_EDGE('',*,*,#8078,.T.);
#10829=ORIENTED_EDGE('',*,*,#8079,.T.);
#10830=ORIENTED_EDGE('',*,*,#8080,.F.);
#10831=ORIENTED_EDGE('',*,*,#8074,.F.);
#10832=ORIENTED_EDGE('',*,*,#8081,.T.);
#10833=ORIENTED_EDGE('',*,*,#8082,.F.);
#10834=ORIENTED_EDGE('',*,*,#8076,.F.);
#10835=ORIENTED_EDGE('',*,*,#8083,.F.);
#10836=ORIENTED_EDGE('',*,*,#8084,.T.);
#10837=ORIENTED_EDGE('',*,*,#8085,.T.);
#10838=ORIENTED_EDGE('',*,*,#8086,.T.);
#10839=ORIENTED_EDGE('',*,*,#8087,.T.);
#10840=ORIENTED_EDGE('',*,*,#8056,.F.);
#10841=ORIENTED_EDGE('',*,*,#8088,.T.);
#10842=ORIENTED_EDGE('',*,*,#8087,.F.);
#10843=ORIENTED_EDGE('',*,*,#8089,.F.);
#10844=ORIENTED_EDGE('',*,*,#8057,.F.);
#10845=ORIENTED_EDGE('',*,*,#8089,.T.);
#10846=ORIENTED_EDGE('',*,*,#8086,.F.);
#10847=ORIENTED_EDGE('',*,*,#8090,.T.);
#10848=ORIENTED_EDGE('',*,*,#8091,.T.);
#10849=ORIENTED_EDGE('',*,*,#8061,.F.);
#10850=ORIENTED_EDGE('',*,*,#8092,.T.);
#10851=ORIENTED_EDGE('',*,*,#8093,.T.);
#10852=ORIENTED_EDGE('',*,*,#8094,.T.);
#10853=ORIENTED_EDGE('',*,*,#8095,.T.);
#10854=ORIENTED_EDGE('',*,*,#8096,.T.);
#10855=ORIENTED_EDGE('',*,*,#8096,.F.);
#10856=ORIENTED_EDGE('',*,*,#8097,.T.);
#10857=ORIENTED_EDGE('',*,*,#8098,.F.);
#10858=ORIENTED_EDGE('',*,*,#8099,.T.);
#10859=ORIENTED_EDGE('',*,*,#8100,.T.);
#10860=ORIENTED_EDGE('',*,*,#8101,.F.);
#10861=ORIENTED_EDGE('',*,*,#8095,.F.);
#10862=ORIENTED_EDGE('',*,*,#8102,.T.);
#10863=ORIENTED_EDGE('',*,*,#8103,.F.);
#10864=ORIENTED_EDGE('',*,*,#8097,.F.);
#10865=ORIENTED_EDGE('',*,*,#8104,.F.);
#10866=ORIENTED_EDGE('',*,*,#8105,.T.);
#10867=ORIENTED_EDGE('',*,*,#8106,.T.);
#10868=ORIENTED_EDGE('',*,*,#8077,.T.);
#10869=ORIENTED_EDGE('',*,*,#8082,.T.);
#10870=ORIENTED_EDGE('',*,*,#8107,.F.);
#10871=ORIENTED_EDGE('',*,*,#8108,.T.);
#10872=ORIENTED_EDGE('',*,*,#8109,.T.);
#10873=ORIENTED_EDGE('',*,*,#8098,.T.);
#10874=ORIENTED_EDGE('',*,*,#8103,.T.);
#10875=ORIENTED_EDGE('',*,*,#8110,.F.);
#10876=ORIENTED_EDGE('',*,*,#8111,.T.);
#10877=ORIENTED_EDGE('',*,*,#8112,.T.);
#10878=ORIENTED_EDGE('',*,*,#8113,.T.);
#10879=ORIENTED_EDGE('',*,*,#8113,.F.);
#10880=ORIENTED_EDGE('',*,*,#8114,.T.);
#10881=ORIENTED_EDGE('',*,*,#8115,.F.);
#10882=ORIENTED_EDGE('',*,*,#8116,.F.);
#10883=ORIENTED_EDGE('',*,*,#8117,.F.);
#10884=ORIENTED_EDGE('',*,*,#8118,.T.);
#10885=ORIENTED_EDGE('',*,*,#8112,.F.);
#10886=ORIENTED_EDGE('',*,*,#8119,.T.);
#10887=ORIENTED_EDGE('',*,*,#8120,.T.);
#10888=ORIENTED_EDGE('',*,*,#8121,.T.);
#10889=ORIENTED_EDGE('',*,*,#8122,.T.);
#10890=ORIENTED_EDGE('',*,*,#8114,.F.);
#10891=ORIENTED_EDGE('',*,*,#8123,.T.);
#10892=ORIENTED_EDGE('',*,*,#8124,.T.);
#10893=ORIENTED_EDGE('',*,*,#8125,.T.);
#10894=ORIENTED_EDGE('',*,*,#8126,.T.);
#10895=ORIENTED_EDGE('',*,*,#8127,.T.);
#10896=ORIENTED_EDGE('',*,*,#8124,.F.);
#10897=ORIENTED_EDGE('',*,*,#8128,.F.);
#10898=ORIENTED_EDGE('',*,*,#8129,.F.);
#10899=ORIENTED_EDGE('',*,*,#8130,.F.);
#10900=ORIENTED_EDGE('',*,*,#8123,.F.);
#10901=ORIENTED_EDGE('',*,*,#8131,.T.);
#10902=ORIENTED_EDGE('',*,*,#8132,.T.);
#10903=ORIENTED_EDGE('',*,*,#8133,.T.);
#10904=ORIENTED_EDGE('',*,*,#8134,.F.);
#10905=ORIENTED_EDGE('',*,*,#8128,.T.);
#10906=ORIENTED_EDGE('',*,*,#8135,.F.);
#10907=ORIENTED_EDGE('',*,*,#8136,.T.);
#10908=ORIENTED_EDGE('',*,*,#8137,.T.);
#10909=ORIENTED_EDGE('',*,*,#8138,.T.);
#10910=ORIENTED_EDGE('',*,*,#8139,.T.);
#10911=ORIENTED_EDGE('',*,*,#8137,.F.);
#10912=ORIENTED_EDGE('',*,*,#8140,.T.);
#10913=ORIENTED_EDGE('',*,*,#8141,.F.);
#10914=ORIENTED_EDGE('',*,*,#8142,.T.);
#10915=ORIENTED_EDGE('',*,*,#8143,.T.);
#10916=ORIENTED_EDGE('',*,*,#8144,.F.);
#10917=ORIENTED_EDGE('',*,*,#8136,.F.);
#10918=ORIENTED_EDGE('',*,*,#8145,.F.);
#10919=ORIENTED_EDGE('',*,*,#8146,.F.);
#10920=ORIENTED_EDGE('',*,*,#8140,.F.);
#10921=ORIENTED_EDGE('',*,*,#8141,.T.);
#10922=ORIENTED_EDGE('',*,*,#8146,.T.);
#10923=ORIENTED_EDGE('',*,*,#8147,.T.);
#10924=ORIENTED_EDGE('',*,*,#8148,.T.);
#10925=ORIENTED_EDGE('',*,*,#8149,.T.);
#10926=ORIENTED_EDGE('',*,*,#8150,.F.);
#10927=ORIENTED_EDGE('',*,*,#8151,.T.);
#10928=ORIENTED_EDGE('',*,*,#8152,.T.);
#10929=ORIENTED_EDGE('',*,*,#8153,.T.);
#10930=ORIENTED_EDGE('',*,*,#8154,.T.);
#10931=ORIENTED_EDGE('',*,*,#8152,.F.);
#10932=ORIENTED_EDGE('',*,*,#8155,.T.);
#10933=ORIENTED_EDGE('',*,*,#8156,.F.);
#10934=ORIENTED_EDGE('',*,*,#8157,.T.);
#10935=ORIENTED_EDGE('',*,*,#8158,.T.);
#10936=ORIENTED_EDGE('',*,*,#8159,.F.);
#10937=ORIENTED_EDGE('',*,*,#8151,.F.);
#10938=ORIENTED_EDGE('',*,*,#8160,.F.);
#10939=ORIENTED_EDGE('',*,*,#8161,.F.);
#10940=ORIENTED_EDGE('',*,*,#8155,.F.);
#10941=ORIENTED_EDGE('',*,*,#8156,.T.);
#10942=ORIENTED_EDGE('',*,*,#8161,.T.);
#10943=ORIENTED_EDGE('',*,*,#8162,.T.);
#10944=ORIENTED_EDGE('',*,*,#8163,.T.);
#10945=ORIENTED_EDGE('',*,*,#8164,.T.);
#10946=ORIENTED_EDGE('',*,*,#8165,.F.);
#10947=ORIENTED_EDGE('',*,*,#8166,.T.);
#10948=ORIENTED_EDGE('',*,*,#8167,.T.);
#10949=ORIENTED_EDGE('',*,*,#8168,.T.);
#10950=ORIENTED_EDGE('',*,*,#8169,.T.);
#10951=ORIENTED_EDGE('',*,*,#8167,.F.);
#10952=ORIENTED_EDGE('',*,*,#8170,.T.);
#10953=ORIENTED_EDGE('',*,*,#8171,.F.);
#10954=ORIENTED_EDGE('',*,*,#8172,.T.);
#10955=ORIENTED_EDGE('',*,*,#8173,.T.);
#10956=ORIENTED_EDGE('',*,*,#8174,.F.);
#10957=ORIENTED_EDGE('',*,*,#8166,.F.);
#10958=ORIENTED_EDGE('',*,*,#8175,.F.);
#10959=ORIENTED_EDGE('',*,*,#8176,.F.);
#10960=ORIENTED_EDGE('',*,*,#8170,.F.);
#10961=ORIENTED_EDGE('',*,*,#8171,.T.);
#10962=ORIENTED_EDGE('',*,*,#8176,.T.);
#10963=ORIENTED_EDGE('',*,*,#8177,.T.);
#10964=ORIENTED_EDGE('',*,*,#8178,.T.);
#10965=ORIENTED_EDGE('',*,*,#8179,.T.);
#10966=ORIENTED_EDGE('',*,*,#8180,.F.);
#10967=ORIENTED_EDGE('',*,*,#8181,.T.);
#10968=ORIENTED_EDGE('',*,*,#8182,.T.);
#10969=ORIENTED_EDGE('',*,*,#8183,.T.);
#10970=ORIENTED_EDGE('',*,*,#8184,.T.);
#10971=ORIENTED_EDGE('',*,*,#8182,.F.);
#10972=ORIENTED_EDGE('',*,*,#8185,.T.);
#10973=ORIENTED_EDGE('',*,*,#8186,.F.);
#10974=ORIENTED_EDGE('',*,*,#8187,.T.);
#10975=ORIENTED_EDGE('',*,*,#8188,.T.);
#10976=ORIENTED_EDGE('',*,*,#8189,.F.);
#10977=ORIENTED_EDGE('',*,*,#8181,.F.);
#10978=ORIENTED_EDGE('',*,*,#8190,.F.);
#10979=ORIENTED_EDGE('',*,*,#8191,.F.);
#10980=ORIENTED_EDGE('',*,*,#8185,.F.);
#10981=ORIENTED_EDGE('',*,*,#8186,.T.);
#10982=ORIENTED_EDGE('',*,*,#8191,.T.);
#10983=ORIENTED_EDGE('',*,*,#8192,.T.);
#10984=ORIENTED_EDGE('',*,*,#8193,.T.);
#10985=ORIENTED_EDGE('',*,*,#8194,.T.);
#10986=ORIENTED_EDGE('',*,*,#8195,.F.);
#10987=ORIENTED_EDGE('',*,*,#8196,.T.);
#10988=ORIENTED_EDGE('',*,*,#8197,.T.);
#10989=ORIENTED_EDGE('',*,*,#8198,.T.);
#10990=ORIENTED_EDGE('',*,*,#8199,.T.);
#10991=ORIENTED_EDGE('',*,*,#8197,.F.);
#10992=ORIENTED_EDGE('',*,*,#8200,.T.);
#10993=ORIENTED_EDGE('',*,*,#8201,.F.);
#10994=ORIENTED_EDGE('',*,*,#8202,.T.);
#10995=ORIENTED_EDGE('',*,*,#8203,.T.);
#10996=ORIENTED_EDGE('',*,*,#8204,.F.);
#10997=ORIENTED_EDGE('',*,*,#8196,.F.);
#10998=ORIENTED_EDGE('',*,*,#8205,.F.);
#10999=ORIENTED_EDGE('',*,*,#8206,.F.);
#11000=ORIENTED_EDGE('',*,*,#8200,.F.);
#11001=ORIENTED_EDGE('',*,*,#8201,.T.);
#11002=ORIENTED_EDGE('',*,*,#8206,.T.);
#11003=ORIENTED_EDGE('',*,*,#8207,.T.);
#11004=ORIENTED_EDGE('',*,*,#8208,.T.);
#11005=ORIENTED_EDGE('',*,*,#8209,.T.);
#11006=ORIENTED_EDGE('',*,*,#8210,.F.);
#11007=ORIENTED_EDGE('',*,*,#8211,.T.);
#11008=ORIENTED_EDGE('',*,*,#8212,.T.);
#11009=ORIENTED_EDGE('',*,*,#8213,.T.);
#11010=ORIENTED_EDGE('',*,*,#8214,.T.);
#11011=ORIENTED_EDGE('',*,*,#8212,.F.);
#11012=ORIENTED_EDGE('',*,*,#8215,.T.);
#11013=ORIENTED_EDGE('',*,*,#8216,.F.);
#11014=ORIENTED_EDGE('',*,*,#8217,.T.);
#11015=ORIENTED_EDGE('',*,*,#8218,.T.);
#11016=ORIENTED_EDGE('',*,*,#8219,.F.);
#11017=ORIENTED_EDGE('',*,*,#8211,.F.);
#11018=ORIENTED_EDGE('',*,*,#8220,.F.);
#11019=ORIENTED_EDGE('',*,*,#8221,.F.);
#11020=ORIENTED_EDGE('',*,*,#8215,.F.);
#11021=ORIENTED_EDGE('',*,*,#8216,.T.);
#11022=ORIENTED_EDGE('',*,*,#8221,.T.);
#11023=ORIENTED_EDGE('',*,*,#8222,.T.);
#11024=ORIENTED_EDGE('',*,*,#8223,.T.);
#11025=ORIENTED_EDGE('',*,*,#8224,.T.);
#11026=ORIENTED_EDGE('',*,*,#8225,.F.);
#11027=ORIENTED_EDGE('',*,*,#8226,.T.);
#11028=ORIENTED_EDGE('',*,*,#8227,.T.);
#11029=ORIENTED_EDGE('',*,*,#8228,.T.);
#11030=ORIENTED_EDGE('',*,*,#8229,.T.);
#11031=ORIENTED_EDGE('',*,*,#8227,.F.);
#11032=ORIENTED_EDGE('',*,*,#8230,.T.);
#11033=ORIENTED_EDGE('',*,*,#8231,.F.);
#11034=ORIENTED_EDGE('',*,*,#8232,.T.);
#11035=ORIENTED_EDGE('',*,*,#8233,.T.);
#11036=ORIENTED_EDGE('',*,*,#8234,.F.);
#11037=ORIENTED_EDGE('',*,*,#8226,.F.);
#11038=ORIENTED_EDGE('',*,*,#8235,.F.);
#11039=ORIENTED_EDGE('',*,*,#8236,.F.);
#11040=ORIENTED_EDGE('',*,*,#8230,.F.);
#11041=ORIENTED_EDGE('',*,*,#8231,.T.);
#11042=ORIENTED_EDGE('',*,*,#8236,.T.);
#11043=ORIENTED_EDGE('',*,*,#8237,.T.);
#11044=ORIENTED_EDGE('',*,*,#8238,.T.);
#11045=ORIENTED_EDGE('',*,*,#8239,.T.);
#11046=ORIENTED_EDGE('',*,*,#8240,.F.);
#11047=ORIENTED_EDGE('',*,*,#8241,.T.);
#11048=ORIENTED_EDGE('',*,*,#8242,.T.);
#11049=ORIENTED_EDGE('',*,*,#8243,.T.);
#11050=ORIENTED_EDGE('',*,*,#8244,.T.);
#11051=ORIENTED_EDGE('',*,*,#8242,.F.);
#11052=ORIENTED_EDGE('',*,*,#8245,.T.);
#11053=ORIENTED_EDGE('',*,*,#8246,.F.);
#11054=ORIENTED_EDGE('',*,*,#8247,.T.);
#11055=ORIENTED_EDGE('',*,*,#8248,.T.);
#11056=ORIENTED_EDGE('',*,*,#8249,.F.);
#11057=ORIENTED_EDGE('',*,*,#8241,.F.);
#11058=ORIENTED_EDGE('',*,*,#8250,.F.);
#11059=ORIENTED_EDGE('',*,*,#8251,.F.);
#11060=ORIENTED_EDGE('',*,*,#8245,.F.);
#11061=ORIENTED_EDGE('',*,*,#8246,.T.);
#11062=ORIENTED_EDGE('',*,*,#8251,.T.);
#11063=ORIENTED_EDGE('',*,*,#8252,.T.);
#11064=ORIENTED_EDGE('',*,*,#8253,.T.);
#11065=ORIENTED_EDGE('',*,*,#8254,.T.);
#11066=ORIENTED_EDGE('',*,*,#8254,.F.);
#11067=ORIENTED_EDGE('',*,*,#8255,.T.);
#11068=ORIENTED_EDGE('',*,*,#8256,.F.);
#11069=ORIENTED_EDGE('',*,*,#8257,.F.);
#11070=ORIENTED_EDGE('',*,*,#8258,.T.);
#11071=ORIENTED_EDGE('',*,*,#8247,.F.);
#11072=ORIENTED_EDGE('',*,*,#8071,.F.);
#11073=ORIENTED_EDGE('',*,*,#8080,.T.);
#11074=ORIENTED_EDGE('',*,*,#8259,.T.);
#11075=ORIENTED_EDGE('',*,*,#8090,.F.);
#11076=ORIENTED_EDGE('',*,*,#8085,.F.);
#11077=ORIENTED_EDGE('',*,*,#8260,.T.);
#11078=ORIENTED_EDGE('',*,*,#8092,.F.);
#11079=ORIENTED_EDGE('',*,*,#8101,.T.);
#11080=ORIENTED_EDGE('',*,*,#8261,.T.);
#11081=ORIENTED_EDGE('',*,*,#8078,.F.);
#11082=ORIENTED_EDGE('',*,*,#8106,.F.);
#11083=ORIENTED_EDGE('',*,*,#8262,.T.);
#11084=ORIENTED_EDGE('',*,*,#8109,.F.);
#11085=ORIENTED_EDGE('',*,*,#8263,.T.);
#11086=ORIENTED_EDGE('',*,*,#8264,.T.);
#11087=ORIENTED_EDGE('',*,*,#8265,.F.);
#11088=ORIENTED_EDGE('',*,*,#8266,.T.);
#11089=ORIENTED_EDGE('',*,*,#8099,.F.);
#11090=ORIENTED_EDGE('',*,*,#8062,.F.);
#11091=ORIENTED_EDGE('',*,*,#8091,.F.);
#11092=ORIENTED_EDGE('',*,*,#8259,.F.);
#11093=ORIENTED_EDGE('',*,*,#8079,.F.);
#11094=ORIENTED_EDGE('',*,*,#8261,.F.);
#11095=ORIENTED_EDGE('',*,*,#8100,.F.);
#11096=ORIENTED_EDGE('',*,*,#8266,.F.);
#11097=ORIENTED_EDGE('',*,*,#8267,.T.);
#11098=ORIENTED_EDGE('',*,*,#8268,.F.);
#11099=ORIENTED_EDGE('',*,*,#8269,.T.);
#11100=ORIENTED_EDGE('',*,*,#8270,.F.);
#11101=ORIENTED_EDGE('',*,*,#8271,.T.);
#11102=ORIENTED_EDGE('',*,*,#8272,.F.);
#11103=ORIENTED_EDGE('',*,*,#8273,.T.);
#11104=ORIENTED_EDGE('',*,*,#8274,.F.);
#11105=ORIENTED_EDGE('',*,*,#8275,.T.);
#11106=ORIENTED_EDGE('',*,*,#8276,.F.);
#11107=ORIENTED_EDGE('',*,*,#8277,.T.);
#11108=ORIENTED_EDGE('',*,*,#8278,.F.);
#11109=ORIENTED_EDGE('',*,*,#8115,.T.);
#11110=ORIENTED_EDGE('',*,*,#8122,.F.);
#11111=ORIENTED_EDGE('',*,*,#8279,.T.);
#11112=ORIENTED_EDGE('',*,*,#8132,.F.);
#11113=ORIENTED_EDGE('',*,*,#8280,.F.);
#11114=ORIENTED_EDGE('',*,*,#8143,.F.);
#11115=ORIENTED_EDGE('',*,*,#8281,.F.);
#11116=ORIENTED_EDGE('',*,*,#8158,.F.);
#11117=ORIENTED_EDGE('',*,*,#8282,.F.);
#11118=ORIENTED_EDGE('',*,*,#8173,.F.);
#11119=ORIENTED_EDGE('',*,*,#8283,.F.);
#11120=ORIENTED_EDGE('',*,*,#8188,.F.);
#11121=ORIENTED_EDGE('',*,*,#8284,.F.);
#11122=ORIENTED_EDGE('',*,*,#8203,.F.);
#11123=ORIENTED_EDGE('',*,*,#8285,.F.);
#11124=ORIENTED_EDGE('',*,*,#8218,.F.);
#11125=ORIENTED_EDGE('',*,*,#8286,.F.);
#11126=ORIENTED_EDGE('',*,*,#8233,.F.);
#11127=ORIENTED_EDGE('',*,*,#8287,.F.);
#11128=ORIENTED_EDGE('',*,*,#8248,.F.);
#11129=ORIENTED_EDGE('',*,*,#8258,.F.);
#11130=ORIENTED_EDGE('',*,*,#8288,.F.);
#11131=ORIENTED_EDGE('',*,*,#8289,.F.);
#11132=ORIENTED_EDGE('',*,*,#8290,.F.);
#11133=ORIENTED_EDGE('',*,*,#8291,.F.);
#11134=ORIENTED_EDGE('',*,*,#8292,.F.);
#11135=ORIENTED_EDGE('',*,*,#8293,.F.);
#11136=ORIENTED_EDGE('',*,*,#8294,.F.);
#11137=ORIENTED_EDGE('',*,*,#8295,.F.);
#11138=ORIENTED_EDGE('',*,*,#8296,.F.);
#11139=ORIENTED_EDGE('',*,*,#8297,.F.);
#11140=ORIENTED_EDGE('',*,*,#8298,.F.);
#11141=ORIENTED_EDGE('',*,*,#8299,.F.);
#11142=ORIENTED_EDGE('',*,*,#8300,.F.);
#11143=ORIENTED_EDGE('',*,*,#8301,.F.);
#11144=ORIENTED_EDGE('',*,*,#8302,.F.);
#11145=ORIENTED_EDGE('',*,*,#8303,.F.);
#11146=ORIENTED_EDGE('',*,*,#8304,.F.);
#11147=ORIENTED_EDGE('',*,*,#8305,.F.);
#11148=ORIENTED_EDGE('',*,*,#8050,.F.);
#11149=ORIENTED_EDGE('',*,*,#8306,.T.);
#11150=ORIENTED_EDGE('',*,*,#8307,.F.);
#11151=ORIENTED_EDGE('',*,*,#8308,.T.);
#11152=ORIENTED_EDGE('',*,*,#8309,.F.);
#11153=ORIENTED_EDGE('',*,*,#8310,.F.);
#11154=ORIENTED_EDGE('',*,*,#8311,.F.);
#11155=ORIENTED_EDGE('',*,*,#8312,.F.);
#11156=ORIENTED_EDGE('',*,*,#8313,.F.);
#11157=ORIENTED_EDGE('',*,*,#8314,.F.);
#11158=ORIENTED_EDGE('',*,*,#8315,.F.);
#11159=ORIENTED_EDGE('',*,*,#8316,.F.);
#11160=ORIENTED_EDGE('',*,*,#8317,.F.);
#11161=ORIENTED_EDGE('',*,*,#8318,.F.);
#11162=ORIENTED_EDGE('',*,*,#8319,.F.);
#11163=ORIENTED_EDGE('',*,*,#8320,.F.);
#11164=ORIENTED_EDGE('',*,*,#8321,.F.);
#11165=ORIENTED_EDGE('',*,*,#8322,.F.);
#11166=ORIENTED_EDGE('',*,*,#8323,.F.);
#11167=ORIENTED_EDGE('',*,*,#8324,.F.);
#11168=ORIENTED_EDGE('',*,*,#8325,.F.);
#11169=ORIENTED_EDGE('',*,*,#8326,.T.);
#11170=ORIENTED_EDGE('',*,*,#8327,.F.);
#11171=ORIENTED_EDGE('',*,*,#8328,.F.);
#11172=ORIENTED_EDGE('',*,*,#8329,.F.);
#11173=ORIENTED_EDGE('',*,*,#8330,.T.);
#11174=ORIENTED_EDGE('',*,*,#8331,.F.);
#11175=ORIENTED_EDGE('',*,*,#8332,.F.);
#11176=ORIENTED_EDGE('',*,*,#8333,.F.);
#11177=ORIENTED_EDGE('',*,*,#8334,.F.);
#11178=ORIENTED_EDGE('',*,*,#8335,.F.);
#11179=ORIENTED_EDGE('',*,*,#8336,.F.);
#11180=ORIENTED_EDGE('',*,*,#8337,.F.);
#11181=ORIENTED_EDGE('',*,*,#8338,.F.);
#11182=ORIENTED_EDGE('',*,*,#8339,.F.);
#11183=ORIENTED_EDGE('',*,*,#8340,.F.);
#11184=ORIENTED_EDGE('',*,*,#8341,.F.);
#11185=ORIENTED_EDGE('',*,*,#8342,.F.);
#11186=ORIENTED_EDGE('',*,*,#8343,.F.);
#11187=ORIENTED_EDGE('',*,*,#8344,.F.);
#11188=ORIENTED_EDGE('',*,*,#8345,.F.);
#11189=ORIENTED_EDGE('',*,*,#8346,.T.);
#11190=ORIENTED_EDGE('',*,*,#8347,.F.);
#11191=ORIENTED_EDGE('',*,*,#8348,.F.);
#11192=ORIENTED_EDGE('',*,*,#8349,.F.);
#11193=ORIENTED_EDGE('',*,*,#8350,.F.);
#11194=ORIENTED_EDGE('',*,*,#8351,.F.);
#11195=ORIENTED_EDGE('',*,*,#8352,.T.);
#11196=ORIENTED_EDGE('',*,*,#8353,.F.);
#11197=ORIENTED_EDGE('',*,*,#8354,.F.);
#11198=ORIENTED_EDGE('',*,*,#8355,.F.);
#11199=ORIENTED_EDGE('',*,*,#8356,.F.);
#11200=ORIENTED_EDGE('',*,*,#8357,.F.);
#11201=ORIENTED_EDGE('',*,*,#8358,.F.);
#11202=ORIENTED_EDGE('',*,*,#8359,.F.);
#11203=ORIENTED_EDGE('',*,*,#8360,.F.);
#11204=ORIENTED_EDGE('',*,*,#8361,.F.);
#11205=ORIENTED_EDGE('',*,*,#8362,.F.);
#11206=ORIENTED_EDGE('',*,*,#8363,.F.);
#11207=ORIENTED_EDGE('',*,*,#8364,.F.);
#11208=ORIENTED_EDGE('',*,*,#8365,.F.);
#11209=ORIENTED_EDGE('',*,*,#8366,.T.);
#11210=ORIENTED_EDGE('',*,*,#8367,.F.);
#11211=ORIENTED_EDGE('',*,*,#8368,.F.);
#11212=ORIENTED_EDGE('',*,*,#8369,.F.);
#11213=ORIENTED_EDGE('',*,*,#8370,.F.);
#11214=ORIENTED_EDGE('',*,*,#8371,.F.);
#11215=ORIENTED_EDGE('',*,*,#8372,.F.);
#11216=ORIENTED_EDGE('',*,*,#8373,.F.);
#11217=ORIENTED_EDGE('',*,*,#8374,.T.);
#11218=ORIENTED_EDGE('',*,*,#8375,.F.);
#11219=ORIENTED_EDGE('',*,*,#8376,.F.);
#11220=ORIENTED_EDGE('',*,*,#8377,.F.);
#11221=ORIENTED_EDGE('',*,*,#8378,.F.);
#11222=ORIENTED_EDGE('',*,*,#8379,.F.);
#11223=ORIENTED_EDGE('',*,*,#8380,.F.);
#11224=ORIENTED_EDGE('',*,*,#8381,.F.);
#11225=ORIENTED_EDGE('',*,*,#8382,.F.);
#11226=ORIENTED_EDGE('',*,*,#8383,.F.);
#11227=ORIENTED_EDGE('',*,*,#8384,.F.);
#11228=ORIENTED_EDGE('',*,*,#8385,.F.);
#11229=ORIENTED_EDGE('',*,*,#8386,.T.);
#11230=ORIENTED_EDGE('',*,*,#8387,.F.);
#11231=ORIENTED_EDGE('',*,*,#8388,.F.);
#11232=ORIENTED_EDGE('',*,*,#8389,.F.);
#11233=ORIENTED_EDGE('',*,*,#8390,.F.);
#11234=ORIENTED_EDGE('',*,*,#8391,.F.);
#11235=ORIENTED_EDGE('',*,*,#8392,.F.);
#11236=ORIENTED_EDGE('',*,*,#8393,.F.);
#11237=ORIENTED_EDGE('',*,*,#8394,.F.);
#11238=ORIENTED_EDGE('',*,*,#8395,.F.);
#11239=ORIENTED_EDGE('',*,*,#8396,.T.);
#11240=ORIENTED_EDGE('',*,*,#8397,.F.);
#11241=ORIENTED_EDGE('',*,*,#8398,.F.);
#11242=ORIENTED_EDGE('',*,*,#8399,.F.);
#11243=ORIENTED_EDGE('',*,*,#8400,.F.);
#11244=ORIENTED_EDGE('',*,*,#8401,.F.);
#11245=ORIENTED_EDGE('',*,*,#8402,.F.);
#11246=ORIENTED_EDGE('',*,*,#8403,.F.);
#11247=ORIENTED_EDGE('',*,*,#8404,.F.);
#11248=ORIENTED_EDGE('',*,*,#8405,.F.);
#11249=ORIENTED_EDGE('',*,*,#8406,.T.);
#11250=ORIENTED_EDGE('',*,*,#8407,.F.);
#11251=ORIENTED_EDGE('',*,*,#8408,.F.);
#11252=ORIENTED_EDGE('',*,*,#8409,.F.);
#11253=ORIENTED_EDGE('',*,*,#8410,.F.);
#11254=ORIENTED_EDGE('',*,*,#8411,.F.);
#11255=ORIENTED_EDGE('',*,*,#8412,.F.);
#11256=ORIENTED_EDGE('',*,*,#8413,.F.);
#11257=ORIENTED_EDGE('',*,*,#8414,.F.);
#11258=ORIENTED_EDGE('',*,*,#8415,.F.);
#11259=ORIENTED_EDGE('',*,*,#8416,.F.);
#11260=ORIENTED_EDGE('',*,*,#8417,.F.);
#11261=ORIENTED_EDGE('',*,*,#8418,.T.);
#11262=ORIENTED_EDGE('',*,*,#8419,.F.);
#11263=ORIENTED_EDGE('',*,*,#8420,.F.);
#11264=ORIENTED_EDGE('',*,*,#8421,.F.);
#11265=ORIENTED_EDGE('',*,*,#8422,.F.);
#11266=ORIENTED_EDGE('',*,*,#8423,.F.);
#11267=ORIENTED_EDGE('',*,*,#8424,.F.);
#11268=ORIENTED_EDGE('',*,*,#8425,.F.);
#11269=ORIENTED_EDGE('',*,*,#8067,.T.);
#11270=ORIENTED_EDGE('',*,*,#8426,.F.);
#11271=ORIENTED_EDGE('',*,*,#8265,.T.);
#11272=ORIENTED_EDGE('',*,*,#8427,.F.);
#11273=ORIENTED_EDGE('',*,*,#8428,.T.);
#11274=ORIENTED_EDGE('',*,*,#8429,.F.);
#11275=ORIENTED_EDGE('',*,*,#8430,.F.);
#11276=ORIENTED_EDGE('',*,*,#8267,.F.);
#11277=ORIENTED_EDGE('',*,*,#8264,.F.);
#11278=ORIENTED_EDGE('',*,*,#8431,.T.);
#11279=ORIENTED_EDGE('',*,*,#8432,.T.);
#11280=ORIENTED_EDGE('',*,*,#8427,.T.);
#11281=ORIENTED_EDGE('',*,*,#8433,.T.);
#11282=ORIENTED_EDGE('',*,*,#8434,.T.);
#11283=ORIENTED_EDGE('',*,*,#8435,.T.);
#11284=ORIENTED_EDGE('',*,*,#8436,.T.);
#11285=ORIENTED_EDGE('',*,*,#8437,.T.);
#11286=ORIENTED_EDGE('',*,*,#8437,.F.);
#11287=ORIENTED_EDGE('',*,*,#8438,.T.);
#11288=ORIENTED_EDGE('',*,*,#8439,.F.);
#11289=ORIENTED_EDGE('',*,*,#8440,.T.);
#11290=ORIENTED_EDGE('',*,*,#8420,.T.);
#11291=ORIENTED_EDGE('',*,*,#8441,.F.);
#11292=ORIENTED_EDGE('',*,*,#8436,.F.);
#11293=ORIENTED_EDGE('',*,*,#8442,.T.);
#11294=ORIENTED_EDGE('',*,*,#8443,.F.);
#11295=ORIENTED_EDGE('',*,*,#8438,.F.);
#11296=ORIENTED_EDGE('',*,*,#8444,.F.);
#11297=ORIENTED_EDGE('',*,*,#8445,.T.);
#11298=ORIENTED_EDGE('',*,*,#8446,.T.);
#11299=ORIENTED_EDGE('',*,*,#8439,.T.);
#11300=ORIENTED_EDGE('',*,*,#8443,.T.);
#11301=ORIENTED_EDGE('',*,*,#8447,.T.);
#11302=ORIENTED_EDGE('',*,*,#8448,.T.);
#11303=ORIENTED_EDGE('',*,*,#8449,.T.);
#11304=ORIENTED_EDGE('',*,*,#8450,.T.);
#11305=ORIENTED_EDGE('',*,*,#8451,.T.);
#11306=ORIENTED_EDGE('',*,*,#8451,.F.);
#11307=ORIENTED_EDGE('',*,*,#8452,.T.);
#11308=ORIENTED_EDGE('',*,*,#8453,.F.);
#11309=ORIENTED_EDGE('',*,*,#8454,.T.);
#11310=ORIENTED_EDGE('',*,*,#8422,.T.);
#11311=ORIENTED_EDGE('',*,*,#8455,.F.);
#11312=ORIENTED_EDGE('',*,*,#8450,.F.);
#11313=ORIENTED_EDGE('',*,*,#8456,.T.);
#11314=ORIENTED_EDGE('',*,*,#8457,.F.);
#11315=ORIENTED_EDGE('',*,*,#8452,.F.);
#11316=ORIENTED_EDGE('',*,*,#8458,.F.);
#11317=ORIENTED_EDGE('',*,*,#8459,.T.);
#11318=ORIENTED_EDGE('',*,*,#8460,.T.);
#11319=ORIENTED_EDGE('',*,*,#8453,.T.);
#11320=ORIENTED_EDGE('',*,*,#8457,.T.);
#11321=ORIENTED_EDGE('',*,*,#8461,.T.);
#11322=ORIENTED_EDGE('',*,*,#8462,.T.);
#11323=ORIENTED_EDGE('',*,*,#8463,.T.);
#11324=ORIENTED_EDGE('',*,*,#8464,.T.);
#11325=ORIENTED_EDGE('',*,*,#8465,.T.);
#11326=ORIENTED_EDGE('',*,*,#8465,.F.);
#11327=ORIENTED_EDGE('',*,*,#8466,.T.);
#11328=ORIENTED_EDGE('',*,*,#8467,.F.);
#11329=ORIENTED_EDGE('',*,*,#8468,.T.);
#11330=ORIENTED_EDGE('',*,*,#8424,.T.);
#11331=ORIENTED_EDGE('',*,*,#8469,.F.);
#11332=ORIENTED_EDGE('',*,*,#8464,.F.);
#11333=ORIENTED_EDGE('',*,*,#8470,.T.);
#11334=ORIENTED_EDGE('',*,*,#8471,.F.);
#11335=ORIENTED_EDGE('',*,*,#8466,.F.);
#11336=ORIENTED_EDGE('',*,*,#8472,.T.);
#11337=ORIENTED_EDGE('',*,*,#8473,.T.);
#11338=ORIENTED_EDGE('',*,*,#8474,.T.);
#11339=ORIENTED_EDGE('',*,*,#8069,.T.);
#11340=ORIENTED_EDGE('',*,*,#8473,.F.);
#11341=ORIENTED_EDGE('',*,*,#8475,.F.);
#11342=ORIENTED_EDGE('',*,*,#8476,.F.);
#11343=ORIENTED_EDGE('',*,*,#8477,.F.);
#11344=ORIENTED_EDGE('',*,*,#8472,.F.);
#11345=ORIENTED_EDGE('',*,*,#8068,.F.);
#11346=ORIENTED_EDGE('',*,*,#8425,.T.);
#11347=ORIENTED_EDGE('',*,*,#8468,.F.);
#11348=ORIENTED_EDGE('',*,*,#8478,.F.);
#11349=ORIENTED_EDGE('',*,*,#8475,.T.);
#11350=ORIENTED_EDGE('',*,*,#8479,.F.);
#11351=ORIENTED_EDGE('',*,*,#8476,.T.);
#11352=ORIENTED_EDGE('',*,*,#8478,.T.);
#11353=ORIENTED_EDGE('',*,*,#8467,.T.);
#11354=ORIENTED_EDGE('',*,*,#8471,.T.);
#11355=ORIENTED_EDGE('',*,*,#8480,.F.);
#11356=ORIENTED_EDGE('',*,*,#8481,.T.);
#11357=ORIENTED_EDGE('',*,*,#8482,.T.);
#11358=ORIENTED_EDGE('',*,*,#8483,.T.);
#11359=ORIENTED_EDGE('',*,*,#8482,.F.);
#11360=ORIENTED_EDGE('',*,*,#8484,.T.);
#11361=ORIENTED_EDGE('',*,*,#8485,.F.);
#11362=ORIENTED_EDGE('',*,*,#8486,.T.);
#11363=ORIENTED_EDGE('',*,*,#8407,.T.);
#11364=ORIENTED_EDGE('',*,*,#8487,.F.);
#11365=ORIENTED_EDGE('',*,*,#8481,.F.);
#11366=ORIENTED_EDGE('',*,*,#8488,.F.);
#11367=ORIENTED_EDGE('',*,*,#8489,.F.);
#11368=ORIENTED_EDGE('',*,*,#8484,.F.);
#11369=ORIENTED_EDGE('',*,*,#8485,.T.);
#11370=ORIENTED_EDGE('',*,*,#8489,.T.);
#11371=ORIENTED_EDGE('',*,*,#8490,.T.);
#11372=ORIENTED_EDGE('',*,*,#8491,.T.);
#11373=ORIENTED_EDGE('',*,*,#8492,.T.);
#11374=ORIENTED_EDGE('',*,*,#8493,.F.);
#11375=ORIENTED_EDGE('',*,*,#8494,.T.);
#11376=ORIENTED_EDGE('',*,*,#8495,.T.);
#11377=ORIENTED_EDGE('',*,*,#8496,.T.);
#11378=ORIENTED_EDGE('',*,*,#8497,.T.);
#11379=ORIENTED_EDGE('',*,*,#8495,.F.);
#11380=ORIENTED_EDGE('',*,*,#8498,.T.);
#11381=ORIENTED_EDGE('',*,*,#8499,.F.);
#11382=ORIENTED_EDGE('',*,*,#8500,.T.);
#11383=ORIENTED_EDGE('',*,*,#8409,.T.);
#11384=ORIENTED_EDGE('',*,*,#8501,.F.);
#11385=ORIENTED_EDGE('',*,*,#8494,.F.);
#11386=ORIENTED_EDGE('',*,*,#8502,.F.);
#11387=ORIENTED_EDGE('',*,*,#8503,.F.);
#11388=ORIENTED_EDGE('',*,*,#8498,.F.);
#11389=ORIENTED_EDGE('',*,*,#8499,.T.);
#11390=ORIENTED_EDGE('',*,*,#8503,.T.);
#11391=ORIENTED_EDGE('',*,*,#8504,.T.);
#11392=ORIENTED_EDGE('',*,*,#8505,.T.);
#11393=ORIENTED_EDGE('',*,*,#8506,.T.);
#11394=ORIENTED_EDGE('',*,*,#8507,.F.);
#11395=ORIENTED_EDGE('',*,*,#8508,.T.);
#11396=ORIENTED_EDGE('',*,*,#8509,.T.);
#11397=ORIENTED_EDGE('',*,*,#8510,.T.);
#11398=ORIENTED_EDGE('',*,*,#8511,.T.);
#11399=ORIENTED_EDGE('',*,*,#8509,.F.);
#11400=ORIENTED_EDGE('',*,*,#8512,.T.);
#11401=ORIENTED_EDGE('',*,*,#8513,.F.);
#11402=ORIENTED_EDGE('',*,*,#8514,.T.);
#11403=ORIENTED_EDGE('',*,*,#8411,.T.);
#11404=ORIENTED_EDGE('',*,*,#8515,.F.);
#11405=ORIENTED_EDGE('',*,*,#8508,.F.);
#11406=ORIENTED_EDGE('',*,*,#8516,.F.);
#11407=ORIENTED_EDGE('',*,*,#8517,.F.);
#11408=ORIENTED_EDGE('',*,*,#8512,.F.);
#11409=ORIENTED_EDGE('',*,*,#8513,.T.);
#11410=ORIENTED_EDGE('',*,*,#8517,.T.);
#11411=ORIENTED_EDGE('',*,*,#8518,.T.);
#11412=ORIENTED_EDGE('',*,*,#8519,.T.);
#11413=ORIENTED_EDGE('',*,*,#8520,.T.);
#11414=ORIENTED_EDGE('',*,*,#8521,.F.);
#11415=ORIENTED_EDGE('',*,*,#8522,.T.);
#11416=ORIENTED_EDGE('',*,*,#8523,.T.);
#11417=ORIENTED_EDGE('',*,*,#8524,.T.);
#11418=ORIENTED_EDGE('',*,*,#8525,.T.);
#11419=ORIENTED_EDGE('',*,*,#8523,.F.);
#11420=ORIENTED_EDGE('',*,*,#8526,.T.);
#11421=ORIENTED_EDGE('',*,*,#8527,.F.);
#11422=ORIENTED_EDGE('',*,*,#8528,.T.);
#11423=ORIENTED_EDGE('',*,*,#8413,.T.);
#11424=ORIENTED_EDGE('',*,*,#8529,.F.);
#11425=ORIENTED_EDGE('',*,*,#8522,.F.);
#11426=ORIENTED_EDGE('',*,*,#8530,.F.);
#11427=ORIENTED_EDGE('',*,*,#8531,.F.);
#11428=ORIENTED_EDGE('',*,*,#8526,.F.);
#11429=ORIENTED_EDGE('',*,*,#8527,.T.);
#11430=ORIENTED_EDGE('',*,*,#8531,.T.);
#11431=ORIENTED_EDGE('',*,*,#8532,.T.);
#11432=ORIENTED_EDGE('',*,*,#8533,.T.);
#11433=ORIENTED_EDGE('',*,*,#8534,.T.);
#11434=ORIENTED_EDGE('',*,*,#8535,.F.);
#11435=ORIENTED_EDGE('',*,*,#8536,.T.);
#11436=ORIENTED_EDGE('',*,*,#8537,.T.);
#11437=ORIENTED_EDGE('',*,*,#8538,.T.);
#11438=ORIENTED_EDGE('',*,*,#8539,.T.);
#11439=ORIENTED_EDGE('',*,*,#8537,.F.);
#11440=ORIENTED_EDGE('',*,*,#8540,.T.);
#11441=ORIENTED_EDGE('',*,*,#8541,.F.);
#11442=ORIENTED_EDGE('',*,*,#8542,.T.);
#11443=ORIENTED_EDGE('',*,*,#8415,.T.);
#11444=ORIENTED_EDGE('',*,*,#8543,.F.);
#11445=ORIENTED_EDGE('',*,*,#8536,.F.);
#11446=ORIENTED_EDGE('',*,*,#8544,.F.);
#11447=ORIENTED_EDGE('',*,*,#8545,.F.);
#11448=ORIENTED_EDGE('',*,*,#8540,.F.);
#11449=ORIENTED_EDGE('',*,*,#8541,.T.);
#11450=ORIENTED_EDGE('',*,*,#8545,.T.);
#11451=ORIENTED_EDGE('',*,*,#8546,.T.);
#11452=ORIENTED_EDGE('',*,*,#8547,.T.);
#11453=ORIENTED_EDGE('',*,*,#8548,.T.);
#11454=ORIENTED_EDGE('',*,*,#8549,.F.);
#11455=ORIENTED_EDGE('',*,*,#8550,.T.);
#11456=ORIENTED_EDGE('',*,*,#8551,.T.);
#11457=ORIENTED_EDGE('',*,*,#8552,.T.);
#11458=ORIENTED_EDGE('',*,*,#8553,.T.);
#11459=ORIENTED_EDGE('',*,*,#8551,.F.);
#11460=ORIENTED_EDGE('',*,*,#8554,.T.);
#11461=ORIENTED_EDGE('',*,*,#8555,.F.);
#11462=ORIENTED_EDGE('',*,*,#8556,.F.);
#11463=ORIENTED_EDGE('',*,*,#8417,.T.);
#11464=ORIENTED_EDGE('',*,*,#8557,.F.);
#11465=ORIENTED_EDGE('',*,*,#8550,.F.);
#11466=ORIENTED_EDGE('',*,*,#8558,.F.);
#11467=ORIENTED_EDGE('',*,*,#8559,.F.);
#11468=ORIENTED_EDGE('',*,*,#8554,.F.);
#11469=ORIENTED_EDGE('',*,*,#8560,.T.);
#11470=ORIENTED_EDGE('',*,*,#8561,.F.);
#11471=ORIENTED_EDGE('',*,*,#8562,.T.);
#11472=ORIENTED_EDGE('',*,*,#8563,.T.);
#11473=ORIENTED_EDGE('',*,*,#8433,.F.);
#11474=ORIENTED_EDGE('',*,*,#8441,.T.);
#11475=ORIENTED_EDGE('',*,*,#8419,.T.);
#11476=ORIENTED_EDGE('',*,*,#8564,.T.);
#11477=ORIENTED_EDGE('',*,*,#8563,.F.);
#11478=ORIENTED_EDGE('',*,*,#8565,.T.);
#11479=ORIENTED_EDGE('',*,*,#8446,.F.);
#11480=ORIENTED_EDGE('',*,*,#8566,.T.);
#11481=ORIENTED_EDGE('',*,*,#8447,.F.);
#11482=ORIENTED_EDGE('',*,*,#8455,.T.);
#11483=ORIENTED_EDGE('',*,*,#8421,.T.);
#11484=ORIENTED_EDGE('',*,*,#8440,.F.);
#11485=ORIENTED_EDGE('',*,*,#8460,.F.);
#11486=ORIENTED_EDGE('',*,*,#8567,.T.);
#11487=ORIENTED_EDGE('',*,*,#8461,.F.);
#11488=ORIENTED_EDGE('',*,*,#8469,.T.);
#11489=ORIENTED_EDGE('',*,*,#8423,.T.);
#11490=ORIENTED_EDGE('',*,*,#8454,.F.);
#11491=ORIENTED_EDGE('',*,*,#8459,.F.);
#11492=ORIENTED_EDGE('',*,*,#8568,.F.);
#11493=ORIENTED_EDGE('',*,*,#8462,.F.);
#11494=ORIENTED_EDGE('',*,*,#8567,.F.);
#11495=ORIENTED_EDGE('',*,*,#8445,.F.);
#11496=ORIENTED_EDGE('',*,*,#8569,.F.);
#11497=ORIENTED_EDGE('',*,*,#8448,.F.);
#11498=ORIENTED_EDGE('',*,*,#8566,.F.);
#11499=ORIENTED_EDGE('',*,*,#8434,.F.);
#11500=ORIENTED_EDGE('',*,*,#8565,.F.);
#11501=ORIENTED_EDGE('',*,*,#8562,.F.);
#11502=ORIENTED_EDGE('',*,*,#8570,.F.);
#11503=ORIENTED_EDGE('',*,*,#8555,.T.);
#11504=ORIENTED_EDGE('',*,*,#8559,.T.);
#11505=ORIENTED_EDGE('',*,*,#8571,.T.);
#11506=ORIENTED_EDGE('',*,*,#8572,.T.);
#11507=ORIENTED_EDGE('',*,*,#8492,.F.);
#11508=ORIENTED_EDGE('',*,*,#8573,.T.);
#11509=ORIENTED_EDGE('',*,*,#8496,.F.);
#11510=ORIENTED_EDGE('',*,*,#8501,.T.);
#11511=ORIENTED_EDGE('',*,*,#8408,.T.);
#11512=ORIENTED_EDGE('',*,*,#8486,.F.);
#11513=ORIENTED_EDGE('',*,*,#8506,.F.);
#11514=ORIENTED_EDGE('',*,*,#8574,.T.);
#11515=ORIENTED_EDGE('',*,*,#8510,.F.);
#11516=ORIENTED_EDGE('',*,*,#8515,.T.);
#11517=ORIENTED_EDGE('',*,*,#8410,.T.);
#11518=ORIENTED_EDGE('',*,*,#8500,.F.);
#11519=ORIENTED_EDGE('',*,*,#8520,.F.);
#11520=ORIENTED_EDGE('',*,*,#8575,.T.);
#11521=ORIENTED_EDGE('',*,*,#8524,.F.);
#11522=ORIENTED_EDGE('',*,*,#8529,.T.);
#11523=ORIENTED_EDGE('',*,*,#8412,.T.);
#11524=ORIENTED_EDGE('',*,*,#8514,.F.);
#11525=ORIENTED_EDGE('',*,*,#8534,.F.);
#11526=ORIENTED_EDGE('',*,*,#8576,.T.);
#11527=ORIENTED_EDGE('',*,*,#8538,.F.);
#11528=ORIENTED_EDGE('',*,*,#8543,.T.);
#11529=ORIENTED_EDGE('',*,*,#8414,.T.);
#11530=ORIENTED_EDGE('',*,*,#8528,.F.);
#11531=ORIENTED_EDGE('',*,*,#8548,.F.);
#11532=ORIENTED_EDGE('',*,*,#8577,.T.);
#11533=ORIENTED_EDGE('',*,*,#8552,.F.);
#11534=ORIENTED_EDGE('',*,*,#8557,.T.);
#11535=ORIENTED_EDGE('',*,*,#8416,.T.);
#11536=ORIENTED_EDGE('',*,*,#8542,.F.);
#11537=ORIENTED_EDGE('',*,*,#8564,.F.);
#11538=ORIENTED_EDGE('',*,*,#8418,.F.);
#11539=ORIENTED_EDGE('',*,*,#8556,.T.);
#11540=ORIENTED_EDGE('',*,*,#8572,.F.);
#11541=ORIENTED_EDGE('',*,*,#8578,.T.);
#11542=ORIENTED_EDGE('',*,*,#8560,.F.);
#11543=ORIENTED_EDGE('',*,*,#8547,.F.);
#11544=ORIENTED_EDGE('',*,*,#8579,.T.);
#11545=ORIENTED_EDGE('',*,*,#8553,.F.);
#11546=ORIENTED_EDGE('',*,*,#8577,.F.);
#11547=ORIENTED_EDGE('',*,*,#8533,.F.);
#11548=ORIENTED_EDGE('',*,*,#8580,.T.);
#11549=ORIENTED_EDGE('',*,*,#8539,.F.);
#11550=ORIENTED_EDGE('',*,*,#8576,.F.);
#11551=ORIENTED_EDGE('',*,*,#8519,.F.);
#11552=ORIENTED_EDGE('',*,*,#8581,.T.);
#11553=ORIENTED_EDGE('',*,*,#8525,.F.);
#11554=ORIENTED_EDGE('',*,*,#8575,.F.);
#11555=ORIENTED_EDGE('',*,*,#8505,.F.);
#11556=ORIENTED_EDGE('',*,*,#8582,.T.);
#11557=ORIENTED_EDGE('',*,*,#8511,.F.);
#11558=ORIENTED_EDGE('',*,*,#8574,.F.);
#11559=ORIENTED_EDGE('',*,*,#8491,.F.);
#11560=ORIENTED_EDGE('',*,*,#8583,.T.);
#11561=ORIENTED_EDGE('',*,*,#8497,.F.);
#11562=ORIENTED_EDGE('',*,*,#8573,.F.);
#11563=ORIENTED_EDGE('',*,*,#8584,.T.);
#11564=ORIENTED_EDGE('',*,*,#8585,.T.);
#11565=ORIENTED_EDGE('',*,*,#8586,.T.);
#11566=ORIENTED_EDGE('',*,*,#8587,.T.);
#11567=ORIENTED_EDGE('',*,*,#8588,.T.);
#11568=ORIENTED_EDGE('',*,*,#8588,.F.);
#11569=ORIENTED_EDGE('',*,*,#8589,.T.);
#11570=ORIENTED_EDGE('',*,*,#8590,.F.);
#11571=ORIENTED_EDGE('',*,*,#8591,.F.);
#11572=ORIENTED_EDGE('',*,*,#8398,.T.);
#11573=ORIENTED_EDGE('',*,*,#8592,.F.);
#11574=ORIENTED_EDGE('',*,*,#8587,.F.);
#11575=ORIENTED_EDGE('',*,*,#8593,.T.);
#11576=ORIENTED_EDGE('',*,*,#8594,.F.);
#11577=ORIENTED_EDGE('',*,*,#8589,.F.);
#11578=ORIENTED_EDGE('',*,*,#8595,.F.);
#11579=ORIENTED_EDGE('',*,*,#8596,.T.);
#11580=ORIENTED_EDGE('',*,*,#8597,.T.);
#11581=ORIENTED_EDGE('',*,*,#8590,.T.);
#11582=ORIENTED_EDGE('',*,*,#8594,.T.);
#11583=ORIENTED_EDGE('',*,*,#8597,.F.);
#11584=ORIENTED_EDGE('',*,*,#8598,.T.);
#11585=ORIENTED_EDGE('',*,*,#8599,.F.);
#11586=ORIENTED_EDGE('',*,*,#8600,.T.);
#11587=ORIENTED_EDGE('',*,*,#8399,.T.);
#11588=ORIENTED_EDGE('',*,*,#8591,.T.);
#11589=ORIENTED_EDGE('',*,*,#8599,.T.);
#11590=ORIENTED_EDGE('',*,*,#8601,.T.);
#11591=ORIENTED_EDGE('',*,*,#8602,.T.);
#11592=ORIENTED_EDGE('',*,*,#8603,.T.);
#11593=ORIENTED_EDGE('',*,*,#8604,.T.);
#11594=ORIENTED_EDGE('',*,*,#8604,.F.);
#11595=ORIENTED_EDGE('',*,*,#8605,.T.);
#11596=ORIENTED_EDGE('',*,*,#8606,.F.);
#11597=ORIENTED_EDGE('',*,*,#8607,.T.);
#11598=ORIENTED_EDGE('',*,*,#8400,.T.);
#11599=ORIENTED_EDGE('',*,*,#8600,.F.);
#11600=ORIENTED_EDGE('',*,*,#8603,.F.);
#11601=ORIENTED_EDGE('',*,*,#8608,.T.);
#11602=ORIENTED_EDGE('',*,*,#8609,.F.);
#11603=ORIENTED_EDGE('',*,*,#8605,.F.);
#11604=ORIENTED_EDGE('',*,*,#8610,.F.);
#11605=ORIENTED_EDGE('',*,*,#8611,.T.);
#11606=ORIENTED_EDGE('',*,*,#8612,.T.);
#11607=ORIENTED_EDGE('',*,*,#8606,.T.);
#11608=ORIENTED_EDGE('',*,*,#8609,.T.);
#11609=ORIENTED_EDGE('',*,*,#8613,.T.);
#11610=ORIENTED_EDGE('',*,*,#8614,.T.);
#11611=ORIENTED_EDGE('',*,*,#8615,.T.);
#11612=ORIENTED_EDGE('',*,*,#8616,.T.);
#11613=ORIENTED_EDGE('',*,*,#8617,.T.);
#11614=ORIENTED_EDGE('',*,*,#8617,.F.);
#11615=ORIENTED_EDGE('',*,*,#8618,.T.);
#11616=ORIENTED_EDGE('',*,*,#8619,.F.);
#11617=ORIENTED_EDGE('',*,*,#8620,.T.);
#11618=ORIENTED_EDGE('',*,*,#8402,.T.);
#11619=ORIENTED_EDGE('',*,*,#8621,.F.);
#11620=ORIENTED_EDGE('',*,*,#8616,.F.);
#11621=ORIENTED_EDGE('',*,*,#8622,.T.);
#11622=ORIENTED_EDGE('',*,*,#8623,.F.);
#11623=ORIENTED_EDGE('',*,*,#8618,.F.);
#11624=ORIENTED_EDGE('',*,*,#8624,.F.);
#11625=ORIENTED_EDGE('',*,*,#8625,.T.);
#11626=ORIENTED_EDGE('',*,*,#8626,.T.);
#11627=ORIENTED_EDGE('',*,*,#8619,.T.);
#11628=ORIENTED_EDGE('',*,*,#8623,.T.);
#11629=ORIENTED_EDGE('',*,*,#8627,.T.);
#11630=ORIENTED_EDGE('',*,*,#8628,.T.);
#11631=ORIENTED_EDGE('',*,*,#8629,.T.);
#11632=ORIENTED_EDGE('',*,*,#8630,.T.);
#11633=ORIENTED_EDGE('',*,*,#8631,.T.);
#11634=ORIENTED_EDGE('',*,*,#8631,.F.);
#11635=ORIENTED_EDGE('',*,*,#8632,.T.);
#11636=ORIENTED_EDGE('',*,*,#8633,.F.);
#11637=ORIENTED_EDGE('',*,*,#8634,.T.);
#11638=ORIENTED_EDGE('',*,*,#8404,.T.);
#11639=ORIENTED_EDGE('',*,*,#8635,.F.);
#11640=ORIENTED_EDGE('',*,*,#8630,.F.);
#11641=ORIENTED_EDGE('',*,*,#8636,.T.);
#11642=ORIENTED_EDGE('',*,*,#8637,.F.);
#11643=ORIENTED_EDGE('',*,*,#8632,.F.);
#11644=ORIENTED_EDGE('',*,*,#8638,.T.);
#11645=ORIENTED_EDGE('',*,*,#8639,.T.);
#11646=ORIENTED_EDGE('',*,*,#8640,.T.);
#11647=ORIENTED_EDGE('',*,*,#8641,.T.);
#11648=ORIENTED_EDGE('',*,*,#8639,.F.);
#11649=ORIENTED_EDGE('',*,*,#8642,.F.);
#11650=ORIENTED_EDGE('',*,*,#8643,.F.);
#11651=ORIENTED_EDGE('',*,*,#8644,.F.);
#11652=ORIENTED_EDGE('',*,*,#8638,.F.);
#11653=ORIENTED_EDGE('',*,*,#8645,.F.);
#11654=ORIENTED_EDGE('',*,*,#8405,.T.);
#11655=ORIENTED_EDGE('',*,*,#8634,.F.);
#11656=ORIENTED_EDGE('',*,*,#8646,.F.);
#11657=ORIENTED_EDGE('',*,*,#8642,.T.);
#11658=ORIENTED_EDGE('',*,*,#8647,.F.);
#11659=ORIENTED_EDGE('',*,*,#8643,.T.);
#11660=ORIENTED_EDGE('',*,*,#8646,.T.);
#11661=ORIENTED_EDGE('',*,*,#8633,.T.);
#11662=ORIENTED_EDGE('',*,*,#8637,.T.);
#11663=ORIENTED_EDGE('',*,*,#8648,.F.);
#11664=ORIENTED_EDGE('',*,*,#8649,.T.);
#11665=ORIENTED_EDGE('',*,*,#8650,.T.);
#11666=ORIENTED_EDGE('',*,*,#8651,.T.);
#11667=ORIENTED_EDGE('',*,*,#8650,.F.);
#11668=ORIENTED_EDGE('',*,*,#8652,.T.);
#11669=ORIENTED_EDGE('',*,*,#8653,.F.);
#11670=ORIENTED_EDGE('',*,*,#8654,.T.);
#11671=ORIENTED_EDGE('',*,*,#8387,.T.);
#11672=ORIENTED_EDGE('',*,*,#8655,.F.);
#11673=ORIENTED_EDGE('',*,*,#8649,.F.);
#11674=ORIENTED_EDGE('',*,*,#8656,.F.);
#11675=ORIENTED_EDGE('',*,*,#8657,.F.);
#11676=ORIENTED_EDGE('',*,*,#8652,.F.);
#11677=ORIENTED_EDGE('',*,*,#8653,.T.);
#11678=ORIENTED_EDGE('',*,*,#8657,.T.);
#11679=ORIENTED_EDGE('',*,*,#8658,.T.);
#11680=ORIENTED_EDGE('',*,*,#8659,.T.);
#11681=ORIENTED_EDGE('',*,*,#8660,.T.);
#11682=ORIENTED_EDGE('',*,*,#8661,.F.);
#11683=ORIENTED_EDGE('',*,*,#8662,.T.);
#11684=ORIENTED_EDGE('',*,*,#8663,.T.);
#11685=ORIENTED_EDGE('',*,*,#8664,.T.);
#11686=ORIENTED_EDGE('',*,*,#8665,.T.);
#11687=ORIENTED_EDGE('',*,*,#8663,.F.);
#11688=ORIENTED_EDGE('',*,*,#8666,.T.);
#11689=ORIENTED_EDGE('',*,*,#8667,.F.);
#11690=ORIENTED_EDGE('',*,*,#8668,.T.);
#11691=ORIENTED_EDGE('',*,*,#8389,.T.);
#11692=ORIENTED_EDGE('',*,*,#8669,.F.);
#11693=ORIENTED_EDGE('',*,*,#8662,.F.);
#11694=ORIENTED_EDGE('',*,*,#8670,.F.);
#11695=ORIENTED_EDGE('',*,*,#8671,.F.);
#11696=ORIENTED_EDGE('',*,*,#8666,.F.);
#11697=ORIENTED_EDGE('',*,*,#8667,.T.);
#11698=ORIENTED_EDGE('',*,*,#8671,.T.);
#11699=ORIENTED_EDGE('',*,*,#8672,.T.);
#11700=ORIENTED_EDGE('',*,*,#8673,.T.);
#11701=ORIENTED_EDGE('',*,*,#8674,.T.);
#11702=ORIENTED_EDGE('',*,*,#8675,.F.);
#11703=ORIENTED_EDGE('',*,*,#8676,.T.);
#11704=ORIENTED_EDGE('',*,*,#8677,.T.);
#11705=ORIENTED_EDGE('',*,*,#8678,.T.);
#11706=ORIENTED_EDGE('',*,*,#8679,.T.);
#11707=ORIENTED_EDGE('',*,*,#8677,.F.);
#11708=ORIENTED_EDGE('',*,*,#8680,.T.);
#11709=ORIENTED_EDGE('',*,*,#8681,.F.);
#11710=ORIENTED_EDGE('',*,*,#8682,.T.);
#11711=ORIENTED_EDGE('',*,*,#8391,.T.);
#11712=ORIENTED_EDGE('',*,*,#8683,.F.);
#11713=ORIENTED_EDGE('',*,*,#8676,.F.);
#11714=ORIENTED_EDGE('',*,*,#8684,.F.);
#11715=ORIENTED_EDGE('',*,*,#8685,.F.);
#11716=ORIENTED_EDGE('',*,*,#8680,.F.);
#11717=ORIENTED_EDGE('',*,*,#8681,.T.);
#11718=ORIENTED_EDGE('',*,*,#8685,.T.);
#11719=ORIENTED_EDGE('',*,*,#8686,.T.);
#11720=ORIENTED_EDGE('',*,*,#8687,.T.);
#11721=ORIENTED_EDGE('',*,*,#8688,.T.);
#11722=ORIENTED_EDGE('',*,*,#8689,.F.);
#11723=ORIENTED_EDGE('',*,*,#8690,.T.);
#11724=ORIENTED_EDGE('',*,*,#8691,.T.);
#11725=ORIENTED_EDGE('',*,*,#8692,.T.);
#11726=ORIENTED_EDGE('',*,*,#8693,.T.);
#11727=ORIENTED_EDGE('',*,*,#8691,.F.);
#11728=ORIENTED_EDGE('',*,*,#8694,.T.);
#11729=ORIENTED_EDGE('',*,*,#8695,.F.);
#11730=ORIENTED_EDGE('',*,*,#8696,.T.);
#11731=ORIENTED_EDGE('',*,*,#8393,.T.);
#11732=ORIENTED_EDGE('',*,*,#8697,.F.);
#11733=ORIENTED_EDGE('',*,*,#8690,.F.);
#11734=ORIENTED_EDGE('',*,*,#8698,.F.);
#11735=ORIENTED_EDGE('',*,*,#8699,.F.);
#11736=ORIENTED_EDGE('',*,*,#8694,.F.);
#11737=ORIENTED_EDGE('',*,*,#8695,.T.);
#11738=ORIENTED_EDGE('',*,*,#8699,.T.);
#11739=ORIENTED_EDGE('',*,*,#8700,.T.);
#11740=ORIENTED_EDGE('',*,*,#8701,.T.);
#11741=ORIENTED_EDGE('',*,*,#8702,.T.);
#11742=ORIENTED_EDGE('',*,*,#8703,.F.);
#11743=ORIENTED_EDGE('',*,*,#8704,.T.);
#11744=ORIENTED_EDGE('',*,*,#8705,.T.);
#11745=ORIENTED_EDGE('',*,*,#8706,.T.);
#11746=ORIENTED_EDGE('',*,*,#8707,.T.);
#11747=ORIENTED_EDGE('',*,*,#8705,.F.);
#11748=ORIENTED_EDGE('',*,*,#8708,.T.);
#11749=ORIENTED_EDGE('',*,*,#8709,.F.);
#11750=ORIENTED_EDGE('',*,*,#8710,.F.);
#11751=ORIENTED_EDGE('',*,*,#8395,.T.);
#11752=ORIENTED_EDGE('',*,*,#8711,.T.);
#11753=ORIENTED_EDGE('',*,*,#8704,.F.);
#11754=ORIENTED_EDGE('',*,*,#8712,.F.);
#11755=ORIENTED_EDGE('',*,*,#8713,.F.);
#11756=ORIENTED_EDGE('',*,*,#8708,.F.);
#11757=ORIENTED_EDGE('',*,*,#8714,.T.);
#11758=ORIENTED_EDGE('',*,*,#8715,.F.);
#11759=ORIENTED_EDGE('',*,*,#8716,.T.);
#11760=ORIENTED_EDGE('',*,*,#8717,.T.);
#11761=ORIENTED_EDGE('',*,*,#8584,.F.);
#11762=ORIENTED_EDGE('',*,*,#8592,.T.);
#11763=ORIENTED_EDGE('',*,*,#8397,.T.);
#11764=ORIENTED_EDGE('',*,*,#8718,.T.);
#11765=ORIENTED_EDGE('',*,*,#8717,.F.);
#11766=ORIENTED_EDGE('',*,*,#8719,.T.);
#11767=ORIENTED_EDGE('',*,*,#8612,.F.);
#11768=ORIENTED_EDGE('',*,*,#8720,.T.);
#11769=ORIENTED_EDGE('',*,*,#8613,.F.);
#11770=ORIENTED_EDGE('',*,*,#8621,.T.);
#11771=ORIENTED_EDGE('',*,*,#8401,.T.);
#11772=ORIENTED_EDGE('',*,*,#8607,.F.);
#11773=ORIENTED_EDGE('',*,*,#8626,.F.);
#11774=ORIENTED_EDGE('',*,*,#8721,.T.);
#11775=ORIENTED_EDGE('',*,*,#8627,.F.);
#11776=ORIENTED_EDGE('',*,*,#8635,.T.);
#11777=ORIENTED_EDGE('',*,*,#8403,.T.);
#11778=ORIENTED_EDGE('',*,*,#8620,.F.);
#11779=ORIENTED_EDGE('',*,*,#8625,.F.);
#11780=ORIENTED_EDGE('',*,*,#8722,.F.);
#11781=ORIENTED_EDGE('',*,*,#8628,.F.);
#11782=ORIENTED_EDGE('',*,*,#8721,.F.);
#11783=ORIENTED_EDGE('',*,*,#8611,.F.);
#11784=ORIENTED_EDGE('',*,*,#8723,.F.);
#11785=ORIENTED_EDGE('',*,*,#8614,.F.);
#11786=ORIENTED_EDGE('',*,*,#8720,.F.);
#11787=ORIENTED_EDGE('',*,*,#8596,.F.);
#11788=ORIENTED_EDGE('',*,*,#8724,.F.);
#11789=ORIENTED_EDGE('',*,*,#8601,.F.);
#11790=ORIENTED_EDGE('',*,*,#8598,.F.);
#11791=ORIENTED_EDGE('',*,*,#8585,.F.);
#11792=ORIENTED_EDGE('',*,*,#8719,.F.);
#11793=ORIENTED_EDGE('',*,*,#8716,.F.);
#11794=ORIENTED_EDGE('',*,*,#8725,.F.);
#11795=ORIENTED_EDGE('',*,*,#8709,.T.);
#11796=ORIENTED_EDGE('',*,*,#8713,.T.);
#11797=ORIENTED_EDGE('',*,*,#8726,.T.);
#11798=ORIENTED_EDGE('',*,*,#8727,.T.);
#11799=ORIENTED_EDGE('',*,*,#8660,.F.);
#11800=ORIENTED_EDGE('',*,*,#8728,.T.);
#11801=ORIENTED_EDGE('',*,*,#8664,.F.);
#11802=ORIENTED_EDGE('',*,*,#8669,.T.);
#11803=ORIENTED_EDGE('',*,*,#8388,.T.);
#11804=ORIENTED_EDGE('',*,*,#8654,.F.);
#11805=ORIENTED_EDGE('',*,*,#8674,.F.);
#11806=ORIENTED_EDGE('',*,*,#8729,.T.);
#11807=ORIENTED_EDGE('',*,*,#8678,.F.);
#11808=ORIENTED_EDGE('',*,*,#8683,.T.);
#11809=ORIENTED_EDGE('',*,*,#8390,.T.);
#11810=ORIENTED_EDGE('',*,*,#8668,.F.);
#11811=ORIENTED_EDGE('',*,*,#8688,.F.);
#11812=ORIENTED_EDGE('',*,*,#8730,.T.);
#11813=ORIENTED_EDGE('',*,*,#8692,.F.);
#11814=ORIENTED_EDGE('',*,*,#8697,.T.);
#11815=ORIENTED_EDGE('',*,*,#8392,.T.);
#11816=ORIENTED_EDGE('',*,*,#8682,.F.);
#11817=ORIENTED_EDGE('',*,*,#8702,.F.);
#11818=ORIENTED_EDGE('',*,*,#8731,.T.);
#11819=ORIENTED_EDGE('',*,*,#8706,.F.);
#11820=ORIENTED_EDGE('',*,*,#8711,.F.);
#11821=ORIENTED_EDGE('',*,*,#8394,.T.);
#11822=ORIENTED_EDGE('',*,*,#8696,.F.);
#11823=ORIENTED_EDGE('',*,*,#8718,.F.);
#11824=ORIENTED_EDGE('',*,*,#8396,.F.);
#11825=ORIENTED_EDGE('',*,*,#8710,.T.);
#11826=ORIENTED_EDGE('',*,*,#8727,.F.);
#11827=ORIENTED_EDGE('',*,*,#8732,.T.);
#11828=ORIENTED_EDGE('',*,*,#8714,.F.);
#11829=ORIENTED_EDGE('',*,*,#8701,.F.);
#11830=ORIENTED_EDGE('',*,*,#8733,.T.);
#11831=ORIENTED_EDGE('',*,*,#8707,.F.);
#11832=ORIENTED_EDGE('',*,*,#8731,.F.);
#11833=ORIENTED_EDGE('',*,*,#8687,.F.);
#11834=ORIENTED_EDGE('',*,*,#8734,.T.);
#11835=ORIENTED_EDGE('',*,*,#8693,.F.);
#11836=ORIENTED_EDGE('',*,*,#8730,.F.);
#11837=ORIENTED_EDGE('',*,*,#8673,.F.);
#11838=ORIENTED_EDGE('',*,*,#8735,.T.);
#11839=ORIENTED_EDGE('',*,*,#8679,.F.);
#11840=ORIENTED_EDGE('',*,*,#8729,.F.);
#11841=ORIENTED_EDGE('',*,*,#8659,.F.);
#11842=ORIENTED_EDGE('',*,*,#8736,.T.);
#11843=ORIENTED_EDGE('',*,*,#8665,.F.);
#11844=ORIENTED_EDGE('',*,*,#8728,.F.);
#11845=ORIENTED_EDGE('',*,*,#8737,.T.);
#11846=ORIENTED_EDGE('',*,*,#8738,.T.);
#11847=ORIENTED_EDGE('',*,*,#8739,.T.);
#11848=ORIENTED_EDGE('',*,*,#8740,.T.);
#11849=ORIENTED_EDGE('',*,*,#8741,.T.);
#11850=ORIENTED_EDGE('',*,*,#8741,.F.);
#11851=ORIENTED_EDGE('',*,*,#8742,.T.);
#11852=ORIENTED_EDGE('',*,*,#8743,.F.);
#11853=ORIENTED_EDGE('',*,*,#8744,.T.);
#11854=ORIENTED_EDGE('',*,*,#8376,.T.);
#11855=ORIENTED_EDGE('',*,*,#8745,.F.);
#11856=ORIENTED_EDGE('',*,*,#8740,.F.);
#11857=ORIENTED_EDGE('',*,*,#8746,.T.);
#11858=ORIENTED_EDGE('',*,*,#8747,.F.);
#11859=ORIENTED_EDGE('',*,*,#8742,.F.);
#11860=ORIENTED_EDGE('',*,*,#8748,.F.);
#11861=ORIENTED_EDGE('',*,*,#8749,.T.);
#11862=ORIENTED_EDGE('',*,*,#8750,.T.);
#11863=ORIENTED_EDGE('',*,*,#8743,.T.);
#11864=ORIENTED_EDGE('',*,*,#8747,.T.);
#11865=ORIENTED_EDGE('',*,*,#8751,.T.);
#11866=ORIENTED_EDGE('',*,*,#8752,.T.);
#11867=ORIENTED_EDGE('',*,*,#8753,.T.);
#11868=ORIENTED_EDGE('',*,*,#8754,.T.);
#11869=ORIENTED_EDGE('',*,*,#8755,.T.);
#11870=ORIENTED_EDGE('',*,*,#8755,.F.);
#11871=ORIENTED_EDGE('',*,*,#8756,.T.);
#11872=ORIENTED_EDGE('',*,*,#8757,.F.);
#11873=ORIENTED_EDGE('',*,*,#8758,.T.);
#11874=ORIENTED_EDGE('',*,*,#8378,.T.);
#11875=ORIENTED_EDGE('',*,*,#8759,.F.);
#11876=ORIENTED_EDGE('',*,*,#8754,.F.);
#11877=ORIENTED_EDGE('',*,*,#8760,.T.);
#11878=ORIENTED_EDGE('',*,*,#8761,.F.);
#11879=ORIENTED_EDGE('',*,*,#8756,.F.);
#11880=ORIENTED_EDGE('',*,*,#8762,.F.);
#11881=ORIENTED_EDGE('',*,*,#8763,.T.);
#11882=ORIENTED_EDGE('',*,*,#8764,.T.);
#11883=ORIENTED_EDGE('',*,*,#8757,.T.);
#11884=ORIENTED_EDGE('',*,*,#8761,.T.);
#11885=ORIENTED_EDGE('',*,*,#8765,.T.);
#11886=ORIENTED_EDGE('',*,*,#8766,.T.);
#11887=ORIENTED_EDGE('',*,*,#8767,.T.);
#11888=ORIENTED_EDGE('',*,*,#8768,.T.);
#11889=ORIENTED_EDGE('',*,*,#8769,.T.);
#11890=ORIENTED_EDGE('',*,*,#8769,.F.);
#11891=ORIENTED_EDGE('',*,*,#8770,.T.);
#11892=ORIENTED_EDGE('',*,*,#8771,.F.);
#11893=ORIENTED_EDGE('',*,*,#8772,.T.);
#11894=ORIENTED_EDGE('',*,*,#8380,.T.);
#11895=ORIENTED_EDGE('',*,*,#8773,.F.);
#11896=ORIENTED_EDGE('',*,*,#8768,.F.);
#11897=ORIENTED_EDGE('',*,*,#8774,.T.);
#11898=ORIENTED_EDGE('',*,*,#8775,.F.);
#11899=ORIENTED_EDGE('',*,*,#8770,.F.);
#11900=ORIENTED_EDGE('',*,*,#8776,.F.);
#11901=ORIENTED_EDGE('',*,*,#8777,.T.);
#11902=ORIENTED_EDGE('',*,*,#8778,.T.);
#11903=ORIENTED_EDGE('',*,*,#8771,.T.);
#11904=ORIENTED_EDGE('',*,*,#8775,.T.);
#11905=ORIENTED_EDGE('',*,*,#8779,.T.);
#11906=ORIENTED_EDGE('',*,*,#8780,.T.);
#11907=ORIENTED_EDGE('',*,*,#8781,.T.);
#11908=ORIENTED_EDGE('',*,*,#8782,.T.);
#11909=ORIENTED_EDGE('',*,*,#8783,.T.);
#11910=ORIENTED_EDGE('',*,*,#8783,.F.);
#11911=ORIENTED_EDGE('',*,*,#8784,.T.);
#11912=ORIENTED_EDGE('',*,*,#8785,.F.);
#11913=ORIENTED_EDGE('',*,*,#8786,.T.);
#11914=ORIENTED_EDGE('',*,*,#8382,.T.);
#11915=ORIENTED_EDGE('',*,*,#8787,.F.);
#11916=ORIENTED_EDGE('',*,*,#8782,.F.);
#11917=ORIENTED_EDGE('',*,*,#8788,.T.);
#11918=ORIENTED_EDGE('',*,*,#8789,.F.);
#11919=ORIENTED_EDGE('',*,*,#8784,.F.);
#11920=ORIENTED_EDGE('',*,*,#8790,.F.);
#11921=ORIENTED_EDGE('',*,*,#8791,.T.);
#11922=ORIENTED_EDGE('',*,*,#8792,.T.);
#11923=ORIENTED_EDGE('',*,*,#8785,.T.);
#11924=ORIENTED_EDGE('',*,*,#8789,.T.);
#11925=ORIENTED_EDGE('',*,*,#8793,.T.);
#11926=ORIENTED_EDGE('',*,*,#8794,.T.);
#11927=ORIENTED_EDGE('',*,*,#8795,.T.);
#11928=ORIENTED_EDGE('',*,*,#8796,.T.);
#11929=ORIENTED_EDGE('',*,*,#8797,.T.);
#11930=ORIENTED_EDGE('',*,*,#8797,.F.);
#11931=ORIENTED_EDGE('',*,*,#8798,.T.);
#11932=ORIENTED_EDGE('',*,*,#8799,.F.);
#11933=ORIENTED_EDGE('',*,*,#8800,.T.);
#11934=ORIENTED_EDGE('',*,*,#8384,.T.);
#11935=ORIENTED_EDGE('',*,*,#8801,.F.);
#11936=ORIENTED_EDGE('',*,*,#8796,.F.);
#11937=ORIENTED_EDGE('',*,*,#8802,.T.);
#11938=ORIENTED_EDGE('',*,*,#8803,.F.);
#11939=ORIENTED_EDGE('',*,*,#8798,.F.);
#11940=ORIENTED_EDGE('',*,*,#8804,.T.);
#11941=ORIENTED_EDGE('',*,*,#8805,.T.);
#11942=ORIENTED_EDGE('',*,*,#8806,.T.);
#11943=ORIENTED_EDGE('',*,*,#8807,.T.);
#11944=ORIENTED_EDGE('',*,*,#8805,.F.);
#11945=ORIENTED_EDGE('',*,*,#8808,.F.);
#11946=ORIENTED_EDGE('',*,*,#8809,.F.);
#11947=ORIENTED_EDGE('',*,*,#8810,.F.);
#11948=ORIENTED_EDGE('',*,*,#8804,.F.);
#11949=ORIENTED_EDGE('',*,*,#8811,.F.);
#11950=ORIENTED_EDGE('',*,*,#8385,.T.);
#11951=ORIENTED_EDGE('',*,*,#8800,.F.);
#11952=ORIENTED_EDGE('',*,*,#8812,.F.);
#11953=ORIENTED_EDGE('',*,*,#8808,.T.);
#11954=ORIENTED_EDGE('',*,*,#8813,.F.);
#11955=ORIENTED_EDGE('',*,*,#8809,.T.);
#11956=ORIENTED_EDGE('',*,*,#8812,.T.);
#11957=ORIENTED_EDGE('',*,*,#8799,.T.);
#11958=ORIENTED_EDGE('',*,*,#8803,.T.);
#11959=ORIENTED_EDGE('',*,*,#8814,.F.);
#11960=ORIENTED_EDGE('',*,*,#8815,.T.);
#11961=ORIENTED_EDGE('',*,*,#8816,.T.);
#11962=ORIENTED_EDGE('',*,*,#8817,.T.);
#11963=ORIENTED_EDGE('',*,*,#8816,.F.);
#11964=ORIENTED_EDGE('',*,*,#8818,.T.);
#11965=ORIENTED_EDGE('',*,*,#8819,.F.);
#11966=ORIENTED_EDGE('',*,*,#8820,.T.);
#11967=ORIENTED_EDGE('',*,*,#8367,.T.);
#11968=ORIENTED_EDGE('',*,*,#8821,.F.);
#11969=ORIENTED_EDGE('',*,*,#8815,.F.);
#11970=ORIENTED_EDGE('',*,*,#8822,.F.);
#11971=ORIENTED_EDGE('',*,*,#8823,.F.);
#11972=ORIENTED_EDGE('',*,*,#8818,.F.);
#11973=ORIENTED_EDGE('',*,*,#8819,.T.);
#11974=ORIENTED_EDGE('',*,*,#8823,.T.);
#11975=ORIENTED_EDGE('',*,*,#8824,.T.);
#11976=ORIENTED_EDGE('',*,*,#8825,.T.);
#11977=ORIENTED_EDGE('',*,*,#8826,.T.);
#11978=ORIENTED_EDGE('',*,*,#8827,.F.);
#11979=ORIENTED_EDGE('',*,*,#8828,.T.);
#11980=ORIENTED_EDGE('',*,*,#8829,.T.);
#11981=ORIENTED_EDGE('',*,*,#8830,.T.);
#11982=ORIENTED_EDGE('',*,*,#8831,.T.);
#11983=ORIENTED_EDGE('',*,*,#8829,.F.);
#11984=ORIENTED_EDGE('',*,*,#8832,.T.);
#11985=ORIENTED_EDGE('',*,*,#8833,.F.);
#11986=ORIENTED_EDGE('',*,*,#8834,.T.);
#11987=ORIENTED_EDGE('',*,*,#8369,.T.);
#11988=ORIENTED_EDGE('',*,*,#8835,.F.);
#11989=ORIENTED_EDGE('',*,*,#8828,.F.);
#11990=ORIENTED_EDGE('',*,*,#8836,.F.);
#11991=ORIENTED_EDGE('',*,*,#8837,.F.);
#11992=ORIENTED_EDGE('',*,*,#8832,.F.);
#11993=ORIENTED_EDGE('',*,*,#8833,.T.);
#11994=ORIENTED_EDGE('',*,*,#8837,.T.);
#11995=ORIENTED_EDGE('',*,*,#8838,.T.);
#11996=ORIENTED_EDGE('',*,*,#8839,.T.);
#11997=ORIENTED_EDGE('',*,*,#8840,.T.);
#11998=ORIENTED_EDGE('',*,*,#8841,.F.);
#11999=ORIENTED_EDGE('',*,*,#8842,.T.);
#12000=ORIENTED_EDGE('',*,*,#8843,.T.);
#12001=ORIENTED_EDGE('',*,*,#8844,.T.);
#12002=ORIENTED_EDGE('',*,*,#8845,.T.);
#12003=ORIENTED_EDGE('',*,*,#8843,.F.);
#12004=ORIENTED_EDGE('',*,*,#8846,.T.);
#12005=ORIENTED_EDGE('',*,*,#8847,.F.);
#12006=ORIENTED_EDGE('',*,*,#8848,.T.);
#12007=ORIENTED_EDGE('',*,*,#8371,.T.);
#12008=ORIENTED_EDGE('',*,*,#8849,.F.);
#12009=ORIENTED_EDGE('',*,*,#8842,.F.);
#12010=ORIENTED_EDGE('',*,*,#8850,.F.);
#12011=ORIENTED_EDGE('',*,*,#8851,.F.);
#12012=ORIENTED_EDGE('',*,*,#8846,.F.);
#12013=ORIENTED_EDGE('',*,*,#8847,.T.);
#12014=ORIENTED_EDGE('',*,*,#8851,.T.);
#12015=ORIENTED_EDGE('',*,*,#8852,.T.);
#12016=ORIENTED_EDGE('',*,*,#8853,.T.);
#12017=ORIENTED_EDGE('',*,*,#8854,.T.);
#12018=ORIENTED_EDGE('',*,*,#8855,.F.);
#12019=ORIENTED_EDGE('',*,*,#8856,.T.);
#12020=ORIENTED_EDGE('',*,*,#8857,.T.);
#12021=ORIENTED_EDGE('',*,*,#8858,.T.);
#12022=ORIENTED_EDGE('',*,*,#8859,.T.);
#12023=ORIENTED_EDGE('',*,*,#8857,.F.);
#12024=ORIENTED_EDGE('',*,*,#8860,.T.);
#12025=ORIENTED_EDGE('',*,*,#8861,.F.);
#12026=ORIENTED_EDGE('',*,*,#8862,.F.);
#12027=ORIENTED_EDGE('',*,*,#8373,.T.);
#12028=ORIENTED_EDGE('',*,*,#8863,.F.);
#12029=ORIENTED_EDGE('',*,*,#8856,.F.);
#12030=ORIENTED_EDGE('',*,*,#8864,.F.);
#12031=ORIENTED_EDGE('',*,*,#8865,.F.);
#12032=ORIENTED_EDGE('',*,*,#8860,.F.);
#12033=ORIENTED_EDGE('',*,*,#8866,.T.);
#12034=ORIENTED_EDGE('',*,*,#8867,.F.);
#12035=ORIENTED_EDGE('',*,*,#8868,.T.);
#12036=ORIENTED_EDGE('',*,*,#8869,.T.);
#12037=ORIENTED_EDGE('',*,*,#8737,.F.);
#12038=ORIENTED_EDGE('',*,*,#8745,.T.);
#12039=ORIENTED_EDGE('',*,*,#8375,.T.);
#12040=ORIENTED_EDGE('',*,*,#8870,.T.);
#12041=ORIENTED_EDGE('',*,*,#8869,.F.);
#12042=ORIENTED_EDGE('',*,*,#8871,.T.);
#12043=ORIENTED_EDGE('',*,*,#8750,.F.);
#12044=ORIENTED_EDGE('',*,*,#8872,.T.);
#12045=ORIENTED_EDGE('',*,*,#8751,.F.);
#12046=ORIENTED_EDGE('',*,*,#8759,.T.);
#12047=ORIENTED_EDGE('',*,*,#8377,.T.);
#12048=ORIENTED_EDGE('',*,*,#8744,.F.);
#12049=ORIENTED_EDGE('',*,*,#8764,.F.);
#12050=ORIENTED_EDGE('',*,*,#8873,.T.);
#12051=ORIENTED_EDGE('',*,*,#8765,.F.);
#12052=ORIENTED_EDGE('',*,*,#8773,.T.);
#12053=ORIENTED_EDGE('',*,*,#8379,.T.);
#12054=ORIENTED_EDGE('',*,*,#8758,.F.);
#12055=ORIENTED_EDGE('',*,*,#8778,.F.);
#12056=ORIENTED_EDGE('',*,*,#8874,.T.);
#12057=ORIENTED_EDGE('',*,*,#8779,.F.);
#12058=ORIENTED_EDGE('',*,*,#8787,.T.);
#12059=ORIENTED_EDGE('',*,*,#8381,.T.);
#12060=ORIENTED_EDGE('',*,*,#8772,.F.);
#12061=ORIENTED_EDGE('',*,*,#8792,.F.);
#12062=ORIENTED_EDGE('',*,*,#8875,.T.);
#12063=ORIENTED_EDGE('',*,*,#8793,.F.);
#12064=ORIENTED_EDGE('',*,*,#8801,.T.);
#12065=ORIENTED_EDGE('',*,*,#8383,.T.);
#12066=ORIENTED_EDGE('',*,*,#8786,.F.);
#12067=ORIENTED_EDGE('',*,*,#8791,.F.);
#12068=ORIENTED_EDGE('',*,*,#8876,.F.);
#12069=ORIENTED_EDGE('',*,*,#8794,.F.);
#12070=ORIENTED_EDGE('',*,*,#8875,.F.);
#12071=ORIENTED_EDGE('',*,*,#8777,.F.);
#12072=ORIENTED_EDGE('',*,*,#8877,.F.);
#12073=ORIENTED_EDGE('',*,*,#8780,.F.);
#12074=ORIENTED_EDGE('',*,*,#8874,.F.);
#12075=ORIENTED_EDGE('',*,*,#8763,.F.);
#12076=ORIENTED_EDGE('',*,*,#8878,.F.);
#12077=ORIENTED_EDGE('',*,*,#8766,.F.);
#12078=ORIENTED_EDGE('',*,*,#8873,.F.);
#12079=ORIENTED_EDGE('',*,*,#8749,.F.);
#12080=ORIENTED_EDGE('',*,*,#8879,.F.);
#12081=ORIENTED_EDGE('',*,*,#8752,.F.);
#12082=ORIENTED_EDGE('',*,*,#8872,.F.);
#12083=ORIENTED_EDGE('',*,*,#8738,.F.);
#12084=ORIENTED_EDGE('',*,*,#8871,.F.);
#12085=ORIENTED_EDGE('',*,*,#8868,.F.);
#12086=ORIENTED_EDGE('',*,*,#8880,.F.);
#12087=ORIENTED_EDGE('',*,*,#8861,.T.);
#12088=ORIENTED_EDGE('',*,*,#8865,.T.);
#12089=ORIENTED_EDGE('',*,*,#8881,.T.);
#12090=ORIENTED_EDGE('',*,*,#8882,.T.);
#12091=ORIENTED_EDGE('',*,*,#8826,.F.);
#12092=ORIENTED_EDGE('',*,*,#8883,.T.);
#12093=ORIENTED_EDGE('',*,*,#8830,.F.);
#12094=ORIENTED_EDGE('',*,*,#8835,.T.);
#12095=ORIENTED_EDGE('',*,*,#8368,.T.);
#12096=ORIENTED_EDGE('',*,*,#8820,.F.);
#12097=ORIENTED_EDGE('',*,*,#8840,.F.);
#12098=ORIENTED_EDGE('',*,*,#8884,.T.);
#12099=ORIENTED_EDGE('',*,*,#8844,.F.);
#12100=ORIENTED_EDGE('',*,*,#8849,.T.);
#12101=ORIENTED_EDGE('',*,*,#8370,.T.);
#12102=ORIENTED_EDGE('',*,*,#8834,.F.);
#12103=ORIENTED_EDGE('',*,*,#8854,.F.);
#12104=ORIENTED_EDGE('',*,*,#8885,.T.);
#12105=ORIENTED_EDGE('',*,*,#8858,.F.);
#12106=ORIENTED_EDGE('',*,*,#8863,.T.);
#12107=ORIENTED_EDGE('',*,*,#8372,.T.);
#12108=ORIENTED_EDGE('',*,*,#8848,.F.);
#12109=ORIENTED_EDGE('',*,*,#8870,.F.);
#12110=ORIENTED_EDGE('',*,*,#8374,.F.);
#12111=ORIENTED_EDGE('',*,*,#8862,.T.);
#12112=ORIENTED_EDGE('',*,*,#8882,.F.);
#12113=ORIENTED_EDGE('',*,*,#8886,.T.);
#12114=ORIENTED_EDGE('',*,*,#8866,.F.);
#12115=ORIENTED_EDGE('',*,*,#8853,.F.);
#12116=ORIENTED_EDGE('',*,*,#8887,.T.);
#12117=ORIENTED_EDGE('',*,*,#8859,.F.);
#12118=ORIENTED_EDGE('',*,*,#8885,.F.);
#12119=ORIENTED_EDGE('',*,*,#8839,.F.);
#12120=ORIENTED_EDGE('',*,*,#8888,.T.);
#12121=ORIENTED_EDGE('',*,*,#8845,.F.);
#12122=ORIENTED_EDGE('',*,*,#8884,.F.);
#12123=ORIENTED_EDGE('',*,*,#8825,.F.);
#12124=ORIENTED_EDGE('',*,*,#8889,.T.);
#12125=ORIENTED_EDGE('',*,*,#8831,.F.);
#12126=ORIENTED_EDGE('',*,*,#8883,.F.);
#12127=ORIENTED_EDGE('',*,*,#8890,.T.);
#12128=ORIENTED_EDGE('',*,*,#8891,.T.);
#12129=ORIENTED_EDGE('',*,*,#8892,.T.);
#12130=ORIENTED_EDGE('',*,*,#8893,.T.);
#12131=ORIENTED_EDGE('',*,*,#8894,.T.);
#12132=ORIENTED_EDGE('',*,*,#8894,.F.);
#12133=ORIENTED_EDGE('',*,*,#8895,.T.);
#12134=ORIENTED_EDGE('',*,*,#8896,.F.);
#12135=ORIENTED_EDGE('',*,*,#8897,.F.);
#12136=ORIENTED_EDGE('',*,*,#8354,.T.);
#12137=ORIENTED_EDGE('',*,*,#8898,.F.);
#12138=ORIENTED_EDGE('',*,*,#8893,.F.);
#12139=ORIENTED_EDGE('',*,*,#8899,.T.);
#12140=ORIENTED_EDGE('',*,*,#8900,.F.);
#12141=ORIENTED_EDGE('',*,*,#8895,.F.);
#12142=ORIENTED_EDGE('',*,*,#8901,.F.);
#12143=ORIENTED_EDGE('',*,*,#8902,.T.);
#12144=ORIENTED_EDGE('',*,*,#8903,.T.);
#12145=ORIENTED_EDGE('',*,*,#8896,.T.);
#12146=ORIENTED_EDGE('',*,*,#8900,.T.);
#12147=ORIENTED_EDGE('',*,*,#8903,.F.);
#12148=ORIENTED_EDGE('',*,*,#8904,.T.);
#12149=ORIENTED_EDGE('',*,*,#8905,.F.);
#12150=ORIENTED_EDGE('',*,*,#8906,.T.);
#12151=ORIENTED_EDGE('',*,*,#8355,.T.);
#12152=ORIENTED_EDGE('',*,*,#8897,.T.);
#12153=ORIENTED_EDGE('',*,*,#8905,.T.);
#12154=ORIENTED_EDGE('',*,*,#8907,.T.);
#12155=ORIENTED_EDGE('',*,*,#8908,.T.);
#12156=ORIENTED_EDGE('',*,*,#8909,.T.);
#12157=ORIENTED_EDGE('',*,*,#8910,.T.);
#12158=ORIENTED_EDGE('',*,*,#8910,.F.);
#12159=ORIENTED_EDGE('',*,*,#8911,.T.);
#12160=ORIENTED_EDGE('',*,*,#8912,.F.);
#12161=ORIENTED_EDGE('',*,*,#8913,.T.);
#12162=ORIENTED_EDGE('',*,*,#8356,.T.);
#12163=ORIENTED_EDGE('',*,*,#8906,.F.);
#12164=ORIENTED_EDGE('',*,*,#8909,.F.);
#12165=ORIENTED_EDGE('',*,*,#8914,.T.);
#12166=ORIENTED_EDGE('',*,*,#8915,.F.);
#12167=ORIENTED_EDGE('',*,*,#8911,.F.);
#12168=ORIENTED_EDGE('',*,*,#8916,.F.);
#12169=ORIENTED_EDGE('',*,*,#8917,.T.);
#12170=ORIENTED_EDGE('',*,*,#8918,.T.);
#12171=ORIENTED_EDGE('',*,*,#8912,.T.);
#12172=ORIENTED_EDGE('',*,*,#8915,.T.);
#12173=ORIENTED_EDGE('',*,*,#8919,.T.);
#12174=ORIENTED_EDGE('',*,*,#8920,.T.);
#12175=ORIENTED_EDGE('',*,*,#8921,.T.);
#12176=ORIENTED_EDGE('',*,*,#8922,.T.);
#12177=ORIENTED_EDGE('',*,*,#8923,.T.);
#12178=ORIENTED_EDGE('',*,*,#8923,.F.);
#12179=ORIENTED_EDGE('',*,*,#8924,.T.);
#12180=ORIENTED_EDGE('',*,*,#8925,.F.);
#12181=ORIENTED_EDGE('',*,*,#8926,.T.);
#12182=ORIENTED_EDGE('',*,*,#8358,.T.);
#12183=ORIENTED_EDGE('',*,*,#8927,.F.);
#12184=ORIENTED_EDGE('',*,*,#8922,.F.);
#12185=ORIENTED_EDGE('',*,*,#8928,.T.);
#12186=ORIENTED_EDGE('',*,*,#8929,.F.);
#12187=ORIENTED_EDGE('',*,*,#8924,.F.);
#12188=ORIENTED_EDGE('',*,*,#8930,.F.);
#12189=ORIENTED_EDGE('',*,*,#8931,.T.);
#12190=ORIENTED_EDGE('',*,*,#8932,.T.);
#12191=ORIENTED_EDGE('',*,*,#8925,.T.);
#12192=ORIENTED_EDGE('',*,*,#8929,.T.);
#12193=ORIENTED_EDGE('',*,*,#8933,.T.);
#12194=ORIENTED_EDGE('',*,*,#8934,.T.);
#12195=ORIENTED_EDGE('',*,*,#8935,.T.);
#12196=ORIENTED_EDGE('',*,*,#8936,.T.);
#12197=ORIENTED_EDGE('',*,*,#8937,.T.);
#12198=ORIENTED_EDGE('',*,*,#8937,.F.);
#12199=ORIENTED_EDGE('',*,*,#8938,.T.);
#12200=ORIENTED_EDGE('',*,*,#8939,.F.);
#12201=ORIENTED_EDGE('',*,*,#8940,.T.);
#12202=ORIENTED_EDGE('',*,*,#8360,.T.);
#12203=ORIENTED_EDGE('',*,*,#8941,.F.);
#12204=ORIENTED_EDGE('',*,*,#8936,.F.);
#12205=ORIENTED_EDGE('',*,*,#8942,.T.);
#12206=ORIENTED_EDGE('',*,*,#8943,.F.);
#12207=ORIENTED_EDGE('',*,*,#8938,.F.);
#12208=ORIENTED_EDGE('',*,*,#8944,.F.);
#12209=ORIENTED_EDGE('',*,*,#8945,.T.);
#12210=ORIENTED_EDGE('',*,*,#8946,.T.);
#12211=ORIENTED_EDGE('',*,*,#8939,.T.);
#12212=ORIENTED_EDGE('',*,*,#8943,.T.);
#12213=ORIENTED_EDGE('',*,*,#8947,.T.);
#12214=ORIENTED_EDGE('',*,*,#8948,.T.);
#12215=ORIENTED_EDGE('',*,*,#8949,.T.);
#12216=ORIENTED_EDGE('',*,*,#8950,.T.);
#12217=ORIENTED_EDGE('',*,*,#8951,.T.);
#12218=ORIENTED_EDGE('',*,*,#8951,.F.);
#12219=ORIENTED_EDGE('',*,*,#8952,.T.);
#12220=ORIENTED_EDGE('',*,*,#8953,.F.);
#12221=ORIENTED_EDGE('',*,*,#8954,.T.);
#12222=ORIENTED_EDGE('',*,*,#8362,.T.);
#12223=ORIENTED_EDGE('',*,*,#8955,.F.);
#12224=ORIENTED_EDGE('',*,*,#8950,.F.);
#12225=ORIENTED_EDGE('',*,*,#8956,.T.);
#12226=ORIENTED_EDGE('',*,*,#8957,.F.);
#12227=ORIENTED_EDGE('',*,*,#8952,.F.);
#12228=ORIENTED_EDGE('',*,*,#8958,.F.);
#12229=ORIENTED_EDGE('',*,*,#8959,.T.);
#12230=ORIENTED_EDGE('',*,*,#8960,.T.);
#12231=ORIENTED_EDGE('',*,*,#8953,.T.);
#12232=ORIENTED_EDGE('',*,*,#8957,.T.);
#12233=ORIENTED_EDGE('',*,*,#8961,.T.);
#12234=ORIENTED_EDGE('',*,*,#8962,.T.);
#12235=ORIENTED_EDGE('',*,*,#8963,.T.);
#12236=ORIENTED_EDGE('',*,*,#8964,.T.);
#12237=ORIENTED_EDGE('',*,*,#8965,.T.);
#12238=ORIENTED_EDGE('',*,*,#8965,.F.);
#12239=ORIENTED_EDGE('',*,*,#8966,.T.);
#12240=ORIENTED_EDGE('',*,*,#8967,.F.);
#12241=ORIENTED_EDGE('',*,*,#8968,.T.);
#12242=ORIENTED_EDGE('',*,*,#8364,.T.);
#12243=ORIENTED_EDGE('',*,*,#8969,.F.);
#12244=ORIENTED_EDGE('',*,*,#8964,.F.);
#12245=ORIENTED_EDGE('',*,*,#8970,.T.);
#12246=ORIENTED_EDGE('',*,*,#8971,.F.);
#12247=ORIENTED_EDGE('',*,*,#8966,.F.);
#12248=ORIENTED_EDGE('',*,*,#8972,.T.);
#12249=ORIENTED_EDGE('',*,*,#8973,.T.);
#12250=ORIENTED_EDGE('',*,*,#8974,.T.);
#12251=ORIENTED_EDGE('',*,*,#8975,.T.);
#12252=ORIENTED_EDGE('',*,*,#8973,.F.);
#12253=ORIENTED_EDGE('',*,*,#8976,.F.);
#12254=ORIENTED_EDGE('',*,*,#8977,.F.);
#12255=ORIENTED_EDGE('',*,*,#8978,.F.);
#12256=ORIENTED_EDGE('',*,*,#8972,.F.);
#12257=ORIENTED_EDGE('',*,*,#8979,.F.);
#12258=ORIENTED_EDGE('',*,*,#8365,.T.);
#12259=ORIENTED_EDGE('',*,*,#8968,.F.);
#12260=ORIENTED_EDGE('',*,*,#8980,.F.);
#12261=ORIENTED_EDGE('',*,*,#8976,.T.);
#12262=ORIENTED_EDGE('',*,*,#8981,.F.);
#12263=ORIENTED_EDGE('',*,*,#8977,.T.);
#12264=ORIENTED_EDGE('',*,*,#8980,.T.);
#12265=ORIENTED_EDGE('',*,*,#8967,.T.);
#12266=ORIENTED_EDGE('',*,*,#8971,.T.);
#12267=ORIENTED_EDGE('',*,*,#8982,.F.);
#12268=ORIENTED_EDGE('',*,*,#8983,.T.);
#12269=ORIENTED_EDGE('',*,*,#8984,.T.);
#12270=ORIENTED_EDGE('',*,*,#8985,.T.);
#12271=ORIENTED_EDGE('',*,*,#8984,.F.);
#12272=ORIENTED_EDGE('',*,*,#8986,.T.);
#12273=ORIENTED_EDGE('',*,*,#8987,.F.);
#12274=ORIENTED_EDGE('',*,*,#8988,.T.);
#12275=ORIENTED_EDGE('',*,*,#8347,.T.);
#12276=ORIENTED_EDGE('',*,*,#8989,.F.);
#12277=ORIENTED_EDGE('',*,*,#8983,.F.);
#12278=ORIENTED_EDGE('',*,*,#8990,.F.);
#12279=ORIENTED_EDGE('',*,*,#8991,.F.);
#12280=ORIENTED_EDGE('',*,*,#8986,.F.);
#12281=ORIENTED_EDGE('',*,*,#8987,.T.);
#12282=ORIENTED_EDGE('',*,*,#8991,.T.);
#12283=ORIENTED_EDGE('',*,*,#8992,.T.);
#12284=ORIENTED_EDGE('',*,*,#8993,.T.);
#12285=ORIENTED_EDGE('',*,*,#8994,.T.);
#12286=ORIENTED_EDGE('',*,*,#8995,.F.);
#12287=ORIENTED_EDGE('',*,*,#8996,.T.);
#12288=ORIENTED_EDGE('',*,*,#8997,.T.);
#12289=ORIENTED_EDGE('',*,*,#8998,.T.);
#12290=ORIENTED_EDGE('',*,*,#8999,.T.);
#12291=ORIENTED_EDGE('',*,*,#8997,.F.);
#12292=ORIENTED_EDGE('',*,*,#9000,.T.);
#12293=ORIENTED_EDGE('',*,*,#9001,.F.);
#12294=ORIENTED_EDGE('',*,*,#9002,.T.);
#12295=ORIENTED_EDGE('',*,*,#8349,.T.);
#12296=ORIENTED_EDGE('',*,*,#9003,.F.);
#12297=ORIENTED_EDGE('',*,*,#8996,.F.);
#12298=ORIENTED_EDGE('',*,*,#9004,.F.);
#12299=ORIENTED_EDGE('',*,*,#9005,.F.);
#12300=ORIENTED_EDGE('',*,*,#9000,.F.);
#12301=ORIENTED_EDGE('',*,*,#9001,.T.);
#12302=ORIENTED_EDGE('',*,*,#9005,.T.);
#12303=ORIENTED_EDGE('',*,*,#9006,.T.);
#12304=ORIENTED_EDGE('',*,*,#9007,.T.);
#12305=ORIENTED_EDGE('',*,*,#9008,.T.);
#12306=ORIENTED_EDGE('',*,*,#9009,.F.);
#12307=ORIENTED_EDGE('',*,*,#9010,.T.);
#12308=ORIENTED_EDGE('',*,*,#9011,.T.);
#12309=ORIENTED_EDGE('',*,*,#9012,.T.);
#12310=ORIENTED_EDGE('',*,*,#9013,.T.);
#12311=ORIENTED_EDGE('',*,*,#9011,.F.);
#12312=ORIENTED_EDGE('',*,*,#9014,.T.);
#12313=ORIENTED_EDGE('',*,*,#9015,.F.);
#12314=ORIENTED_EDGE('',*,*,#9016,.F.);
#12315=ORIENTED_EDGE('',*,*,#8351,.T.);
#12316=ORIENTED_EDGE('',*,*,#9017,.T.);
#12317=ORIENTED_EDGE('',*,*,#9010,.F.);
#12318=ORIENTED_EDGE('',*,*,#9018,.F.);
#12319=ORIENTED_EDGE('',*,*,#9019,.F.);
#12320=ORIENTED_EDGE('',*,*,#9014,.F.);
#12321=ORIENTED_EDGE('',*,*,#9020,.T.);
#12322=ORIENTED_EDGE('',*,*,#9021,.F.);
#12323=ORIENTED_EDGE('',*,*,#9022,.T.);
#12324=ORIENTED_EDGE('',*,*,#9023,.T.);
#12325=ORIENTED_EDGE('',*,*,#8890,.F.);
#12326=ORIENTED_EDGE('',*,*,#8898,.T.);
#12327=ORIENTED_EDGE('',*,*,#8353,.T.);
#12328=ORIENTED_EDGE('',*,*,#9024,.T.);
#12329=ORIENTED_EDGE('',*,*,#9023,.F.);
#12330=ORIENTED_EDGE('',*,*,#9025,.T.);
#12331=ORIENTED_EDGE('',*,*,#8918,.F.);
#12332=ORIENTED_EDGE('',*,*,#9026,.T.);
#12333=ORIENTED_EDGE('',*,*,#8919,.F.);
#12334=ORIENTED_EDGE('',*,*,#8927,.T.);
#12335=ORIENTED_EDGE('',*,*,#8357,.T.);
#12336=ORIENTED_EDGE('',*,*,#8913,.F.);
#12337=ORIENTED_EDGE('',*,*,#8932,.F.);
#12338=ORIENTED_EDGE('',*,*,#9027,.T.);
#12339=ORIENTED_EDGE('',*,*,#8933,.F.);
#12340=ORIENTED_EDGE('',*,*,#8941,.T.);
#12341=ORIENTED_EDGE('',*,*,#8359,.T.);
#12342=ORIENTED_EDGE('',*,*,#8926,.F.);
#12343=ORIENTED_EDGE('',*,*,#8946,.F.);
#12344=ORIENTED_EDGE('',*,*,#9028,.T.);
#12345=ORIENTED_EDGE('',*,*,#8947,.F.);
#12346=ORIENTED_EDGE('',*,*,#8955,.T.);
#12347=ORIENTED_EDGE('',*,*,#8361,.T.);
#12348=ORIENTED_EDGE('',*,*,#8940,.F.);
#12349=ORIENTED_EDGE('',*,*,#8960,.F.);
#12350=ORIENTED_EDGE('',*,*,#9029,.T.);
#12351=ORIENTED_EDGE('',*,*,#8961,.F.);
#12352=ORIENTED_EDGE('',*,*,#8969,.T.);
#12353=ORIENTED_EDGE('',*,*,#8363,.T.);
#12354=ORIENTED_EDGE('',*,*,#8954,.F.);
#12355=ORIENTED_EDGE('',*,*,#8959,.F.);
#12356=ORIENTED_EDGE('',*,*,#9030,.F.);
#12357=ORIENTED_EDGE('',*,*,#8962,.F.);
#12358=ORIENTED_EDGE('',*,*,#9029,.F.);
#12359=ORIENTED_EDGE('',*,*,#8945,.F.);
#12360=ORIENTED_EDGE('',*,*,#9031,.F.);
#12361=ORIENTED_EDGE('',*,*,#8948,.F.);
#12362=ORIENTED_EDGE('',*,*,#9028,.F.);
#12363=ORIENTED_EDGE('',*,*,#8931,.F.);
#12364=ORIENTED_EDGE('',*,*,#9032,.F.);
#12365=ORIENTED_EDGE('',*,*,#8934,.F.);
#12366=ORIENTED_EDGE('',*,*,#9027,.F.);
#12367=ORIENTED_EDGE('',*,*,#8917,.F.);
#12368=ORIENTED_EDGE('',*,*,#9033,.F.);
#12369=ORIENTED_EDGE('',*,*,#8920,.F.);
#12370=ORIENTED_EDGE('',*,*,#9026,.F.);
#12371=ORIENTED_EDGE('',*,*,#8902,.F.);
#12372=ORIENTED_EDGE('',*,*,#9034,.F.);
#12373=ORIENTED_EDGE('',*,*,#8907,.F.);
#12374=ORIENTED_EDGE('',*,*,#8904,.F.);
#12375=ORIENTED_EDGE('',*,*,#8891,.F.);
#12376=ORIENTED_EDGE('',*,*,#9025,.F.);
#12377=ORIENTED_EDGE('',*,*,#9022,.F.);
#12378=ORIENTED_EDGE('',*,*,#9035,.F.);
#12379=ORIENTED_EDGE('',*,*,#9015,.T.);
#12380=ORIENTED_EDGE('',*,*,#9019,.T.);
#12381=ORIENTED_EDGE('',*,*,#9036,.T.);
#12382=ORIENTED_EDGE('',*,*,#9037,.T.);
#12383=ORIENTED_EDGE('',*,*,#8994,.F.);
#12384=ORIENTED_EDGE('',*,*,#9038,.T.);
#12385=ORIENTED_EDGE('',*,*,#8998,.F.);
#12386=ORIENTED_EDGE('',*,*,#9003,.T.);
#12387=ORIENTED_EDGE('',*,*,#8348,.T.);
#12388=ORIENTED_EDGE('',*,*,#8988,.F.);
#12389=ORIENTED_EDGE('',*,*,#9008,.F.);
#12390=ORIENTED_EDGE('',*,*,#9039,.T.);
#12391=ORIENTED_EDGE('',*,*,#9012,.F.);
#12392=ORIENTED_EDGE('',*,*,#9017,.F.);
#12393=ORIENTED_EDGE('',*,*,#8350,.T.);
#12394=ORIENTED_EDGE('',*,*,#9002,.F.);
#12395=ORIENTED_EDGE('',*,*,#9024,.F.);
#12396=ORIENTED_EDGE('',*,*,#8352,.F.);
#12397=ORIENTED_EDGE('',*,*,#9016,.T.);
#12398=ORIENTED_EDGE('',*,*,#9037,.F.);
#12399=ORIENTED_EDGE('',*,*,#9040,.T.);
#12400=ORIENTED_EDGE('',*,*,#9020,.F.);
#12401=ORIENTED_EDGE('',*,*,#9007,.F.);
#12402=ORIENTED_EDGE('',*,*,#9041,.T.);
#12403=ORIENTED_EDGE('',*,*,#9013,.F.);
#12404=ORIENTED_EDGE('',*,*,#9039,.F.);
#12405=ORIENTED_EDGE('',*,*,#8993,.F.);
#12406=ORIENTED_EDGE('',*,*,#9042,.T.);
#12407=ORIENTED_EDGE('',*,*,#8999,.F.);
#12408=ORIENTED_EDGE('',*,*,#9038,.F.);
#12409=ORIENTED_EDGE('',*,*,#9043,.T.);
#12410=ORIENTED_EDGE('',*,*,#9044,.T.);
#12411=ORIENTED_EDGE('',*,*,#9045,.T.);
#12412=ORIENTED_EDGE('',*,*,#9046,.T.);
#12413=ORIENTED_EDGE('',*,*,#9047,.T.);
#12414=ORIENTED_EDGE('',*,*,#9047,.F.);
#12415=ORIENTED_EDGE('',*,*,#9048,.T.);
#12416=ORIENTED_EDGE('',*,*,#9049,.F.);
#12417=ORIENTED_EDGE('',*,*,#9050,.T.);
#12418=ORIENTED_EDGE('',*,*,#8332,.T.);
#12419=ORIENTED_EDGE('',*,*,#9051,.F.);
#12420=ORIENTED_EDGE('',*,*,#9046,.F.);
#12421=ORIENTED_EDGE('',*,*,#9052,.T.);
#12422=ORIENTED_EDGE('',*,*,#9053,.F.);
#12423=ORIENTED_EDGE('',*,*,#9048,.F.);
#12424=ORIENTED_EDGE('',*,*,#9054,.F.);
#12425=ORIENTED_EDGE('',*,*,#9055,.T.);
#12426=ORIENTED_EDGE('',*,*,#9056,.T.);
#12427=ORIENTED_EDGE('',*,*,#9049,.T.);
#12428=ORIENTED_EDGE('',*,*,#9053,.T.);
#12429=ORIENTED_EDGE('',*,*,#9057,.T.);
#12430=ORIENTED_EDGE('',*,*,#9058,.T.);
#12431=ORIENTED_EDGE('',*,*,#9059,.T.);
#12432=ORIENTED_EDGE('',*,*,#9060,.T.);
#12433=ORIENTED_EDGE('',*,*,#9061,.T.);
#12434=ORIENTED_EDGE('',*,*,#9061,.F.);
#12435=ORIENTED_EDGE('',*,*,#9062,.T.);
#12436=ORIENTED_EDGE('',*,*,#9063,.F.);
#12437=ORIENTED_EDGE('',*,*,#9064,.T.);
#12438=ORIENTED_EDGE('',*,*,#8334,.T.);
#12439=ORIENTED_EDGE('',*,*,#9065,.F.);
#12440=ORIENTED_EDGE('',*,*,#9060,.F.);
#12441=ORIENTED_EDGE('',*,*,#9066,.T.);
#12442=ORIENTED_EDGE('',*,*,#9067,.F.);
#12443=ORIENTED_EDGE('',*,*,#9062,.F.);
#12444=ORIENTED_EDGE('',*,*,#9068,.F.);
#12445=ORIENTED_EDGE('',*,*,#9069,.T.);
#12446=ORIENTED_EDGE('',*,*,#9070,.T.);
#12447=ORIENTED_EDGE('',*,*,#9063,.T.);
#12448=ORIENTED_EDGE('',*,*,#9067,.T.);
#12449=ORIENTED_EDGE('',*,*,#9071,.T.);
#12450=ORIENTED_EDGE('',*,*,#9072,.T.);
#12451=ORIENTED_EDGE('',*,*,#9073,.T.);
#12452=ORIENTED_EDGE('',*,*,#9074,.T.);
#12453=ORIENTED_EDGE('',*,*,#9075,.T.);
#12454=ORIENTED_EDGE('',*,*,#9075,.F.);
#12455=ORIENTED_EDGE('',*,*,#9076,.T.);
#12456=ORIENTED_EDGE('',*,*,#9077,.F.);
#12457=ORIENTED_EDGE('',*,*,#9078,.T.);
#12458=ORIENTED_EDGE('',*,*,#8336,.T.);
#12459=ORIENTED_EDGE('',*,*,#9079,.F.);
#12460=ORIENTED_EDGE('',*,*,#9074,.F.);
#12461=ORIENTED_EDGE('',*,*,#9080,.T.);
#12462=ORIENTED_EDGE('',*,*,#9081,.F.);
#12463=ORIENTED_EDGE('',*,*,#9076,.F.);
#12464=ORIENTED_EDGE('',*,*,#9082,.F.);
#12465=ORIENTED_EDGE('',*,*,#9083,.T.);
#12466=ORIENTED_EDGE('',*,*,#9084,.T.);
#12467=ORIENTED_EDGE('',*,*,#9077,.T.);
#12468=ORIENTED_EDGE('',*,*,#9081,.T.);
#12469=ORIENTED_EDGE('',*,*,#9085,.T.);
#12470=ORIENTED_EDGE('',*,*,#9086,.T.);
#12471=ORIENTED_EDGE('',*,*,#9087,.T.);
#12472=ORIENTED_EDGE('',*,*,#9088,.T.);
#12473=ORIENTED_EDGE('',*,*,#9089,.T.);
#12474=ORIENTED_EDGE('',*,*,#9089,.F.);
#12475=ORIENTED_EDGE('',*,*,#9090,.T.);
#12476=ORIENTED_EDGE('',*,*,#9091,.F.);
#12477=ORIENTED_EDGE('',*,*,#9092,.T.);
#12478=ORIENTED_EDGE('',*,*,#8338,.T.);
#12479=ORIENTED_EDGE('',*,*,#9093,.F.);
#12480=ORIENTED_EDGE('',*,*,#9088,.F.);
#12481=ORIENTED_EDGE('',*,*,#9094,.T.);
#12482=ORIENTED_EDGE('',*,*,#9095,.F.);
#12483=ORIENTED_EDGE('',*,*,#9090,.F.);
#12484=ORIENTED_EDGE('',*,*,#9096,.F.);
#12485=ORIENTED_EDGE('',*,*,#9097,.T.);
#12486=ORIENTED_EDGE('',*,*,#9098,.T.);
#12487=ORIENTED_EDGE('',*,*,#9091,.T.);
#12488=ORIENTED_EDGE('',*,*,#9095,.T.);
#12489=ORIENTED_EDGE('',*,*,#9099,.T.);
#12490=ORIENTED_EDGE('',*,*,#9100,.T.);
#12491=ORIENTED_EDGE('',*,*,#9101,.T.);
#12492=ORIENTED_EDGE('',*,*,#9102,.T.);
#12493=ORIENTED_EDGE('',*,*,#9103,.T.);
#12494=ORIENTED_EDGE('',*,*,#9103,.F.);
#12495=ORIENTED_EDGE('',*,*,#9104,.T.);
#12496=ORIENTED_EDGE('',*,*,#9105,.F.);
#12497=ORIENTED_EDGE('',*,*,#9106,.T.);
#12498=ORIENTED_EDGE('',*,*,#8340,.T.);
#12499=ORIENTED_EDGE('',*,*,#9107,.F.);
#12500=ORIENTED_EDGE('',*,*,#9102,.F.);
#12501=ORIENTED_EDGE('',*,*,#9108,.T.);
#12502=ORIENTED_EDGE('',*,*,#9109,.F.);
#12503=ORIENTED_EDGE('',*,*,#9104,.F.);
#12504=ORIENTED_EDGE('',*,*,#9110,.F.);
#12505=ORIENTED_EDGE('',*,*,#9111,.T.);
#12506=ORIENTED_EDGE('',*,*,#9112,.T.);
#12507=ORIENTED_EDGE('',*,*,#9105,.T.);
#12508=ORIENTED_EDGE('',*,*,#9109,.T.);
#12509=ORIENTED_EDGE('',*,*,#9113,.T.);
#12510=ORIENTED_EDGE('',*,*,#9114,.T.);
#12511=ORIENTED_EDGE('',*,*,#9115,.T.);
#12512=ORIENTED_EDGE('',*,*,#9116,.T.);
#12513=ORIENTED_EDGE('',*,*,#9117,.T.);
#12514=ORIENTED_EDGE('',*,*,#9117,.F.);
#12515=ORIENTED_EDGE('',*,*,#9118,.T.);
#12516=ORIENTED_EDGE('',*,*,#9119,.F.);
#12517=ORIENTED_EDGE('',*,*,#9120,.T.);
#12518=ORIENTED_EDGE('',*,*,#8342,.T.);
#12519=ORIENTED_EDGE('',*,*,#9121,.F.);
#12520=ORIENTED_EDGE('',*,*,#9116,.F.);
#12521=ORIENTED_EDGE('',*,*,#9122,.T.);
#12522=ORIENTED_EDGE('',*,*,#9123,.F.);
#12523=ORIENTED_EDGE('',*,*,#9118,.F.);
#12524=ORIENTED_EDGE('',*,*,#9124,.F.);
#12525=ORIENTED_EDGE('',*,*,#9125,.T.);
#12526=ORIENTED_EDGE('',*,*,#9126,.T.);
#12527=ORIENTED_EDGE('',*,*,#9119,.T.);
#12528=ORIENTED_EDGE('',*,*,#9123,.T.);
#12529=ORIENTED_EDGE('',*,*,#9127,.T.);
#12530=ORIENTED_EDGE('',*,*,#9128,.T.);
#12531=ORIENTED_EDGE('',*,*,#9129,.T.);
#12532=ORIENTED_EDGE('',*,*,#9130,.T.);
#12533=ORIENTED_EDGE('',*,*,#9131,.T.);
#12534=ORIENTED_EDGE('',*,*,#9131,.F.);
#12535=ORIENTED_EDGE('',*,*,#9132,.T.);
#12536=ORIENTED_EDGE('',*,*,#9133,.F.);
#12537=ORIENTED_EDGE('',*,*,#9134,.T.);
#12538=ORIENTED_EDGE('',*,*,#8344,.T.);
#12539=ORIENTED_EDGE('',*,*,#9135,.F.);
#12540=ORIENTED_EDGE('',*,*,#9130,.F.);
#12541=ORIENTED_EDGE('',*,*,#9136,.T.);
#12542=ORIENTED_EDGE('',*,*,#9137,.F.);
#12543=ORIENTED_EDGE('',*,*,#9132,.F.);
#12544=ORIENTED_EDGE('',*,*,#9138,.T.);
#12545=ORIENTED_EDGE('',*,*,#9139,.T.);
#12546=ORIENTED_EDGE('',*,*,#9140,.T.);
#12547=ORIENTED_EDGE('',*,*,#9141,.T.);
#12548=ORIENTED_EDGE('',*,*,#9139,.F.);
#12549=ORIENTED_EDGE('',*,*,#9142,.F.);
#12550=ORIENTED_EDGE('',*,*,#9143,.F.);
#12551=ORIENTED_EDGE('',*,*,#9144,.F.);
#12552=ORIENTED_EDGE('',*,*,#9138,.F.);
#12553=ORIENTED_EDGE('',*,*,#9145,.F.);
#12554=ORIENTED_EDGE('',*,*,#8345,.T.);
#12555=ORIENTED_EDGE('',*,*,#9134,.F.);
#12556=ORIENTED_EDGE('',*,*,#9146,.F.);
#12557=ORIENTED_EDGE('',*,*,#9142,.T.);
#12558=ORIENTED_EDGE('',*,*,#9147,.F.);
#12559=ORIENTED_EDGE('',*,*,#9143,.T.);
#12560=ORIENTED_EDGE('',*,*,#9146,.T.);
#12561=ORIENTED_EDGE('',*,*,#9133,.T.);
#12562=ORIENTED_EDGE('',*,*,#9137,.T.);
#12563=ORIENTED_EDGE('',*,*,#9148,.F.);
#12564=ORIENTED_EDGE('',*,*,#9149,.T.);
#12565=ORIENTED_EDGE('',*,*,#9150,.T.);
#12566=ORIENTED_EDGE('',*,*,#9151,.T.);
#12567=ORIENTED_EDGE('',*,*,#9150,.F.);
#12568=ORIENTED_EDGE('',*,*,#9152,.T.);
#12569=ORIENTED_EDGE('',*,*,#9153,.F.);
#12570=ORIENTED_EDGE('',*,*,#9154,.T.);
#12571=ORIENTED_EDGE('',*,*,#8327,.T.);
#12572=ORIENTED_EDGE('',*,*,#9155,.F.);
#12573=ORIENTED_EDGE('',*,*,#9149,.F.);
#12574=ORIENTED_EDGE('',*,*,#9156,.F.);
#12575=ORIENTED_EDGE('',*,*,#9157,.F.);
#12576=ORIENTED_EDGE('',*,*,#9152,.F.);
#12577=ORIENTED_EDGE('',*,*,#9153,.T.);
#12578=ORIENTED_EDGE('',*,*,#9157,.T.);
#12579=ORIENTED_EDGE('',*,*,#9158,.T.);
#12580=ORIENTED_EDGE('',*,*,#9159,.T.);
#12581=ORIENTED_EDGE('',*,*,#9160,.T.);
#12582=ORIENTED_EDGE('',*,*,#9161,.F.);
#12583=ORIENTED_EDGE('',*,*,#9162,.T.);
#12584=ORIENTED_EDGE('',*,*,#9163,.T.);
#12585=ORIENTED_EDGE('',*,*,#9164,.T.);
#12586=ORIENTED_EDGE('',*,*,#9165,.T.);
#12587=ORIENTED_EDGE('',*,*,#9163,.F.);
#12588=ORIENTED_EDGE('',*,*,#9166,.T.);
#12589=ORIENTED_EDGE('',*,*,#9167,.F.);
#12590=ORIENTED_EDGE('',*,*,#9168,.F.);
#12591=ORIENTED_EDGE('',*,*,#8329,.T.);
#12592=ORIENTED_EDGE('',*,*,#9169,.F.);
#12593=ORIENTED_EDGE('',*,*,#9162,.F.);
#12594=ORIENTED_EDGE('',*,*,#9170,.F.);
#12595=ORIENTED_EDGE('',*,*,#9171,.F.);
#12596=ORIENTED_EDGE('',*,*,#9166,.F.);
#12597=ORIENTED_EDGE('',*,*,#9172,.T.);
#12598=ORIENTED_EDGE('',*,*,#9173,.F.);
#12599=ORIENTED_EDGE('',*,*,#9174,.T.);
#12600=ORIENTED_EDGE('',*,*,#9175,.T.);
#12601=ORIENTED_EDGE('',*,*,#9043,.F.);
#12602=ORIENTED_EDGE('',*,*,#9051,.T.);
#12603=ORIENTED_EDGE('',*,*,#8331,.T.);
#12604=ORIENTED_EDGE('',*,*,#9176,.T.);
#12605=ORIENTED_EDGE('',*,*,#9175,.F.);
#12606=ORIENTED_EDGE('',*,*,#9177,.T.);
#12607=ORIENTED_EDGE('',*,*,#9056,.F.);
#12608=ORIENTED_EDGE('',*,*,#9178,.T.);
#12609=ORIENTED_EDGE('',*,*,#9057,.F.);
#12610=ORIENTED_EDGE('',*,*,#9065,.T.);
#12611=ORIENTED_EDGE('',*,*,#8333,.T.);
#12612=ORIENTED_EDGE('',*,*,#9050,.F.);
#12613=ORIENTED_EDGE('',*,*,#9070,.F.);
#12614=ORIENTED_EDGE('',*,*,#9179,.T.);
#12615=ORIENTED_EDGE('',*,*,#9071,.F.);
#12616=ORIENTED_EDGE('',*,*,#9079,.T.);
#12617=ORIENTED_EDGE('',*,*,#8335,.T.);
#12618=ORIENTED_EDGE('',*,*,#9064,.F.);
#12619=ORIENTED_EDGE('',*,*,#9084,.F.);
#12620=ORIENTED_EDGE('',*,*,#9180,.T.);
#12621=ORIENTED_EDGE('',*,*,#9085,.F.);
#12622=ORIENTED_EDGE('',*,*,#9093,.T.);
#12623=ORIENTED_EDGE('',*,*,#8337,.T.);
#12624=ORIENTED_EDGE('',*,*,#9078,.F.);
#12625=ORIENTED_EDGE('',*,*,#9098,.F.);
#12626=ORIENTED_EDGE('',*,*,#9181,.T.);
#12627=ORIENTED_EDGE('',*,*,#9099,.F.);
#12628=ORIENTED_EDGE('',*,*,#9107,.T.);
#12629=ORIENTED_EDGE('',*,*,#8339,.T.);
#12630=ORIENTED_EDGE('',*,*,#9092,.F.);
#12631=ORIENTED_EDGE('',*,*,#9112,.F.);
#12632=ORIENTED_EDGE('',*,*,#9182,.T.);
#12633=ORIENTED_EDGE('',*,*,#9113,.F.);
#12634=ORIENTED_EDGE('',*,*,#9121,.T.);
#12635=ORIENTED_EDGE('',*,*,#8341,.T.);
#12636=ORIENTED_EDGE('',*,*,#9106,.F.);
#12637=ORIENTED_EDGE('',*,*,#9126,.F.);
#12638=ORIENTED_EDGE('',*,*,#9183,.T.);
#12639=ORIENTED_EDGE('',*,*,#9127,.F.);
#12640=ORIENTED_EDGE('',*,*,#9135,.T.);
#12641=ORIENTED_EDGE('',*,*,#8343,.T.);
#12642=ORIENTED_EDGE('',*,*,#9120,.F.);
#12643=ORIENTED_EDGE('',*,*,#9125,.F.);
#12644=ORIENTED_EDGE('',*,*,#9184,.F.);
#12645=ORIENTED_EDGE('',*,*,#9128,.F.);
#12646=ORIENTED_EDGE('',*,*,#9183,.F.);
#12647=ORIENTED_EDGE('',*,*,#9111,.F.);
#12648=ORIENTED_EDGE('',*,*,#9185,.F.);
#12649=ORIENTED_EDGE('',*,*,#9114,.F.);
#12650=ORIENTED_EDGE('',*,*,#9182,.F.);
#12651=ORIENTED_EDGE('',*,*,#9097,.F.);
#12652=ORIENTED_EDGE('',*,*,#9186,.F.);
#12653=ORIENTED_EDGE('',*,*,#9100,.F.);
#12654=ORIENTED_EDGE('',*,*,#9181,.F.);
#12655=ORIENTED_EDGE('',*,*,#9083,.F.);
#12656=ORIENTED_EDGE('',*,*,#9187,.F.);
#12657=ORIENTED_EDGE('',*,*,#9086,.F.);
#12658=ORIENTED_EDGE('',*,*,#9180,.F.);
#12659=ORIENTED_EDGE('',*,*,#9069,.F.);
#12660=ORIENTED_EDGE('',*,*,#9188,.F.);
#12661=ORIENTED_EDGE('',*,*,#9072,.F.);
#12662=ORIENTED_EDGE('',*,*,#9179,.F.);
#12663=ORIENTED_EDGE('',*,*,#9055,.F.);
#12664=ORIENTED_EDGE('',*,*,#9189,.F.);
#12665=ORIENTED_EDGE('',*,*,#9058,.F.);
#12666=ORIENTED_EDGE('',*,*,#9178,.F.);
#12667=ORIENTED_EDGE('',*,*,#9044,.F.);
#12668=ORIENTED_EDGE('',*,*,#9177,.F.);
#12669=ORIENTED_EDGE('',*,*,#9174,.F.);
#12670=ORIENTED_EDGE('',*,*,#9190,.F.);
#12671=ORIENTED_EDGE('',*,*,#9167,.T.);
#12672=ORIENTED_EDGE('',*,*,#9171,.T.);
#12673=ORIENTED_EDGE('',*,*,#9191,.T.);
#12674=ORIENTED_EDGE('',*,*,#9192,.T.);
#12675=ORIENTED_EDGE('',*,*,#9160,.F.);
#12676=ORIENTED_EDGE('',*,*,#9193,.T.);
#12677=ORIENTED_EDGE('',*,*,#9164,.F.);
#12678=ORIENTED_EDGE('',*,*,#9169,.T.);
#12679=ORIENTED_EDGE('',*,*,#8328,.T.);
#12680=ORIENTED_EDGE('',*,*,#9154,.F.);
#12681=ORIENTED_EDGE('',*,*,#9176,.F.);
#12682=ORIENTED_EDGE('',*,*,#8330,.F.);
#12683=ORIENTED_EDGE('',*,*,#9168,.T.);
#12684=ORIENTED_EDGE('',*,*,#9192,.F.);
#12685=ORIENTED_EDGE('',*,*,#9194,.T.);
#12686=ORIENTED_EDGE('',*,*,#9172,.F.);
#12687=ORIENTED_EDGE('',*,*,#9159,.F.);
#12688=ORIENTED_EDGE('',*,*,#9195,.T.);
#12689=ORIENTED_EDGE('',*,*,#9165,.F.);
#12690=ORIENTED_EDGE('',*,*,#9193,.F.);
#12691=ORIENTED_EDGE('',*,*,#9196,.T.);
#12692=ORIENTED_EDGE('',*,*,#9197,.T.);
#12693=ORIENTED_EDGE('',*,*,#9198,.T.);
#12694=ORIENTED_EDGE('',*,*,#9199,.T.);
#12695=ORIENTED_EDGE('',*,*,#9200,.T.);
#12696=ORIENTED_EDGE('',*,*,#9200,.F.);
#12697=ORIENTED_EDGE('',*,*,#9201,.T.);
#12698=ORIENTED_EDGE('',*,*,#9202,.F.);
#12699=ORIENTED_EDGE('',*,*,#9203,.T.);
#12700=ORIENTED_EDGE('',*,*,#8310,.T.);
#12701=ORIENTED_EDGE('',*,*,#9204,.F.);
#12702=ORIENTED_EDGE('',*,*,#9199,.F.);
#12703=ORIENTED_EDGE('',*,*,#9205,.T.);
#12704=ORIENTED_EDGE('',*,*,#9206,.F.);
#12705=ORIENTED_EDGE('',*,*,#9201,.F.);
#12706=ORIENTED_EDGE('',*,*,#9207,.F.);
#12707=ORIENTED_EDGE('',*,*,#9208,.T.);
#12708=ORIENTED_EDGE('',*,*,#9209,.T.);
#12709=ORIENTED_EDGE('',*,*,#9202,.T.);
#12710=ORIENTED_EDGE('',*,*,#9206,.T.);
#12711=ORIENTED_EDGE('',*,*,#9210,.T.);
#12712=ORIENTED_EDGE('',*,*,#9211,.T.);
#12713=ORIENTED_EDGE('',*,*,#9212,.T.);
#12714=ORIENTED_EDGE('',*,*,#9213,.T.);
#12715=ORIENTED_EDGE('',*,*,#9214,.T.);
#12716=ORIENTED_EDGE('',*,*,#9214,.F.);
#12717=ORIENTED_EDGE('',*,*,#9215,.T.);
#12718=ORIENTED_EDGE('',*,*,#9216,.F.);
#12719=ORIENTED_EDGE('',*,*,#9217,.T.);
#12720=ORIENTED_EDGE('',*,*,#8312,.T.);
#12721=ORIENTED_EDGE('',*,*,#9218,.F.);
#12722=ORIENTED_EDGE('',*,*,#9213,.F.);
#12723=ORIENTED_EDGE('',*,*,#9219,.T.);
#12724=ORIENTED_EDGE('',*,*,#9220,.F.);
#12725=ORIENTED_EDGE('',*,*,#9215,.F.);
#12726=ORIENTED_EDGE('',*,*,#9221,.F.);
#12727=ORIENTED_EDGE('',*,*,#9222,.T.);
#12728=ORIENTED_EDGE('',*,*,#9223,.T.);
#12729=ORIENTED_EDGE('',*,*,#9216,.T.);
#12730=ORIENTED_EDGE('',*,*,#9220,.T.);
#12731=ORIENTED_EDGE('',*,*,#9224,.T.);
#12732=ORIENTED_EDGE('',*,*,#9225,.T.);
#12733=ORIENTED_EDGE('',*,*,#9226,.T.);
#12734=ORIENTED_EDGE('',*,*,#9227,.T.);
#12735=ORIENTED_EDGE('',*,*,#9228,.T.);
#12736=ORIENTED_EDGE('',*,*,#9228,.F.);
#12737=ORIENTED_EDGE('',*,*,#9229,.T.);
#12738=ORIENTED_EDGE('',*,*,#9230,.F.);
#12739=ORIENTED_EDGE('',*,*,#9231,.T.);
#12740=ORIENTED_EDGE('',*,*,#8314,.T.);
#12741=ORIENTED_EDGE('',*,*,#9232,.F.);
#12742=ORIENTED_EDGE('',*,*,#9227,.F.);
#12743=ORIENTED_EDGE('',*,*,#9233,.T.);
#12744=ORIENTED_EDGE('',*,*,#9234,.F.);
#12745=ORIENTED_EDGE('',*,*,#9229,.F.);
#12746=ORIENTED_EDGE('',*,*,#9235,.F.);
#12747=ORIENTED_EDGE('',*,*,#9236,.T.);
#12748=ORIENTED_EDGE('',*,*,#9237,.T.);
#12749=ORIENTED_EDGE('',*,*,#9230,.T.);
#12750=ORIENTED_EDGE('',*,*,#9234,.T.);
#12751=ORIENTED_EDGE('',*,*,#9238,.T.);
#12752=ORIENTED_EDGE('',*,*,#9239,.T.);
#12753=ORIENTED_EDGE('',*,*,#9240,.T.);
#12754=ORIENTED_EDGE('',*,*,#9241,.T.);
#12755=ORIENTED_EDGE('',*,*,#9242,.T.);
#12756=ORIENTED_EDGE('',*,*,#9242,.F.);
#12757=ORIENTED_EDGE('',*,*,#9243,.T.);
#12758=ORIENTED_EDGE('',*,*,#9244,.F.);
#12759=ORIENTED_EDGE('',*,*,#9245,.T.);
#12760=ORIENTED_EDGE('',*,*,#8316,.T.);
#12761=ORIENTED_EDGE('',*,*,#9246,.F.);
#12762=ORIENTED_EDGE('',*,*,#9241,.F.);
#12763=ORIENTED_EDGE('',*,*,#9247,.T.);
#12764=ORIENTED_EDGE('',*,*,#9248,.F.);
#12765=ORIENTED_EDGE('',*,*,#9243,.F.);
#12766=ORIENTED_EDGE('',*,*,#9249,.F.);
#12767=ORIENTED_EDGE('',*,*,#9250,.T.);
#12768=ORIENTED_EDGE('',*,*,#9251,.T.);
#12769=ORIENTED_EDGE('',*,*,#9244,.T.);
#12770=ORIENTED_EDGE('',*,*,#9248,.T.);
#12771=ORIENTED_EDGE('',*,*,#9252,.T.);
#12772=ORIENTED_EDGE('',*,*,#9253,.T.);
#12773=ORIENTED_EDGE('',*,*,#9254,.T.);
#12774=ORIENTED_EDGE('',*,*,#9255,.T.);
#12775=ORIENTED_EDGE('',*,*,#9256,.T.);
#12776=ORIENTED_EDGE('',*,*,#9256,.F.);
#12777=ORIENTED_EDGE('',*,*,#9257,.T.);
#12778=ORIENTED_EDGE('',*,*,#9258,.F.);
#12779=ORIENTED_EDGE('',*,*,#9259,.T.);
#12780=ORIENTED_EDGE('',*,*,#8318,.T.);
#12781=ORIENTED_EDGE('',*,*,#9260,.F.);
#12782=ORIENTED_EDGE('',*,*,#9255,.F.);
#12783=ORIENTED_EDGE('',*,*,#9261,.T.);
#12784=ORIENTED_EDGE('',*,*,#9262,.F.);
#12785=ORIENTED_EDGE('',*,*,#9257,.F.);
#12786=ORIENTED_EDGE('',*,*,#9263,.F.);
#12787=ORIENTED_EDGE('',*,*,#9264,.T.);
#12788=ORIENTED_EDGE('',*,*,#9265,.T.);
#12789=ORIENTED_EDGE('',*,*,#9258,.T.);
#12790=ORIENTED_EDGE('',*,*,#9262,.T.);
#12791=ORIENTED_EDGE('',*,*,#9266,.T.);
#12792=ORIENTED_EDGE('',*,*,#9267,.T.);
#12793=ORIENTED_EDGE('',*,*,#9268,.T.);
#12794=ORIENTED_EDGE('',*,*,#9269,.T.);
#12795=ORIENTED_EDGE('',*,*,#9270,.T.);
#12796=ORIENTED_EDGE('',*,*,#9270,.F.);
#12797=ORIENTED_EDGE('',*,*,#9271,.T.);
#12798=ORIENTED_EDGE('',*,*,#9272,.F.);
#12799=ORIENTED_EDGE('',*,*,#9273,.T.);
#12800=ORIENTED_EDGE('',*,*,#8320,.T.);
#12801=ORIENTED_EDGE('',*,*,#9274,.F.);
#12802=ORIENTED_EDGE('',*,*,#9269,.F.);
#12803=ORIENTED_EDGE('',*,*,#9275,.T.);
#12804=ORIENTED_EDGE('',*,*,#9276,.F.);
#12805=ORIENTED_EDGE('',*,*,#9271,.F.);
#12806=ORIENTED_EDGE('',*,*,#9277,.F.);
#12807=ORIENTED_EDGE('',*,*,#9278,.T.);
#12808=ORIENTED_EDGE('',*,*,#9279,.T.);
#12809=ORIENTED_EDGE('',*,*,#9272,.T.);
#12810=ORIENTED_EDGE('',*,*,#9276,.T.);
#12811=ORIENTED_EDGE('',*,*,#9280,.T.);
#12812=ORIENTED_EDGE('',*,*,#9281,.T.);
#12813=ORIENTED_EDGE('',*,*,#9282,.T.);
#12814=ORIENTED_EDGE('',*,*,#9283,.T.);
#12815=ORIENTED_EDGE('',*,*,#9284,.T.);
#12816=ORIENTED_EDGE('',*,*,#9284,.F.);
#12817=ORIENTED_EDGE('',*,*,#9285,.T.);
#12818=ORIENTED_EDGE('',*,*,#9286,.F.);
#12819=ORIENTED_EDGE('',*,*,#9287,.T.);
#12820=ORIENTED_EDGE('',*,*,#8322,.T.);
#12821=ORIENTED_EDGE('',*,*,#9288,.F.);
#12822=ORIENTED_EDGE('',*,*,#9283,.F.);
#12823=ORIENTED_EDGE('',*,*,#9289,.T.);
#12824=ORIENTED_EDGE('',*,*,#9290,.F.);
#12825=ORIENTED_EDGE('',*,*,#9285,.F.);
#12826=ORIENTED_EDGE('',*,*,#9291,.F.);
#12827=ORIENTED_EDGE('',*,*,#9292,.T.);
#12828=ORIENTED_EDGE('',*,*,#9293,.T.);
#12829=ORIENTED_EDGE('',*,*,#9286,.T.);
#12830=ORIENTED_EDGE('',*,*,#9290,.T.);
#12831=ORIENTED_EDGE('',*,*,#9294,.T.);
#12832=ORIENTED_EDGE('',*,*,#9295,.T.);
#12833=ORIENTED_EDGE('',*,*,#9296,.T.);
#12834=ORIENTED_EDGE('',*,*,#9297,.T.);
#12835=ORIENTED_EDGE('',*,*,#9298,.T.);
#12836=ORIENTED_EDGE('',*,*,#9298,.F.);
#12837=ORIENTED_EDGE('',*,*,#9299,.T.);
#12838=ORIENTED_EDGE('',*,*,#9300,.F.);
#12839=ORIENTED_EDGE('',*,*,#9301,.T.);
#12840=ORIENTED_EDGE('',*,*,#8324,.T.);
#12841=ORIENTED_EDGE('',*,*,#9302,.F.);
#12842=ORIENTED_EDGE('',*,*,#9297,.F.);
#12843=ORIENTED_EDGE('',*,*,#9303,.T.);
#12844=ORIENTED_EDGE('',*,*,#9304,.F.);
#12845=ORIENTED_EDGE('',*,*,#9299,.F.);
#12846=ORIENTED_EDGE('',*,*,#9305,.T.);
#12847=ORIENTED_EDGE('',*,*,#9306,.T.);
#12848=ORIENTED_EDGE('',*,*,#9307,.T.);
#12849=ORIENTED_EDGE('',*,*,#9308,.T.);
#12850=ORIENTED_EDGE('',*,*,#9306,.F.);
#12851=ORIENTED_EDGE('',*,*,#9309,.F.);
#12852=ORIENTED_EDGE('',*,*,#9310,.F.);
#12853=ORIENTED_EDGE('',*,*,#9311,.F.);
#12854=ORIENTED_EDGE('',*,*,#9305,.F.);
#12855=ORIENTED_EDGE('',*,*,#9312,.F.);
#12856=ORIENTED_EDGE('',*,*,#8325,.T.);
#12857=ORIENTED_EDGE('',*,*,#9301,.F.);
#12858=ORIENTED_EDGE('',*,*,#9313,.F.);
#12859=ORIENTED_EDGE('',*,*,#9309,.T.);
#12860=ORIENTED_EDGE('',*,*,#9314,.F.);
#12861=ORIENTED_EDGE('',*,*,#9310,.T.);
#12862=ORIENTED_EDGE('',*,*,#9313,.T.);
#12863=ORIENTED_EDGE('',*,*,#9300,.T.);
#12864=ORIENTED_EDGE('',*,*,#9304,.T.);
#12865=ORIENTED_EDGE('',*,*,#9315,.F.);
#12866=ORIENTED_EDGE('',*,*,#9316,.T.);
#12867=ORIENTED_EDGE('',*,*,#9317,.T.);
#12868=ORIENTED_EDGE('',*,*,#9318,.T.);
#12869=ORIENTED_EDGE('',*,*,#9317,.F.);
#12870=ORIENTED_EDGE('',*,*,#9319,.T.);
#12871=ORIENTED_EDGE('',*,*,#9320,.F.);
#12872=ORIENTED_EDGE('',*,*,#9321,.F.);
#12873=ORIENTED_EDGE('',*,*,#8307,.T.);
#12874=ORIENTED_EDGE('',*,*,#9322,.F.);
#12875=ORIENTED_EDGE('',*,*,#9316,.F.);
#12876=ORIENTED_EDGE('',*,*,#9323,.F.);
#12877=ORIENTED_EDGE('',*,*,#9324,.F.);
#12878=ORIENTED_EDGE('',*,*,#9319,.F.);
#12879=ORIENTED_EDGE('',*,*,#9325,.T.);
#12880=ORIENTED_EDGE('',*,*,#9326,.F.);
#12881=ORIENTED_EDGE('',*,*,#9327,.T.);
#12882=ORIENTED_EDGE('',*,*,#9328,.T.);
#12883=ORIENTED_EDGE('',*,*,#9196,.F.);
#12884=ORIENTED_EDGE('',*,*,#9204,.T.);
#12885=ORIENTED_EDGE('',*,*,#8309,.T.);
#12886=ORIENTED_EDGE('',*,*,#9329,.T.);
#12887=ORIENTED_EDGE('',*,*,#9328,.F.);
#12888=ORIENTED_EDGE('',*,*,#9330,.T.);
#12889=ORIENTED_EDGE('',*,*,#9209,.F.);
#12890=ORIENTED_EDGE('',*,*,#9331,.T.);
#12891=ORIENTED_EDGE('',*,*,#9210,.F.);
#12892=ORIENTED_EDGE('',*,*,#9218,.T.);
#12893=ORIENTED_EDGE('',*,*,#8311,.T.);
#12894=ORIENTED_EDGE('',*,*,#9203,.F.);
#12895=ORIENTED_EDGE('',*,*,#9223,.F.);
#12896=ORIENTED_EDGE('',*,*,#9332,.T.);
#12897=ORIENTED_EDGE('',*,*,#9224,.F.);
#12898=ORIENTED_EDGE('',*,*,#9232,.T.);
#12899=ORIENTED_EDGE('',*,*,#8313,.T.);
#12900=ORIENTED_EDGE('',*,*,#9217,.F.);
#12901=ORIENTED_EDGE('',*,*,#9237,.F.);
#12902=ORIENTED_EDGE('',*,*,#9333,.T.);
#12903=ORIENTED_EDGE('',*,*,#9238,.F.);
#12904=ORIENTED_EDGE('',*,*,#9246,.T.);
#12905=ORIENTED_EDGE('',*,*,#8315,.T.);
#12906=ORIENTED_EDGE('',*,*,#9231,.F.);
#12907=ORIENTED_EDGE('',*,*,#9251,.F.);
#12908=ORIENTED_EDGE('',*,*,#9334,.T.);
#12909=ORIENTED_EDGE('',*,*,#9252,.F.);
#12910=ORIENTED_EDGE('',*,*,#9260,.T.);
#12911=ORIENTED_EDGE('',*,*,#8317,.T.);
#12912=ORIENTED_EDGE('',*,*,#9245,.F.);
#12913=ORIENTED_EDGE('',*,*,#9265,.F.);
#12914=ORIENTED_EDGE('',*,*,#9335,.T.);
#12915=ORIENTED_EDGE('',*,*,#9266,.F.);
#12916=ORIENTED_EDGE('',*,*,#9274,.T.);
#12917=ORIENTED_EDGE('',*,*,#8319,.T.);
#12918=ORIENTED_EDGE('',*,*,#9259,.F.);
#12919=ORIENTED_EDGE('',*,*,#9279,.F.);
#12920=ORIENTED_EDGE('',*,*,#9336,.T.);
#12921=ORIENTED_EDGE('',*,*,#9280,.F.);
#12922=ORIENTED_EDGE('',*,*,#9288,.T.);
#12923=ORIENTED_EDGE('',*,*,#8321,.T.);
#12924=ORIENTED_EDGE('',*,*,#9273,.F.);
#12925=ORIENTED_EDGE('',*,*,#9293,.F.);
#12926=ORIENTED_EDGE('',*,*,#9337,.T.);
#12927=ORIENTED_EDGE('',*,*,#9294,.F.);
#12928=ORIENTED_EDGE('',*,*,#9302,.T.);
#12929=ORIENTED_EDGE('',*,*,#8323,.T.);
#12930=ORIENTED_EDGE('',*,*,#9287,.F.);
#12931=ORIENTED_EDGE('',*,*,#9292,.F.);
#12932=ORIENTED_EDGE('',*,*,#9338,.F.);
#12933=ORIENTED_EDGE('',*,*,#9295,.F.);
#12934=ORIENTED_EDGE('',*,*,#9337,.F.);
#12935=ORIENTED_EDGE('',*,*,#9278,.F.);
#12936=ORIENTED_EDGE('',*,*,#9339,.F.);
#12937=ORIENTED_EDGE('',*,*,#9281,.F.);
#12938=ORIENTED_EDGE('',*,*,#9336,.F.);
#12939=ORIENTED_EDGE('',*,*,#9264,.F.);
#12940=ORIENTED_EDGE('',*,*,#9340,.F.);
#12941=ORIENTED_EDGE('',*,*,#9267,.F.);
#12942=ORIENTED_EDGE('',*,*,#9335,.F.);
#12943=ORIENTED_EDGE('',*,*,#9250,.F.);
#12944=ORIENTED_EDGE('',*,*,#9341,.F.);
#12945=ORIENTED_EDGE('',*,*,#9253,.F.);
#12946=ORIENTED_EDGE('',*,*,#9334,.F.);
#12947=ORIENTED_EDGE('',*,*,#9236,.F.);
#12948=ORIENTED_EDGE('',*,*,#9342,.F.);
#12949=ORIENTED_EDGE('',*,*,#9239,.F.);
#12950=ORIENTED_EDGE('',*,*,#9333,.F.);
#12951=ORIENTED_EDGE('',*,*,#9222,.F.);
#12952=ORIENTED_EDGE('',*,*,#9343,.F.);
#12953=ORIENTED_EDGE('',*,*,#9225,.F.);
#12954=ORIENTED_EDGE('',*,*,#9332,.F.);
#12955=ORIENTED_EDGE('',*,*,#9208,.F.);
#12956=ORIENTED_EDGE('',*,*,#9344,.F.);
#12957=ORIENTED_EDGE('',*,*,#9211,.F.);
#12958=ORIENTED_EDGE('',*,*,#9331,.F.);
#12959=ORIENTED_EDGE('',*,*,#9197,.F.);
#12960=ORIENTED_EDGE('',*,*,#9330,.F.);
#12961=ORIENTED_EDGE('',*,*,#9327,.F.);
#12962=ORIENTED_EDGE('',*,*,#9345,.F.);
#12963=ORIENTED_EDGE('',*,*,#9320,.T.);
#12964=ORIENTED_EDGE('',*,*,#9324,.T.);
#12965=ORIENTED_EDGE('',*,*,#9346,.T.);
#12966=ORIENTED_EDGE('',*,*,#9347,.T.);
#12967=ORIENTED_EDGE('',*,*,#9329,.F.);
#12968=ORIENTED_EDGE('',*,*,#8308,.F.);
#12969=ORIENTED_EDGE('',*,*,#9321,.T.);
#12970=ORIENTED_EDGE('',*,*,#9347,.F.);
#12971=ORIENTED_EDGE('',*,*,#9348,.T.);
#12972=ORIENTED_EDGE('',*,*,#9325,.F.);
#12973=ORIENTED_EDGE('',*,*,#9349,.F.);
#12974=ORIENTED_EDGE('',*,*,#9350,.T.);
#12975=ORIENTED_EDGE('',*,*,#9351,.T.);
#12976=ORIENTED_EDGE('',*,*,#8256,.T.);
#12977=ORIENTED_EDGE('',*,*,#9352,.T.);
#12978=ORIENTED_EDGE('',*,*,#9351,.F.);
#12979=ORIENTED_EDGE('',*,*,#9353,.T.);
#12980=ORIENTED_EDGE('',*,*,#9354,.F.);
#12981=ORIENTED_EDGE('',*,*,#9355,.T.);
#12982=ORIENTED_EDGE('',*,*,#8288,.T.);
#12983=ORIENTED_EDGE('',*,*,#8257,.T.);
#12984=ORIENTED_EDGE('',*,*,#9350,.F.);
#12985=ORIENTED_EDGE('',*,*,#9356,.F.);
#12986=ORIENTED_EDGE('',*,*,#9357,.F.);
#12987=ORIENTED_EDGE('',*,*,#9353,.F.);
#12988=ORIENTED_EDGE('',*,*,#9354,.T.);
#12989=ORIENTED_EDGE('',*,*,#9357,.T.);
#12990=ORIENTED_EDGE('',*,*,#9358,.T.);
#12991=ORIENTED_EDGE('',*,*,#9359,.T.);
#12992=ORIENTED_EDGE('',*,*,#9360,.T.);
#12993=ORIENTED_EDGE('',*,*,#9361,.F.);
#12994=ORIENTED_EDGE('',*,*,#9362,.T.);
#12995=ORIENTED_EDGE('',*,*,#9363,.T.);
#12996=ORIENTED_EDGE('',*,*,#9364,.T.);
#12997=ORIENTED_EDGE('',*,*,#9365,.T.);
#12998=ORIENTED_EDGE('',*,*,#9363,.F.);
#12999=ORIENTED_EDGE('',*,*,#9366,.T.);
#13000=ORIENTED_EDGE('',*,*,#9367,.F.);
#13001=ORIENTED_EDGE('',*,*,#9368,.T.);
#13002=ORIENTED_EDGE('',*,*,#8290,.T.);
#13003=ORIENTED_EDGE('',*,*,#9369,.F.);
#13004=ORIENTED_EDGE('',*,*,#9362,.F.);
#13005=ORIENTED_EDGE('',*,*,#9370,.F.);
#13006=ORIENTED_EDGE('',*,*,#9371,.F.);
#13007=ORIENTED_EDGE('',*,*,#9366,.F.);
#13008=ORIENTED_EDGE('',*,*,#9367,.T.);
#13009=ORIENTED_EDGE('',*,*,#9371,.T.);
#13010=ORIENTED_EDGE('',*,*,#9372,.T.);
#13011=ORIENTED_EDGE('',*,*,#9373,.T.);
#13012=ORIENTED_EDGE('',*,*,#9374,.T.);
#13013=ORIENTED_EDGE('',*,*,#9375,.F.);
#13014=ORIENTED_EDGE('',*,*,#9376,.T.);
#13015=ORIENTED_EDGE('',*,*,#9377,.T.);
#13016=ORIENTED_EDGE('',*,*,#9378,.T.);
#13017=ORIENTED_EDGE('',*,*,#9379,.T.);
#13018=ORIENTED_EDGE('',*,*,#9377,.F.);
#13019=ORIENTED_EDGE('',*,*,#9380,.T.);
#13020=ORIENTED_EDGE('',*,*,#9381,.F.);
#13021=ORIENTED_EDGE('',*,*,#9382,.T.);
#13022=ORIENTED_EDGE('',*,*,#8292,.T.);
#13023=ORIENTED_EDGE('',*,*,#9383,.F.);
#13024=ORIENTED_EDGE('',*,*,#9376,.F.);
#13025=ORIENTED_EDGE('',*,*,#9384,.F.);
#13026=ORIENTED_EDGE('',*,*,#9385,.F.);
#13027=ORIENTED_EDGE('',*,*,#9380,.F.);
#13028=ORIENTED_EDGE('',*,*,#9381,.T.);
#13029=ORIENTED_EDGE('',*,*,#9385,.T.);
#13030=ORIENTED_EDGE('',*,*,#9386,.T.);
#13031=ORIENTED_EDGE('',*,*,#9387,.T.);
#13032=ORIENTED_EDGE('',*,*,#9388,.T.);
#13033=ORIENTED_EDGE('',*,*,#9389,.F.);
#13034=ORIENTED_EDGE('',*,*,#9390,.T.);
#13035=ORIENTED_EDGE('',*,*,#9391,.T.);
#13036=ORIENTED_EDGE('',*,*,#9392,.T.);
#13037=ORIENTED_EDGE('',*,*,#9393,.T.);
#13038=ORIENTED_EDGE('',*,*,#9391,.F.);
#13039=ORIENTED_EDGE('',*,*,#9394,.T.);
#13040=ORIENTED_EDGE('',*,*,#9395,.F.);
#13041=ORIENTED_EDGE('',*,*,#9396,.T.);
#13042=ORIENTED_EDGE('',*,*,#8294,.T.);
#13043=ORIENTED_EDGE('',*,*,#9397,.F.);
#13044=ORIENTED_EDGE('',*,*,#9390,.F.);
#13045=ORIENTED_EDGE('',*,*,#9398,.F.);
#13046=ORIENTED_EDGE('',*,*,#9399,.F.);
#13047=ORIENTED_EDGE('',*,*,#9394,.F.);
#13048=ORIENTED_EDGE('',*,*,#9395,.T.);
#13049=ORIENTED_EDGE('',*,*,#9399,.T.);
#13050=ORIENTED_EDGE('',*,*,#9400,.T.);
#13051=ORIENTED_EDGE('',*,*,#9401,.T.);
#13052=ORIENTED_EDGE('',*,*,#9402,.T.);
#13053=ORIENTED_EDGE('',*,*,#9403,.F.);
#13054=ORIENTED_EDGE('',*,*,#9404,.T.);
#13055=ORIENTED_EDGE('',*,*,#9405,.T.);
#13056=ORIENTED_EDGE('',*,*,#9406,.T.);
#13057=ORIENTED_EDGE('',*,*,#9407,.T.);
#13058=ORIENTED_EDGE('',*,*,#9405,.F.);
#13059=ORIENTED_EDGE('',*,*,#9408,.T.);
#13060=ORIENTED_EDGE('',*,*,#9409,.F.);
#13061=ORIENTED_EDGE('',*,*,#9410,.T.);
#13062=ORIENTED_EDGE('',*,*,#8296,.T.);
#13063=ORIENTED_EDGE('',*,*,#9411,.F.);
#13064=ORIENTED_EDGE('',*,*,#9404,.F.);
#13065=ORIENTED_EDGE('',*,*,#9412,.F.);
#13066=ORIENTED_EDGE('',*,*,#9413,.F.);
#13067=ORIENTED_EDGE('',*,*,#9408,.F.);
#13068=ORIENTED_EDGE('',*,*,#9409,.T.);
#13069=ORIENTED_EDGE('',*,*,#9413,.T.);
#13070=ORIENTED_EDGE('',*,*,#9414,.T.);
#13071=ORIENTED_EDGE('',*,*,#9415,.T.);
#13072=ORIENTED_EDGE('',*,*,#9416,.T.);
#13073=ORIENTED_EDGE('',*,*,#9417,.F.);
#13074=ORIENTED_EDGE('',*,*,#9418,.T.);
#13075=ORIENTED_EDGE('',*,*,#9419,.T.);
#13076=ORIENTED_EDGE('',*,*,#9420,.T.);
#13077=ORIENTED_EDGE('',*,*,#9421,.T.);
#13078=ORIENTED_EDGE('',*,*,#9419,.F.);
#13079=ORIENTED_EDGE('',*,*,#9422,.T.);
#13080=ORIENTED_EDGE('',*,*,#9423,.F.);
#13081=ORIENTED_EDGE('',*,*,#9424,.T.);
#13082=ORIENTED_EDGE('',*,*,#8298,.T.);
#13083=ORIENTED_EDGE('',*,*,#9425,.F.);
#13084=ORIENTED_EDGE('',*,*,#9418,.F.);
#13085=ORIENTED_EDGE('',*,*,#9426,.F.);
#13086=ORIENTED_EDGE('',*,*,#9427,.F.);
#13087=ORIENTED_EDGE('',*,*,#9422,.F.);
#13088=ORIENTED_EDGE('',*,*,#9423,.T.);
#13089=ORIENTED_EDGE('',*,*,#9427,.T.);
#13090=ORIENTED_EDGE('',*,*,#9428,.T.);
#13091=ORIENTED_EDGE('',*,*,#9429,.T.);
#13092=ORIENTED_EDGE('',*,*,#9430,.T.);
#13093=ORIENTED_EDGE('',*,*,#9431,.F.);
#13094=ORIENTED_EDGE('',*,*,#9432,.T.);
#13095=ORIENTED_EDGE('',*,*,#9433,.T.);
#13096=ORIENTED_EDGE('',*,*,#9434,.T.);
#13097=ORIENTED_EDGE('',*,*,#9435,.T.);
#13098=ORIENTED_EDGE('',*,*,#9433,.F.);
#13099=ORIENTED_EDGE('',*,*,#9436,.T.);
#13100=ORIENTED_EDGE('',*,*,#9437,.F.);
#13101=ORIENTED_EDGE('',*,*,#9438,.T.);
#13102=ORIENTED_EDGE('',*,*,#8300,.T.);
#13103=ORIENTED_EDGE('',*,*,#9439,.F.);
#13104=ORIENTED_EDGE('',*,*,#9432,.F.);
#13105=ORIENTED_EDGE('',*,*,#9440,.F.);
#13106=ORIENTED_EDGE('',*,*,#9441,.F.);
#13107=ORIENTED_EDGE('',*,*,#9436,.F.);
#13108=ORIENTED_EDGE('',*,*,#9437,.T.);
#13109=ORIENTED_EDGE('',*,*,#9441,.T.);
#13110=ORIENTED_EDGE('',*,*,#9442,.T.);
#13111=ORIENTED_EDGE('',*,*,#9443,.T.);
#13112=ORIENTED_EDGE('',*,*,#9444,.T.);
#13113=ORIENTED_EDGE('',*,*,#9445,.F.);
#13114=ORIENTED_EDGE('',*,*,#9446,.T.);
#13115=ORIENTED_EDGE('',*,*,#9447,.T.);
#13116=ORIENTED_EDGE('',*,*,#9448,.T.);
#13117=ORIENTED_EDGE('',*,*,#9449,.T.);
#13118=ORIENTED_EDGE('',*,*,#9447,.F.);
#13119=ORIENTED_EDGE('',*,*,#9450,.T.);
#13120=ORIENTED_EDGE('',*,*,#9451,.F.);
#13121=ORIENTED_EDGE('',*,*,#9452,.T.);
#13122=ORIENTED_EDGE('',*,*,#8302,.T.);
#13123=ORIENTED_EDGE('',*,*,#9453,.F.);
#13124=ORIENTED_EDGE('',*,*,#9446,.F.);
#13125=ORIENTED_EDGE('',*,*,#9454,.F.);
#13126=ORIENTED_EDGE('',*,*,#9455,.F.);
#13127=ORIENTED_EDGE('',*,*,#9450,.F.);
#13128=ORIENTED_EDGE('',*,*,#9451,.T.);
#13129=ORIENTED_EDGE('',*,*,#9455,.T.);
#13130=ORIENTED_EDGE('',*,*,#9456,.T.);
#13131=ORIENTED_EDGE('',*,*,#9457,.T.);
#13132=ORIENTED_EDGE('',*,*,#9458,.T.);
#13133=ORIENTED_EDGE('',*,*,#9459,.F.);
#13134=ORIENTED_EDGE('',*,*,#9460,.T.);
#13135=ORIENTED_EDGE('',*,*,#9461,.T.);
#13136=ORIENTED_EDGE('',*,*,#9462,.T.);
#13137=ORIENTED_EDGE('',*,*,#9463,.T.);
#13138=ORIENTED_EDGE('',*,*,#9461,.F.);
#13139=ORIENTED_EDGE('',*,*,#9464,.T.);
#13140=ORIENTED_EDGE('',*,*,#9465,.F.);
#13141=ORIENTED_EDGE('',*,*,#9466,.T.);
#13142=ORIENTED_EDGE('',*,*,#8304,.T.);
#13143=ORIENTED_EDGE('',*,*,#9467,.F.);
#13144=ORIENTED_EDGE('',*,*,#9460,.F.);
#13145=ORIENTED_EDGE('',*,*,#9468,.F.);
#13146=ORIENTED_EDGE('',*,*,#9469,.F.);
#13147=ORIENTED_EDGE('',*,*,#9464,.F.);
#13148=ORIENTED_EDGE('',*,*,#9470,.F.);
#13149=ORIENTED_EDGE('',*,*,#8047,.T.);
#13150=ORIENTED_EDGE('',*,*,#8052,.T.);
#13151=ORIENTED_EDGE('',*,*,#9471,.T.);
#13152=ORIENTED_EDGE('',*,*,#9472,.T.);
#13153=ORIENTED_EDGE('',*,*,#9472,.F.);
#13154=ORIENTED_EDGE('',*,*,#9473,.F.);
#13155=ORIENTED_EDGE('',*,*,#9474,.F.);
#13156=ORIENTED_EDGE('',*,*,#9475,.T.);
#13157=ORIENTED_EDGE('',*,*,#9471,.F.);
#13158=ORIENTED_EDGE('',*,*,#8051,.F.);
#13159=ORIENTED_EDGE('',*,*,#8305,.T.);
#13160=ORIENTED_EDGE('',*,*,#9466,.F.);
#13161=ORIENTED_EDGE('',*,*,#9476,.F.);
#13162=ORIENTED_EDGE('',*,*,#9473,.T.);
#13163=ORIENTED_EDGE('',*,*,#9465,.T.);
#13164=ORIENTED_EDGE('',*,*,#9469,.T.);
#13165=ORIENTED_EDGE('',*,*,#9477,.T.);
#13166=ORIENTED_EDGE('',*,*,#9474,.T.);
#13167=ORIENTED_EDGE('',*,*,#9476,.T.);
#13168=ORIENTED_EDGE('',*,*,#9360,.F.);
#13169=ORIENTED_EDGE('',*,*,#9478,.T.);
#13170=ORIENTED_EDGE('',*,*,#9364,.F.);
#13171=ORIENTED_EDGE('',*,*,#9369,.T.);
#13172=ORIENTED_EDGE('',*,*,#8289,.T.);
#13173=ORIENTED_EDGE('',*,*,#9355,.F.);
#13174=ORIENTED_EDGE('',*,*,#9374,.F.);
#13175=ORIENTED_EDGE('',*,*,#9479,.T.);
#13176=ORIENTED_EDGE('',*,*,#9378,.F.);
#13177=ORIENTED_EDGE('',*,*,#9383,.T.);
#13178=ORIENTED_EDGE('',*,*,#8291,.T.);
#13179=ORIENTED_EDGE('',*,*,#9368,.F.);
#13180=ORIENTED_EDGE('',*,*,#9388,.F.);
#13181=ORIENTED_EDGE('',*,*,#9480,.T.);
#13182=ORIENTED_EDGE('',*,*,#9392,.F.);
#13183=ORIENTED_EDGE('',*,*,#9397,.T.);
#13184=ORIENTED_EDGE('',*,*,#8293,.T.);
#13185=ORIENTED_EDGE('',*,*,#9382,.F.);
#13186=ORIENTED_EDGE('',*,*,#9402,.F.);
#13187=ORIENTED_EDGE('',*,*,#9481,.T.);
#13188=ORIENTED_EDGE('',*,*,#9406,.F.);
#13189=ORIENTED_EDGE('',*,*,#9411,.T.);
#13190=ORIENTED_EDGE('',*,*,#8295,.T.);
#13191=ORIENTED_EDGE('',*,*,#9396,.F.);
#13192=ORIENTED_EDGE('',*,*,#9416,.F.);
#13193=ORIENTED_EDGE('',*,*,#9482,.T.);
#13194=ORIENTED_EDGE('',*,*,#9420,.F.);
#13195=ORIENTED_EDGE('',*,*,#9425,.T.);
#13196=ORIENTED_EDGE('',*,*,#8297,.T.);
#13197=ORIENTED_EDGE('',*,*,#9410,.F.);
#13198=ORIENTED_EDGE('',*,*,#9430,.F.);
#13199=ORIENTED_EDGE('',*,*,#9483,.T.);
#13200=ORIENTED_EDGE('',*,*,#9434,.F.);
#13201=ORIENTED_EDGE('',*,*,#9439,.T.);
#13202=ORIENTED_EDGE('',*,*,#8299,.T.);
#13203=ORIENTED_EDGE('',*,*,#9424,.F.);
#13204=ORIENTED_EDGE('',*,*,#9444,.F.);
#13205=ORIENTED_EDGE('',*,*,#9484,.T.);
#13206=ORIENTED_EDGE('',*,*,#9448,.F.);
#13207=ORIENTED_EDGE('',*,*,#9453,.T.);
#13208=ORIENTED_EDGE('',*,*,#8301,.T.);
#13209=ORIENTED_EDGE('',*,*,#9438,.F.);
#13210=ORIENTED_EDGE('',*,*,#9458,.F.);
#13211=ORIENTED_EDGE('',*,*,#9485,.T.);
#13212=ORIENTED_EDGE('',*,*,#9462,.F.);
#13213=ORIENTED_EDGE('',*,*,#9467,.T.);
#13214=ORIENTED_EDGE('',*,*,#8303,.T.);
#13215=ORIENTED_EDGE('',*,*,#9452,.F.);
#13216=ORIENTED_EDGE('',*,*,#9457,.F.);
#13217=ORIENTED_EDGE('',*,*,#9486,.T.);
#13218=ORIENTED_EDGE('',*,*,#9463,.F.);
#13219=ORIENTED_EDGE('',*,*,#9485,.F.);
#13220=ORIENTED_EDGE('',*,*,#9443,.F.);
#13221=ORIENTED_EDGE('',*,*,#9487,.T.);
#13222=ORIENTED_EDGE('',*,*,#9449,.F.);
#13223=ORIENTED_EDGE('',*,*,#9484,.F.);
#13224=ORIENTED_EDGE('',*,*,#9429,.F.);
#13225=ORIENTED_EDGE('',*,*,#9488,.T.);
#13226=ORIENTED_EDGE('',*,*,#9435,.F.);
#13227=ORIENTED_EDGE('',*,*,#9483,.F.);
#13228=ORIENTED_EDGE('',*,*,#9415,.F.);
#13229=ORIENTED_EDGE('',*,*,#9489,.T.);
#13230=ORIENTED_EDGE('',*,*,#9421,.F.);
#13231=ORIENTED_EDGE('',*,*,#9482,.F.);
#13232=ORIENTED_EDGE('',*,*,#9401,.F.);
#13233=ORIENTED_EDGE('',*,*,#9490,.T.);
#13234=ORIENTED_EDGE('',*,*,#9407,.F.);
#13235=ORIENTED_EDGE('',*,*,#9481,.F.);
#13236=ORIENTED_EDGE('',*,*,#9387,.F.);
#13237=ORIENTED_EDGE('',*,*,#9491,.T.);
#13238=ORIENTED_EDGE('',*,*,#9393,.F.);
#13239=ORIENTED_EDGE('',*,*,#9480,.F.);
#13240=ORIENTED_EDGE('',*,*,#9373,.F.);
#13241=ORIENTED_EDGE('',*,*,#9492,.T.);
#13242=ORIENTED_EDGE('',*,*,#9379,.F.);
#13243=ORIENTED_EDGE('',*,*,#9479,.F.);
#13244=ORIENTED_EDGE('',*,*,#9359,.F.);
#13245=ORIENTED_EDGE('',*,*,#9493,.T.);
#13246=ORIENTED_EDGE('',*,*,#9365,.F.);
#13247=ORIENTED_EDGE('',*,*,#9478,.F.);
#13248=ORIENTED_EDGE('',*,*,#9494,.T.);
#13249=ORIENTED_EDGE('',*,*,#9495,.T.);
#13250=ORIENTED_EDGE('',*,*,#8426,.T.);
#13251=ORIENTED_EDGE('',*,*,#9495,.F.);
#13252=ORIENTED_EDGE('',*,*,#9496,.F.);
#13253=ORIENTED_EDGE('',*,*,#9497,.T.);
#13254=ORIENTED_EDGE('',*,*,#9494,.F.);
#13255=ORIENTED_EDGE('',*,*,#9497,.F.);
#13256=ORIENTED_EDGE('',*,*,#9498,.T.);
#13257=ORIENTED_EDGE('',*,*,#9499,.F.);
#13258=ORIENTED_EDGE('',*,*,#8129,.T.);
#13259=ORIENTED_EDGE('',*,*,#8134,.T.);
#13260=ORIENTED_EDGE('',*,*,#8127,.F.);
#13261=ORIENTED_EDGE('',*,*,#9500,.T.);
#13262=ORIENTED_EDGE('',*,*,#8138,.F.);
#13263=ORIENTED_EDGE('',*,*,#8144,.T.);
#13264=ORIENTED_EDGE('',*,*,#8280,.T.);
#13265=ORIENTED_EDGE('',*,*,#8131,.F.);
#13266=ORIENTED_EDGE('',*,*,#8149,.F.);
#13267=ORIENTED_EDGE('',*,*,#9501,.T.);
#13268=ORIENTED_EDGE('',*,*,#8153,.F.);
#13269=ORIENTED_EDGE('',*,*,#8159,.T.);
#13270=ORIENTED_EDGE('',*,*,#8281,.T.);
#13271=ORIENTED_EDGE('',*,*,#8142,.F.);
#13272=ORIENTED_EDGE('',*,*,#8164,.F.);
#13273=ORIENTED_EDGE('',*,*,#9502,.T.);
#13274=ORIENTED_EDGE('',*,*,#8168,.F.);
#13275=ORIENTED_EDGE('',*,*,#8174,.T.);
#13276=ORIENTED_EDGE('',*,*,#8282,.T.);
#13277=ORIENTED_EDGE('',*,*,#8157,.F.);
#13278=ORIENTED_EDGE('',*,*,#8179,.F.);
#13279=ORIENTED_EDGE('',*,*,#9503,.T.);
#13280=ORIENTED_EDGE('',*,*,#8183,.F.);
#13281=ORIENTED_EDGE('',*,*,#8189,.T.);
#13282=ORIENTED_EDGE('',*,*,#8283,.T.);
#13283=ORIENTED_EDGE('',*,*,#8172,.F.);
#13284=ORIENTED_EDGE('',*,*,#8194,.F.);
#13285=ORIENTED_EDGE('',*,*,#9504,.T.);
#13286=ORIENTED_EDGE('',*,*,#8198,.F.);
#13287=ORIENTED_EDGE('',*,*,#8204,.T.);
#13288=ORIENTED_EDGE('',*,*,#8284,.T.);
#13289=ORIENTED_EDGE('',*,*,#8187,.F.);
#13290=ORIENTED_EDGE('',*,*,#8209,.F.);
#13291=ORIENTED_EDGE('',*,*,#9505,.T.);
#13292=ORIENTED_EDGE('',*,*,#8213,.F.);
#13293=ORIENTED_EDGE('',*,*,#8219,.T.);
#13294=ORIENTED_EDGE('',*,*,#8285,.T.);
#13295=ORIENTED_EDGE('',*,*,#8202,.F.);
#13296=ORIENTED_EDGE('',*,*,#8224,.F.);
#13297=ORIENTED_EDGE('',*,*,#9506,.T.);
#13298=ORIENTED_EDGE('',*,*,#8228,.F.);
#13299=ORIENTED_EDGE('',*,*,#8234,.T.);
#13300=ORIENTED_EDGE('',*,*,#8286,.T.);
#13301=ORIENTED_EDGE('',*,*,#8217,.F.);
#13302=ORIENTED_EDGE('',*,*,#8239,.F.);
#13303=ORIENTED_EDGE('',*,*,#9507,.T.);
#13304=ORIENTED_EDGE('',*,*,#8243,.F.);
#13305=ORIENTED_EDGE('',*,*,#8249,.T.);
#13306=ORIENTED_EDGE('',*,*,#8287,.T.);
#13307=ORIENTED_EDGE('',*,*,#8232,.F.);
#13308=ORIENTED_EDGE('',*,*,#8253,.F.);
#13309=ORIENTED_EDGE('',*,*,#9508,.T.);
#13310=ORIENTED_EDGE('',*,*,#9352,.F.);
#13311=ORIENTED_EDGE('',*,*,#8255,.F.);
#13312=ORIENTED_EDGE('',*,*,#8238,.F.);
#13313=ORIENTED_EDGE('',*,*,#9509,.T.);
#13314=ORIENTED_EDGE('',*,*,#8244,.F.);
#13315=ORIENTED_EDGE('',*,*,#9507,.F.);
#13316=ORIENTED_EDGE('',*,*,#8223,.F.);
#13317=ORIENTED_EDGE('',*,*,#9510,.T.);
#13318=ORIENTED_EDGE('',*,*,#8229,.F.);
#13319=ORIENTED_EDGE('',*,*,#9506,.F.);
#13320=ORIENTED_EDGE('',*,*,#8208,.F.);
#13321=ORIENTED_EDGE('',*,*,#9511,.T.);
#13322=ORIENTED_EDGE('',*,*,#8214,.F.);
#13323=ORIENTED_EDGE('',*,*,#9505,.F.);
#13324=ORIENTED_EDGE('',*,*,#8193,.F.);
#13325=ORIENTED_EDGE('',*,*,#9512,.T.);
#13326=ORIENTED_EDGE('',*,*,#8199,.F.);
#13327=ORIENTED_EDGE('',*,*,#9504,.F.);
#13328=ORIENTED_EDGE('',*,*,#8178,.F.);
#13329=ORIENTED_EDGE('',*,*,#9513,.T.);
#13330=ORIENTED_EDGE('',*,*,#8184,.F.);
#13331=ORIENTED_EDGE('',*,*,#9503,.F.);
#13332=ORIENTED_EDGE('',*,*,#8163,.F.);
#13333=ORIENTED_EDGE('',*,*,#9514,.T.);
#13334=ORIENTED_EDGE('',*,*,#8169,.F.);
#13335=ORIENTED_EDGE('',*,*,#9502,.F.);
#13336=ORIENTED_EDGE('',*,*,#8148,.F.);
#13337=ORIENTED_EDGE('',*,*,#9515,.T.);
#13338=ORIENTED_EDGE('',*,*,#8154,.F.);
#13339=ORIENTED_EDGE('',*,*,#9501,.F.);
#13340=ORIENTED_EDGE('',*,*,#8126,.F.);
#13341=ORIENTED_EDGE('',*,*,#9516,.T.);
#13342=ORIENTED_EDGE('',*,*,#8139,.F.);
#13343=ORIENTED_EDGE('',*,*,#9500,.F.);
#13344=ORIENTED_EDGE('',*,*,#9517,.T.);
#13345=ORIENTED_EDGE('',*,*,#9518,.T.);
#13346=ORIENTED_EDGE('',*,*,#9519,.T.);
#13347=ORIENTED_EDGE('',*,*,#8120,.F.);
#13348=ORIENTED_EDGE('',*,*,#8133,.F.);
#13349=ORIENTED_EDGE('',*,*,#8279,.F.);
#13350=ORIENTED_EDGE('',*,*,#8121,.F.);
#13351=ORIENTED_EDGE('',*,*,#9519,.F.);
#13352=ORIENTED_EDGE('',*,*,#9520,.T.);
#13353=ORIENTED_EDGE('',*,*,#9498,.F.);
#13354=ORIENTED_EDGE('',*,*,#8429,.T.);
#13355=ORIENTED_EDGE('',*,*,#9521,.F.);
#13356=ORIENTED_EDGE('',*,*,#9522,.T.);
#13357=ORIENTED_EDGE('',*,*,#9523,.T.);
#13358=ORIENTED_EDGE('',*,*,#9524,.T.);
#13359=ORIENTED_EDGE('',*,*,#9525,.T.);
#13360=ORIENTED_EDGE('',*,*,#9526,.T.);
#13361=ORIENTED_EDGE('',*,*,#8268,.T.);
#13362=ORIENTED_EDGE('',*,*,#8430,.T.);
#13363=ORIENTED_EDGE('',*,*,#9523,.F.);
#13364=ORIENTED_EDGE('',*,*,#9527,.T.);
#13365=ORIENTED_EDGE('',*,*,#9528,.T.);
#13366=ORIENTED_EDGE('',*,*,#9529,.T.);
#13367=ORIENTED_EDGE('',*,*,#9525,.F.);
#13368=ORIENTED_EDGE('',*,*,#9526,.F.);
#13369=ORIENTED_EDGE('',*,*,#9529,.F.);
#13370=ORIENTED_EDGE('',*,*,#9530,.T.);
#13371=ORIENTED_EDGE('',*,*,#9531,.F.);
#13372=ORIENTED_EDGE('',*,*,#9532,.F.);
#13373=ORIENTED_EDGE('',*,*,#8269,.F.);
#13374=ORIENTED_EDGE('',*,*,#9533,.T.);
#13375=ORIENTED_EDGE('',*,*,#9534,.F.);
#13376=ORIENTED_EDGE('',*,*,#9535,.T.);
#13377=ORIENTED_EDGE('',*,*,#9536,.T.);
#13378=ORIENTED_EDGE('',*,*,#9537,.T.);
#13379=ORIENTED_EDGE('',*,*,#9538,.T.);
#13380=ORIENTED_EDGE('',*,*,#8116,.T.);
#13381=ORIENTED_EDGE('',*,*,#8278,.T.);
#13382=ORIENTED_EDGE('',*,*,#9539,.T.);
#13383=ORIENTED_EDGE('',*,*,#9536,.F.);
#13384=ORIENTED_EDGE('',*,*,#9540,.T.);
#13385=ORIENTED_EDGE('',*,*,#9541,.T.);
#13386=ORIENTED_EDGE('',*,*,#8117,.T.);
#13387=ORIENTED_EDGE('',*,*,#9538,.F.);
#13388=ORIENTED_EDGE('',*,*,#9533,.F.);
#13389=ORIENTED_EDGE('',*,*,#9539,.F.);
#13390=ORIENTED_EDGE('',*,*,#8277,.F.);
#13391=ORIENTED_EDGE('',*,*,#9542,.F.);
#13392=ORIENTED_EDGE('',*,*,#9543,.F.);
#13393=ORIENTED_EDGE('',*,*,#9544,.T.);
#13394=ORIENTED_EDGE('',*,*,#9531,.T.);
#13395=ORIENTED_EDGE('',*,*,#9545,.F.);
#13396=ORIENTED_EDGE('',*,*,#9546,.T.);
#13397=ORIENTED_EDGE('',*,*,#9547,.T.);
#13398=ORIENTED_EDGE('',*,*,#9548,.T.);
#13399=ORIENTED_EDGE('',*,*,#9549,.T.);
#13400=ORIENTED_EDGE('',*,*,#9550,.T.);
#13401=ORIENTED_EDGE('',*,*,#8270,.T.);
#13402=ORIENTED_EDGE('',*,*,#9532,.T.);
#13403=ORIENTED_EDGE('',*,*,#9547,.F.);
#13404=ORIENTED_EDGE('',*,*,#9551,.T.);
#13405=ORIENTED_EDGE('',*,*,#9552,.T.);
#13406=ORIENTED_EDGE('',*,*,#9553,.T.);
#13407=ORIENTED_EDGE('',*,*,#9549,.F.);
#13408=ORIENTED_EDGE('',*,*,#9550,.F.);
#13409=ORIENTED_EDGE('',*,*,#9553,.F.);
#13410=ORIENTED_EDGE('',*,*,#9554,.T.);
#13411=ORIENTED_EDGE('',*,*,#9555,.F.);
#13412=ORIENTED_EDGE('',*,*,#9556,.F.);
#13413=ORIENTED_EDGE('',*,*,#8271,.F.);
#13414=ORIENTED_EDGE('',*,*,#9557,.T.);
#13415=ORIENTED_EDGE('',*,*,#9558,.F.);
#13416=ORIENTED_EDGE('',*,*,#9559,.T.);
#13417=ORIENTED_EDGE('',*,*,#9560,.T.);
#13418=ORIENTED_EDGE('',*,*,#9561,.T.);
#13419=ORIENTED_EDGE('',*,*,#9562,.T.);
#13420=ORIENTED_EDGE('',*,*,#9542,.T.);
#13421=ORIENTED_EDGE('',*,*,#8276,.T.);
#13422=ORIENTED_EDGE('',*,*,#9563,.T.);
#13423=ORIENTED_EDGE('',*,*,#9560,.F.);
#13424=ORIENTED_EDGE('',*,*,#9564,.T.);
#13425=ORIENTED_EDGE('',*,*,#9565,.T.);
#13426=ORIENTED_EDGE('',*,*,#9543,.T.);
#13427=ORIENTED_EDGE('',*,*,#9562,.F.);
#13428=ORIENTED_EDGE('',*,*,#9557,.F.);
#13429=ORIENTED_EDGE('',*,*,#9563,.F.);
#13430=ORIENTED_EDGE('',*,*,#8275,.F.);
#13431=ORIENTED_EDGE('',*,*,#9566,.F.);
#13432=ORIENTED_EDGE('',*,*,#9567,.F.);
#13433=ORIENTED_EDGE('',*,*,#9568,.T.);
#13434=ORIENTED_EDGE('',*,*,#9555,.T.);
#13435=ORIENTED_EDGE('',*,*,#9569,.F.);
#13436=ORIENTED_EDGE('',*,*,#9570,.T.);
#13437=ORIENTED_EDGE('',*,*,#9571,.T.);
#13438=ORIENTED_EDGE('',*,*,#9572,.T.);
#13439=ORIENTED_EDGE('',*,*,#9573,.T.);
#13440=ORIENTED_EDGE('',*,*,#9574,.T.);
#13441=ORIENTED_EDGE('',*,*,#8272,.T.);
#13442=ORIENTED_EDGE('',*,*,#9556,.T.);
#13443=ORIENTED_EDGE('',*,*,#9571,.F.);
#13444=ORIENTED_EDGE('',*,*,#9575,.T.);
#13445=ORIENTED_EDGE('',*,*,#9576,.T.);
#13446=ORIENTED_EDGE('',*,*,#9577,.T.);
#13447=ORIENTED_EDGE('',*,*,#9573,.F.);
#13448=ORIENTED_EDGE('',*,*,#9574,.F.);
#13449=ORIENTED_EDGE('',*,*,#9577,.F.);
#13450=ORIENTED_EDGE('',*,*,#9578,.T.);
#13451=ORIENTED_EDGE('',*,*,#9579,.F.);
#13452=ORIENTED_EDGE('',*,*,#9580,.F.);
#13453=ORIENTED_EDGE('',*,*,#8273,.F.);
#13454=ORIENTED_EDGE('',*,*,#9579,.T.);
#13455=ORIENTED_EDGE('',*,*,#9581,.F.);
#13456=ORIENTED_EDGE('',*,*,#9582,.T.);
#13457=ORIENTED_EDGE('',*,*,#9583,.T.);
#13458=ORIENTED_EDGE('',*,*,#9584,.T.);
#13459=ORIENTED_EDGE('',*,*,#9585,.T.);
#13460=ORIENTED_EDGE('',*,*,#9566,.T.);
#13461=ORIENTED_EDGE('',*,*,#8274,.T.);
#13462=ORIENTED_EDGE('',*,*,#9580,.T.);
#13463=ORIENTED_EDGE('',*,*,#9583,.F.);
#13464=ORIENTED_EDGE('',*,*,#9586,.T.);
#13465=ORIENTED_EDGE('',*,*,#9587,.T.);
#13466=ORIENTED_EDGE('',*,*,#9567,.T.);
#13467=ORIENTED_EDGE('',*,*,#9585,.F.);
#13468=ORIENTED_EDGE('',*,*,#9588,.T.);
#13469=ORIENTED_EDGE('',*,*,#9589,.T.);
#13470=ORIENTED_EDGE('',*,*,#9590,.T.);
#13471=ORIENTED_EDGE('',*,*,#9589,.F.);
#13472=ORIENTED_EDGE('',*,*,#9590,.F.);
#13473=ORIENTED_EDGE('',*,*,#9591,.F.);
#13474=ORIENTED_EDGE('',*,*,#9588,.F.);
#13475=ORIENTED_EDGE('',*,*,#9592,.T.);
#13476=ORIENTED_EDGE('',*,*,#9593,.T.);
#13477=ORIENTED_EDGE('',*,*,#9594,.T.);
#13478=ORIENTED_EDGE('',*,*,#9595,.T.);
#13479=ORIENTED_EDGE('',*,*,#9596,.T.);
#13480=ORIENTED_EDGE('',*,*,#9597,.T.);
#13481=ORIENTED_EDGE('',*,*,#9598,.T.);
#13482=ORIENTED_EDGE('',*,*,#9599,.T.);
#13483=ORIENTED_EDGE('',*,*,#9600,.T.);
#13484=ORIENTED_EDGE('',*,*,#9601,.T.);
#13485=ORIENTED_EDGE('',*,*,#9602,.T.);
#13486=ORIENTED_EDGE('',*,*,#9603,.T.);
#13487=ORIENTED_EDGE('',*,*,#9604,.T.);
#13488=ORIENTED_EDGE('',*,*,#9605,.T.);
#13489=ORIENTED_EDGE('',*,*,#9606,.T.);
#13490=ORIENTED_EDGE('',*,*,#9607,.T.);
#13491=ORIENTED_EDGE('',*,*,#8060,.T.);
#13492=ORIENTED_EDGE('',*,*,#9608,.T.);
#13493=ORIENTED_EDGE('',*,*,#8477,.T.);
#13494=ORIENTED_EDGE('',*,*,#9609,.T.);
#13495=ORIENTED_EDGE('',*,*,#8568,.T.);
#13496=ORIENTED_EDGE('',*,*,#9610,.T.);
#13497=ORIENTED_EDGE('',*,*,#8569,.T.);
#13498=ORIENTED_EDGE('',*,*,#9611,.T.);
#13499=ORIENTED_EDGE('',*,*,#8570,.T.);
#13500=ORIENTED_EDGE('',*,*,#9612,.T.);
#13501=ORIENTED_EDGE('',*,*,#8558,.T.);
#13502=ORIENTED_EDGE('',*,*,#9613,.T.);
#13503=ORIENTED_EDGE('',*,*,#8544,.T.);
#13504=ORIENTED_EDGE('',*,*,#9614,.T.);
#13505=ORIENTED_EDGE('',*,*,#8530,.T.);
#13506=ORIENTED_EDGE('',*,*,#9615,.T.);
#13507=ORIENTED_EDGE('',*,*,#8516,.T.);
#13508=ORIENTED_EDGE('',*,*,#9616,.T.);
#13509=ORIENTED_EDGE('',*,*,#8502,.T.);
#13510=ORIENTED_EDGE('',*,*,#9617,.T.);
#13511=ORIENTED_EDGE('',*,*,#8488,.T.);
#13512=ORIENTED_EDGE('',*,*,#9618,.T.);
#13513=ORIENTED_EDGE('',*,*,#8644,.T.);
#13514=ORIENTED_EDGE('',*,*,#9619,.T.);
#13515=ORIENTED_EDGE('',*,*,#8722,.T.);
#13516=ORIENTED_EDGE('',*,*,#9620,.T.);
#13517=ORIENTED_EDGE('',*,*,#8723,.T.);
#13518=ORIENTED_EDGE('',*,*,#9621,.T.);
#13519=ORIENTED_EDGE('',*,*,#8724,.T.);
#13520=ORIENTED_EDGE('',*,*,#9622,.T.);
#13521=ORIENTED_EDGE('',*,*,#8725,.T.);
#13522=ORIENTED_EDGE('',*,*,#9623,.T.);
#13523=ORIENTED_EDGE('',*,*,#8712,.T.);
#13524=ORIENTED_EDGE('',*,*,#9624,.T.);
#13525=ORIENTED_EDGE('',*,*,#8698,.T.);
#13526=ORIENTED_EDGE('',*,*,#9625,.T.);
#13527=ORIENTED_EDGE('',*,*,#8684,.T.);
#13528=ORIENTED_EDGE('',*,*,#9626,.T.);
#13529=ORIENTED_EDGE('',*,*,#8670,.T.);
#13530=ORIENTED_EDGE('',*,*,#9627,.T.);
#13531=ORIENTED_EDGE('',*,*,#8656,.T.);
#13532=ORIENTED_EDGE('',*,*,#9628,.T.);
#13533=ORIENTED_EDGE('',*,*,#8810,.T.);
#13534=ORIENTED_EDGE('',*,*,#9629,.T.);
#13535=ORIENTED_EDGE('',*,*,#8876,.T.);
#13536=ORIENTED_EDGE('',*,*,#9630,.T.);
#13537=ORIENTED_EDGE('',*,*,#8877,.T.);
#13538=ORIENTED_EDGE('',*,*,#9631,.T.);
#13539=ORIENTED_EDGE('',*,*,#8878,.T.);
#13540=ORIENTED_EDGE('',*,*,#9632,.T.);
#13541=ORIENTED_EDGE('',*,*,#8879,.T.);
#13542=ORIENTED_EDGE('',*,*,#9633,.T.);
#13543=ORIENTED_EDGE('',*,*,#8880,.T.);
#13544=ORIENTED_EDGE('',*,*,#9634,.T.);
#13545=ORIENTED_EDGE('',*,*,#8864,.T.);
#13546=ORIENTED_EDGE('',*,*,#9635,.T.);
#13547=ORIENTED_EDGE('',*,*,#8850,.T.);
#13548=ORIENTED_EDGE('',*,*,#9636,.T.);
#13549=ORIENTED_EDGE('',*,*,#8836,.T.);
#13550=ORIENTED_EDGE('',*,*,#9637,.T.);
#13551=ORIENTED_EDGE('',*,*,#8822,.T.);
#13552=ORIENTED_EDGE('',*,*,#9638,.T.);
#13553=ORIENTED_EDGE('',*,*,#8978,.T.);
#13554=ORIENTED_EDGE('',*,*,#9639,.T.);
#13555=ORIENTED_EDGE('',*,*,#9030,.T.);
#13556=ORIENTED_EDGE('',*,*,#9640,.T.);
#13557=ORIENTED_EDGE('',*,*,#9031,.T.);
#13558=ORIENTED_EDGE('',*,*,#9641,.T.);
#13559=ORIENTED_EDGE('',*,*,#9032,.T.);
#13560=ORIENTED_EDGE('',*,*,#9642,.T.);
#13561=ORIENTED_EDGE('',*,*,#9033,.T.);
#13562=ORIENTED_EDGE('',*,*,#9643,.T.);
#13563=ORIENTED_EDGE('',*,*,#9034,.T.);
#13564=ORIENTED_EDGE('',*,*,#9644,.T.);
#13565=ORIENTED_EDGE('',*,*,#9035,.T.);
#13566=ORIENTED_EDGE('',*,*,#9645,.T.);
#13567=ORIENTED_EDGE('',*,*,#9018,.T.);
#13568=ORIENTED_EDGE('',*,*,#9646,.T.);
#13569=ORIENTED_EDGE('',*,*,#9004,.T.);
#13570=ORIENTED_EDGE('',*,*,#9647,.T.);
#13571=ORIENTED_EDGE('',*,*,#8990,.T.);
#13572=ORIENTED_EDGE('',*,*,#9648,.T.);
#13573=ORIENTED_EDGE('',*,*,#9144,.T.);
#13574=ORIENTED_EDGE('',*,*,#9649,.T.);
#13575=ORIENTED_EDGE('',*,*,#9184,.T.);
#13576=ORIENTED_EDGE('',*,*,#9650,.T.);
#13577=ORIENTED_EDGE('',*,*,#9185,.T.);
#13578=ORIENTED_EDGE('',*,*,#9651,.T.);
#13579=ORIENTED_EDGE('',*,*,#9186,.T.);
#13580=ORIENTED_EDGE('',*,*,#9652,.T.);
#13581=ORIENTED_EDGE('',*,*,#9187,.T.);
#13582=ORIENTED_EDGE('',*,*,#9653,.T.);
#13583=ORIENTED_EDGE('',*,*,#9188,.T.);
#13584=ORIENTED_EDGE('',*,*,#9654,.T.);
#13585=ORIENTED_EDGE('',*,*,#9189,.T.);
#13586=ORIENTED_EDGE('',*,*,#9655,.T.);
#13587=ORIENTED_EDGE('',*,*,#9190,.T.);
#13588=ORIENTED_EDGE('',*,*,#9656,.T.);
#13589=ORIENTED_EDGE('',*,*,#9170,.T.);
#13590=ORIENTED_EDGE('',*,*,#9657,.T.);
#13591=ORIENTED_EDGE('',*,*,#9156,.T.);
#13592=ORIENTED_EDGE('',*,*,#9658,.T.);
#13593=ORIENTED_EDGE('',*,*,#9311,.T.);
#13594=ORIENTED_EDGE('',*,*,#9659,.T.);
#13595=ORIENTED_EDGE('',*,*,#9338,.T.);
#13596=ORIENTED_EDGE('',*,*,#9660,.T.);
#13597=ORIENTED_EDGE('',*,*,#9339,.T.);
#13598=ORIENTED_EDGE('',*,*,#9661,.T.);
#13599=ORIENTED_EDGE('',*,*,#9340,.T.);
#13600=ORIENTED_EDGE('',*,*,#9662,.T.);
#13601=ORIENTED_EDGE('',*,*,#9341,.T.);
#13602=ORIENTED_EDGE('',*,*,#9663,.T.);
#13603=ORIENTED_EDGE('',*,*,#9342,.T.);
#13604=ORIENTED_EDGE('',*,*,#9664,.T.);
#13605=ORIENTED_EDGE('',*,*,#9343,.T.);
#13606=ORIENTED_EDGE('',*,*,#9665,.T.);
#13607=ORIENTED_EDGE('',*,*,#9344,.T.);
#13608=ORIENTED_EDGE('',*,*,#9666,.T.);
#13609=ORIENTED_EDGE('',*,*,#9345,.T.);
#13610=ORIENTED_EDGE('',*,*,#9667,.T.);
#13611=ORIENTED_EDGE('',*,*,#9323,.T.);
#13612=ORIENTED_EDGE('',*,*,#9668,.T.);
#13613=ORIENTED_EDGE('',*,*,#8048,.T.);
#13614=ORIENTED_EDGE('',*,*,#9669,.T.);
#13615=ORIENTED_EDGE('',*,*,#9468,.T.);
#13616=ORIENTED_EDGE('',*,*,#9670,.T.);
#13617=ORIENTED_EDGE('',*,*,#9454,.T.);
#13618=ORIENTED_EDGE('',*,*,#9671,.T.);
#13619=ORIENTED_EDGE('',*,*,#9440,.T.);
#13620=ORIENTED_EDGE('',*,*,#9672,.T.);
#13621=ORIENTED_EDGE('',*,*,#9426,.T.);
#13622=ORIENTED_EDGE('',*,*,#9673,.T.);
#13623=ORIENTED_EDGE('',*,*,#9412,.T.);
#13624=ORIENTED_EDGE('',*,*,#9674,.T.);
#13625=ORIENTED_EDGE('',*,*,#9398,.T.);
#13626=ORIENTED_EDGE('',*,*,#9675,.T.);
#13627=ORIENTED_EDGE('',*,*,#9384,.T.);
#13628=ORIENTED_EDGE('',*,*,#9676,.T.);
#13629=ORIENTED_EDGE('',*,*,#9370,.T.);
#13630=ORIENTED_EDGE('',*,*,#9677,.T.);
#13631=ORIENTED_EDGE('',*,*,#9356,.T.);
#13632=ORIENTED_EDGE('',*,*,#9678,.T.);
#13633=ORIENTED_EDGE('',*,*,#8250,.T.);
#13634=ORIENTED_EDGE('',*,*,#9679,.T.);
#13635=ORIENTED_EDGE('',*,*,#8235,.T.);
#13636=ORIENTED_EDGE('',*,*,#9680,.T.);
#13637=ORIENTED_EDGE('',*,*,#8220,.T.);
#13638=ORIENTED_EDGE('',*,*,#9681,.T.);
#13639=ORIENTED_EDGE('',*,*,#8205,.T.);
#13640=ORIENTED_EDGE('',*,*,#9682,.T.);
#13641=ORIENTED_EDGE('',*,*,#8190,.T.);
#13642=ORIENTED_EDGE('',*,*,#9683,.T.);
#13643=ORIENTED_EDGE('',*,*,#8175,.T.);
#13644=ORIENTED_EDGE('',*,*,#9684,.T.);
#13645=ORIENTED_EDGE('',*,*,#8160,.T.);
#13646=ORIENTED_EDGE('',*,*,#9685,.T.);
#13647=ORIENTED_EDGE('',*,*,#8145,.T.);
#13648=ORIENTED_EDGE('',*,*,#9686,.T.);
#13649=ORIENTED_EDGE('',*,*,#8130,.T.);
#13650=ORIENTED_EDGE('',*,*,#9687,.T.);
#13651=ORIENTED_EDGE('',*,*,#9688,.T.);
#13652=ORIENTED_EDGE('',*,*,#9689,.T.);
#13653=ORIENTED_EDGE('',*,*,#9690,.T.);
#13654=ORIENTED_EDGE('',*,*,#9691,.T.);
#13655=ORIENTED_EDGE('',*,*,#9692,.T.);
#13656=ORIENTED_EDGE('',*,*,#9693,.T.);
#13657=ORIENTED_EDGE('',*,*,#9592,.F.);
#13658=ORIENTED_EDGE('',*,*,#9694,.T.);
#13659=ORIENTED_EDGE('',*,*,#9695,.T.);
#13660=ORIENTED_EDGE('',*,*,#9696,.T.);
#13661=ORIENTED_EDGE('',*,*,#9695,.F.);
#13662=ORIENTED_EDGE('',*,*,#9697,.T.);
#13663=ORIENTED_EDGE('',*,*,#9698,.F.);
#13664=ORIENTED_EDGE('',*,*,#9699,.F.);
#13665=ORIENTED_EDGE('',*,*,#9700,.T.);
#13666=ORIENTED_EDGE('',*,*,#9701,.F.);
#13667=ORIENTED_EDGE('',*,*,#9702,.F.);
#13668=ORIENTED_EDGE('',*,*,#9694,.F.);
#13669=ORIENTED_EDGE('',*,*,#9696,.F.);
#13670=ORIENTED_EDGE('',*,*,#9703,.T.);
#13671=ORIENTED_EDGE('',*,*,#9704,.F.);
#13672=ORIENTED_EDGE('',*,*,#9703,.F.);
#13673=ORIENTED_EDGE('',*,*,#9698,.T.);
#13674=ORIENTED_EDGE('',*,*,#9705,.T.);
#13675=ORIENTED_EDGE('',*,*,#9706,.T.);
#13676=ORIENTED_EDGE('',*,*,#9705,.F.);
#13677=ORIENTED_EDGE('',*,*,#9706,.F.);
#13678=ORIENTED_EDGE('',*,*,#9707,.T.);
#13679=ORIENTED_EDGE('',*,*,#9708,.F.);
#13680=ORIENTED_EDGE('',*,*,#9707,.F.);
#13681=ORIENTED_EDGE('',*,*,#9702,.T.);
#13682=ORIENTED_EDGE('',*,*,#9709,.T.);
#13683=ORIENTED_EDGE('',*,*,#9710,.T.);
#13684=ORIENTED_EDGE('',*,*,#9709,.F.);
#13685=ORIENTED_EDGE('',*,*,#9710,.F.);
#13686=ORIENTED_EDGE('',*,*,#9711,.T.);
#13687=ORIENTED_EDGE('',*,*,#9712,.F.);
#13688=ORIENTED_EDGE('',*,*,#9711,.F.);
#13689=ORIENTED_EDGE('',*,*,#9699,.T.);
#13690=ORIENTED_EDGE('',*,*,#9713,.T.);
#13691=ORIENTED_EDGE('',*,*,#9714,.T.);
#13692=ORIENTED_EDGE('',*,*,#9713,.F.);
#13693=ORIENTED_EDGE('',*,*,#9714,.F.);
#13694=ORIENTED_EDGE('',*,*,#9715,.T.);
#13695=ORIENTED_EDGE('',*,*,#9716,.F.);
#13696=ORIENTED_EDGE('',*,*,#9715,.F.);
#13697=ORIENTED_EDGE('',*,*,#9701,.T.);
#13698=ORIENTED_EDGE('',*,*,#9717,.T.);
#13699=ORIENTED_EDGE('',*,*,#9718,.T.);
#13700=ORIENTED_EDGE('',*,*,#9717,.F.);
#13701=ORIENTED_EDGE('',*,*,#9718,.F.);
#13702=ORIENTED_EDGE('',*,*,#9719,.T.);
#13703=ORIENTED_EDGE('',*,*,#9720,.F.);
#13704=ORIENTED_EDGE('',*,*,#9719,.F.);
#13705=ORIENTED_EDGE('',*,*,#9591,.T.);
#13706=ORIENTED_EDGE('',*,*,#9721,.T.);
#13707=ORIENTED_EDGE('',*,*,#9722,.T.);
#13708=ORIENTED_EDGE('',*,*,#9721,.F.);
#13709=ORIENTED_EDGE('',*,*,#9722,.F.);
#13710=ORIENTED_EDGE('',*,*,#9723,.T.);
#13711=ORIENTED_EDGE('',*,*,#9697,.F.);
#13712=ORIENTED_EDGE('',*,*,#9723,.F.);
#13713=ORIENTED_EDGE('',*,*,#9582,.F.);
#13714=ORIENTED_EDGE('',*,*,#9594,.F.);
#13715=ORIENTED_EDGE('',*,*,#9586,.F.);
#13716=ORIENTED_EDGE('',*,*,#9584,.F.);
#13717=ORIENTED_EDGE('',*,*,#9570,.F.);
#13718=ORIENTED_EDGE('',*,*,#9596,.F.);
#13719=ORIENTED_EDGE('',*,*,#9575,.F.);
#13720=ORIENTED_EDGE('',*,*,#9572,.F.);
#13721=ORIENTED_EDGE('',*,*,#9559,.F.);
#13722=ORIENTED_EDGE('',*,*,#9692,.F.);
#13723=ORIENTED_EDGE('',*,*,#9564,.F.);
#13724=ORIENTED_EDGE('',*,*,#9561,.F.);
#13725=ORIENTED_EDGE('',*,*,#9546,.F.);
#13726=ORIENTED_EDGE('',*,*,#9598,.F.);
#13727=ORIENTED_EDGE('',*,*,#9551,.F.);
#13728=ORIENTED_EDGE('',*,*,#9548,.F.);
#13729=ORIENTED_EDGE('',*,*,#9535,.F.);
#13730=ORIENTED_EDGE('',*,*,#9690,.F.);
#13731=ORIENTED_EDGE('',*,*,#9540,.F.);
#13732=ORIENTED_EDGE('',*,*,#9537,.F.);
#13733=ORIENTED_EDGE('',*,*,#9522,.F.);
#13734=ORIENTED_EDGE('',*,*,#9600,.F.);
#13735=ORIENTED_EDGE('',*,*,#9527,.F.);
#13736=ORIENTED_EDGE('',*,*,#9524,.F.);
#13737=ORIENTED_EDGE('',*,*,#8111,.F.);
#13738=ORIENTED_EDGE('',*,*,#9688,.F.);
#13739=ORIENTED_EDGE('',*,*,#9517,.F.);
#13740=ORIENTED_EDGE('',*,*,#8119,.F.);
#13741=ORIENTED_EDGE('',*,*,#8108,.F.);
#13742=ORIENTED_EDGE('',*,*,#9602,.F.);
#13743=ORIENTED_EDGE('',*,*,#8431,.F.);
#13744=ORIENTED_EDGE('',*,*,#8263,.F.);
#13745=ORIENTED_EDGE('',*,*,#8093,.F.);
#13746=ORIENTED_EDGE('',*,*,#8262,.F.);
#13747=ORIENTED_EDGE('',*,*,#8105,.F.);
#13748=ORIENTED_EDGE('',*,*,#9604,.F.);
#13749=ORIENTED_EDGE('',*,*,#8072,.F.);
#13750=ORIENTED_EDGE('',*,*,#8260,.F.);
#13751=ORIENTED_EDGE('',*,*,#8084,.F.);
#13752=ORIENTED_EDGE('',*,*,#9606,.F.);
#13753=ORIENTED_EDGE('',*,*,#9644,.F.);
#13754=ORIENTED_EDGE('',*,*,#8901,.T.);
#13755=ORIENTED_EDGE('',*,*,#8899,.F.);
#13756=ORIENTED_EDGE('',*,*,#8892,.F.);
#13757=ORIENTED_EDGE('',*,*,#9643,.F.);
#13758=ORIENTED_EDGE('',*,*,#8916,.T.);
#13759=ORIENTED_EDGE('',*,*,#8914,.F.);
#13760=ORIENTED_EDGE('',*,*,#8908,.F.);
#13761=ORIENTED_EDGE('',*,*,#9642,.F.);
#13762=ORIENTED_EDGE('',*,*,#8930,.T.);
#13763=ORIENTED_EDGE('',*,*,#8928,.F.);
#13764=ORIENTED_EDGE('',*,*,#8921,.F.);
#13765=ORIENTED_EDGE('',*,*,#9641,.F.);
#13766=ORIENTED_EDGE('',*,*,#8944,.T.);
#13767=ORIENTED_EDGE('',*,*,#8942,.F.);
#13768=ORIENTED_EDGE('',*,*,#8935,.F.);
#13769=ORIENTED_EDGE('',*,*,#9640,.F.);
#13770=ORIENTED_EDGE('',*,*,#8958,.T.);
#13771=ORIENTED_EDGE('',*,*,#8956,.F.);
#13772=ORIENTED_EDGE('',*,*,#8949,.F.);
#13773=ORIENTED_EDGE('',*,*,#9639,.F.);
#13774=ORIENTED_EDGE('',*,*,#8981,.T.);
#13775=ORIENTED_EDGE('',*,*,#8970,.F.);
#13776=ORIENTED_EDGE('',*,*,#8963,.F.);
#13777=ORIENTED_EDGE('',*,*,#8817,.F.);
#13778=ORIENTED_EDGE('',*,*,#8821,.T.);
#13779=ORIENTED_EDGE('',*,*,#8366,.F.);
#13780=ORIENTED_EDGE('',*,*,#8979,.T.);
#13781=ORIENTED_EDGE('',*,*,#8975,.F.);
#13782=ORIENTED_EDGE('',*,*,#9724,.T.);
#13783=ORIENTED_EDGE('',*,*,#9638,.F.);
#13784=ORIENTED_EDGE('',*,*,#8814,.T.);
#13785=ORIENTED_EDGE('',*,*,#9724,.F.);
#13786=ORIENTED_EDGE('',*,*,#8974,.F.);
#13787=ORIENTED_EDGE('',*,*,#9637,.F.);
#13788=ORIENTED_EDGE('',*,*,#8827,.T.);
#13789=ORIENTED_EDGE('',*,*,#8889,.F.);
#13790=ORIENTED_EDGE('',*,*,#8824,.F.);
#13791=ORIENTED_EDGE('',*,*,#9636,.F.);
#13792=ORIENTED_EDGE('',*,*,#8841,.T.);
#13793=ORIENTED_EDGE('',*,*,#8888,.F.);
#13794=ORIENTED_EDGE('',*,*,#8838,.F.);
#13795=ORIENTED_EDGE('',*,*,#9635,.F.);
#13796=ORIENTED_EDGE('',*,*,#8855,.T.);
#13797=ORIENTED_EDGE('',*,*,#8887,.F.);
#13798=ORIENTED_EDGE('',*,*,#8852,.F.);
#13799=ORIENTED_EDGE('',*,*,#9634,.F.);
#13800=ORIENTED_EDGE('',*,*,#8867,.T.);
#13801=ORIENTED_EDGE('',*,*,#8886,.F.);
#13802=ORIENTED_EDGE('',*,*,#8881,.F.);
#13803=ORIENTED_EDGE('',*,*,#9633,.F.);
#13804=ORIENTED_EDGE('',*,*,#8748,.T.);
#13805=ORIENTED_EDGE('',*,*,#8746,.F.);
#13806=ORIENTED_EDGE('',*,*,#8739,.F.);
#13807=ORIENTED_EDGE('',*,*,#9632,.F.);
#13808=ORIENTED_EDGE('',*,*,#8762,.T.);
#13809=ORIENTED_EDGE('',*,*,#8760,.F.);
#13810=ORIENTED_EDGE('',*,*,#8753,.F.);
#13811=ORIENTED_EDGE('',*,*,#9631,.F.);
#13812=ORIENTED_EDGE('',*,*,#8776,.T.);
#13813=ORIENTED_EDGE('',*,*,#8774,.F.);
#13814=ORIENTED_EDGE('',*,*,#8767,.F.);
#13815=ORIENTED_EDGE('',*,*,#9630,.F.);
#13816=ORIENTED_EDGE('',*,*,#8790,.T.);
#13817=ORIENTED_EDGE('',*,*,#8788,.F.);
#13818=ORIENTED_EDGE('',*,*,#8781,.F.);
#13819=ORIENTED_EDGE('',*,*,#9629,.F.);
#13820=ORIENTED_EDGE('',*,*,#8813,.T.);
#13821=ORIENTED_EDGE('',*,*,#8802,.F.);
#13822=ORIENTED_EDGE('',*,*,#8795,.F.);
#13823=ORIENTED_EDGE('',*,*,#8651,.F.);
#13824=ORIENTED_EDGE('',*,*,#8655,.T.);
#13825=ORIENTED_EDGE('',*,*,#8386,.F.);
#13826=ORIENTED_EDGE('',*,*,#8811,.T.);
#13827=ORIENTED_EDGE('',*,*,#8807,.F.);
#13828=ORIENTED_EDGE('',*,*,#9725,.T.);
#13829=ORIENTED_EDGE('',*,*,#9628,.F.);
#13830=ORIENTED_EDGE('',*,*,#8648,.T.);
#13831=ORIENTED_EDGE('',*,*,#9725,.F.);
#13832=ORIENTED_EDGE('',*,*,#8806,.F.);
#13833=ORIENTED_EDGE('',*,*,#9627,.F.);
#13834=ORIENTED_EDGE('',*,*,#8661,.T.);
#13835=ORIENTED_EDGE('',*,*,#8736,.F.);
#13836=ORIENTED_EDGE('',*,*,#8658,.F.);
#13837=ORIENTED_EDGE('',*,*,#9626,.F.);
#13838=ORIENTED_EDGE('',*,*,#8675,.T.);
#13839=ORIENTED_EDGE('',*,*,#8735,.F.);
#13840=ORIENTED_EDGE('',*,*,#8672,.F.);
#13841=ORIENTED_EDGE('',*,*,#9625,.F.);
#13842=ORIENTED_EDGE('',*,*,#8689,.T.);
#13843=ORIENTED_EDGE('',*,*,#8734,.F.);
#13844=ORIENTED_EDGE('',*,*,#8686,.F.);
#13845=ORIENTED_EDGE('',*,*,#9624,.F.);
#13846=ORIENTED_EDGE('',*,*,#8703,.T.);
#13847=ORIENTED_EDGE('',*,*,#8733,.F.);
#13848=ORIENTED_EDGE('',*,*,#8700,.F.);
#13849=ORIENTED_EDGE('',*,*,#9623,.F.);
#13850=ORIENTED_EDGE('',*,*,#8715,.T.);
#13851=ORIENTED_EDGE('',*,*,#8732,.F.);
#13852=ORIENTED_EDGE('',*,*,#8726,.F.);
#13853=ORIENTED_EDGE('',*,*,#9622,.F.);
#13854=ORIENTED_EDGE('',*,*,#8595,.T.);
#13855=ORIENTED_EDGE('',*,*,#8593,.F.);
#13856=ORIENTED_EDGE('',*,*,#8586,.F.);
#13857=ORIENTED_EDGE('',*,*,#9621,.F.);
#13858=ORIENTED_EDGE('',*,*,#8610,.T.);
#13859=ORIENTED_EDGE('',*,*,#8608,.F.);
#13860=ORIENTED_EDGE('',*,*,#8602,.F.);
#13861=ORIENTED_EDGE('',*,*,#9620,.F.);
#13862=ORIENTED_EDGE('',*,*,#8624,.T.);
#13863=ORIENTED_EDGE('',*,*,#8622,.F.);
#13864=ORIENTED_EDGE('',*,*,#8615,.F.);
#13865=ORIENTED_EDGE('',*,*,#9619,.F.);
#13866=ORIENTED_EDGE('',*,*,#8647,.T.);
#13867=ORIENTED_EDGE('',*,*,#8636,.F.);
#13868=ORIENTED_EDGE('',*,*,#8629,.F.);
#13869=ORIENTED_EDGE('',*,*,#8483,.F.);
#13870=ORIENTED_EDGE('',*,*,#8487,.T.);
#13871=ORIENTED_EDGE('',*,*,#8406,.F.);
#13872=ORIENTED_EDGE('',*,*,#8645,.T.);
#13873=ORIENTED_EDGE('',*,*,#8641,.F.);
#13874=ORIENTED_EDGE('',*,*,#9726,.T.);
#13875=ORIENTED_EDGE('',*,*,#9618,.F.);
#13876=ORIENTED_EDGE('',*,*,#8480,.T.);
#13877=ORIENTED_EDGE('',*,*,#9726,.F.);
#13878=ORIENTED_EDGE('',*,*,#8640,.F.);
#13879=ORIENTED_EDGE('',*,*,#9617,.F.);
#13880=ORIENTED_EDGE('',*,*,#8493,.T.);
#13881=ORIENTED_EDGE('',*,*,#8583,.F.);
#13882=ORIENTED_EDGE('',*,*,#8490,.F.);
#13883=ORIENTED_EDGE('',*,*,#9616,.F.);
#13884=ORIENTED_EDGE('',*,*,#8507,.T.);
#13885=ORIENTED_EDGE('',*,*,#8582,.F.);
#13886=ORIENTED_EDGE('',*,*,#8504,.F.);
#13887=ORIENTED_EDGE('',*,*,#9615,.F.);
#13888=ORIENTED_EDGE('',*,*,#8521,.T.);
#13889=ORIENTED_EDGE('',*,*,#8581,.F.);
#13890=ORIENTED_EDGE('',*,*,#8518,.F.);
#13891=ORIENTED_EDGE('',*,*,#9614,.F.);
#13892=ORIENTED_EDGE('',*,*,#8535,.T.);
#13893=ORIENTED_EDGE('',*,*,#8580,.F.);
#13894=ORIENTED_EDGE('',*,*,#8532,.F.);
#13895=ORIENTED_EDGE('',*,*,#9613,.F.);
#13896=ORIENTED_EDGE('',*,*,#8549,.T.);
#13897=ORIENTED_EDGE('',*,*,#8579,.F.);
#13898=ORIENTED_EDGE('',*,*,#8546,.F.);
#13899=ORIENTED_EDGE('',*,*,#9612,.F.);
#13900=ORIENTED_EDGE('',*,*,#8561,.T.);
#13901=ORIENTED_EDGE('',*,*,#8578,.F.);
#13902=ORIENTED_EDGE('',*,*,#8571,.F.);
#13903=ORIENTED_EDGE('',*,*,#9611,.F.);
#13904=ORIENTED_EDGE('',*,*,#8444,.T.);
#13905=ORIENTED_EDGE('',*,*,#8442,.F.);
#13906=ORIENTED_EDGE('',*,*,#8435,.F.);
#13907=ORIENTED_EDGE('',*,*,#9610,.F.);
#13908=ORIENTED_EDGE('',*,*,#8458,.T.);
#13909=ORIENTED_EDGE('',*,*,#8456,.F.);
#13910=ORIENTED_EDGE('',*,*,#8449,.F.);
#13911=ORIENTED_EDGE('',*,*,#9609,.F.);
#13912=ORIENTED_EDGE('',*,*,#8479,.T.);
#13913=ORIENTED_EDGE('',*,*,#8470,.F.);
#13914=ORIENTED_EDGE('',*,*,#8463,.F.);
#13915=ORIENTED_EDGE('',*,*,#9608,.F.);
#13916=ORIENTED_EDGE('',*,*,#8065,.T.);
#13917=ORIENTED_EDGE('',*,*,#8070,.F.);
#13918=ORIENTED_EDGE('',*,*,#8474,.F.);
#13919=ORIENTED_EDGE('',*,*,#9607,.F.);
#13920=ORIENTED_EDGE('',*,*,#8083,.T.);
#13921=ORIENTED_EDGE('',*,*,#8088,.F.);
#13922=ORIENTED_EDGE('',*,*,#8055,.F.);
#13923=ORIENTED_EDGE('',*,*,#9605,.F.);
#13924=ORIENTED_EDGE('',*,*,#8104,.T.);
#13925=ORIENTED_EDGE('',*,*,#8081,.F.);
#13926=ORIENTED_EDGE('',*,*,#8073,.F.);
#13927=ORIENTED_EDGE('',*,*,#9603,.F.);
#13928=ORIENTED_EDGE('',*,*,#8107,.T.);
#13929=ORIENTED_EDGE('',*,*,#8102,.F.);
#13930=ORIENTED_EDGE('',*,*,#8094,.F.);
#13931=ORIENTED_EDGE('',*,*,#9601,.F.);
#13932=ORIENTED_EDGE('',*,*,#9521,.T.);
#13933=ORIENTED_EDGE('',*,*,#8428,.F.);
#13934=ORIENTED_EDGE('',*,*,#8432,.F.);
#13935=ORIENTED_EDGE('',*,*,#9599,.F.);
#13936=ORIENTED_EDGE('',*,*,#9545,.T.);
#13937=ORIENTED_EDGE('',*,*,#9530,.F.);
#13938=ORIENTED_EDGE('',*,*,#9528,.F.);
#13939=ORIENTED_EDGE('',*,*,#9597,.F.);
#13940=ORIENTED_EDGE('',*,*,#9569,.T.);
#13941=ORIENTED_EDGE('',*,*,#9554,.F.);
#13942=ORIENTED_EDGE('',*,*,#9552,.F.);
#13943=ORIENTED_EDGE('',*,*,#9595,.F.);
#13944=ORIENTED_EDGE('',*,*,#9581,.T.);
#13945=ORIENTED_EDGE('',*,*,#9578,.F.);
#13946=ORIENTED_EDGE('',*,*,#9576,.F.);
#13947=ORIENTED_EDGE('',*,*,#9693,.F.);
#13948=ORIENTED_EDGE('',*,*,#9558,.T.);
#13949=ORIENTED_EDGE('',*,*,#9568,.F.);
#13950=ORIENTED_EDGE('',*,*,#9587,.F.);
#13951=ORIENTED_EDGE('',*,*,#9593,.F.);
#13952=ORIENTED_EDGE('',*,*,#9691,.F.);
#13953=ORIENTED_EDGE('',*,*,#9534,.T.);
#13954=ORIENTED_EDGE('',*,*,#9544,.F.);
#13955=ORIENTED_EDGE('',*,*,#9565,.F.);
#13956=ORIENTED_EDGE('',*,*,#9689,.F.);
#13957=ORIENTED_EDGE('',*,*,#8110,.T.);
#13958=ORIENTED_EDGE('',*,*,#8118,.F.);
#13959=ORIENTED_EDGE('',*,*,#9541,.F.);
#13960=ORIENTED_EDGE('',*,*,#9687,.F.);
#13961=ORIENTED_EDGE('',*,*,#9499,.T.);
#13962=ORIENTED_EDGE('',*,*,#9520,.F.);
#13963=ORIENTED_EDGE('',*,*,#9518,.F.);
#13964=ORIENTED_EDGE('',*,*,#9686,.F.);
#13965=ORIENTED_EDGE('',*,*,#8135,.T.);
#13966=ORIENTED_EDGE('',*,*,#9516,.F.);
#13967=ORIENTED_EDGE('',*,*,#8125,.F.);
#13968=ORIENTED_EDGE('',*,*,#9685,.F.);
#13969=ORIENTED_EDGE('',*,*,#8150,.T.);
#13970=ORIENTED_EDGE('',*,*,#9515,.F.);
#13971=ORIENTED_EDGE('',*,*,#8147,.F.);
#13972=ORIENTED_EDGE('',*,*,#9684,.F.);
#13973=ORIENTED_EDGE('',*,*,#8165,.T.);
#13974=ORIENTED_EDGE('',*,*,#9514,.F.);
#13975=ORIENTED_EDGE('',*,*,#8162,.F.);
#13976=ORIENTED_EDGE('',*,*,#9683,.F.);
#13977=ORIENTED_EDGE('',*,*,#8180,.T.);
#13978=ORIENTED_EDGE('',*,*,#9513,.F.);
#13979=ORIENTED_EDGE('',*,*,#8177,.F.);
#13980=ORIENTED_EDGE('',*,*,#9682,.F.);
#13981=ORIENTED_EDGE('',*,*,#8195,.T.);
#13982=ORIENTED_EDGE('',*,*,#9512,.F.);
#13983=ORIENTED_EDGE('',*,*,#8192,.F.);
#13984=ORIENTED_EDGE('',*,*,#9681,.F.);
#13985=ORIENTED_EDGE('',*,*,#8210,.T.);
#13986=ORIENTED_EDGE('',*,*,#9511,.F.);
#13987=ORIENTED_EDGE('',*,*,#8207,.F.);
#13988=ORIENTED_EDGE('',*,*,#9680,.F.);
#13989=ORIENTED_EDGE('',*,*,#8225,.T.);
#13990=ORIENTED_EDGE('',*,*,#9510,.F.);
#13991=ORIENTED_EDGE('',*,*,#8222,.F.);
#13992=ORIENTED_EDGE('',*,*,#9679,.F.);
#13993=ORIENTED_EDGE('',*,*,#8240,.T.);
#13994=ORIENTED_EDGE('',*,*,#9509,.F.);
#13995=ORIENTED_EDGE('',*,*,#8237,.F.);
#13996=ORIENTED_EDGE('',*,*,#9678,.F.);
#13997=ORIENTED_EDGE('',*,*,#9349,.T.);
#13998=ORIENTED_EDGE('',*,*,#9508,.F.);
#13999=ORIENTED_EDGE('',*,*,#8252,.F.);
#14000=ORIENTED_EDGE('',*,*,#9677,.F.);
#14001=ORIENTED_EDGE('',*,*,#9361,.T.);
#14002=ORIENTED_EDGE('',*,*,#9493,.F.);
#14003=ORIENTED_EDGE('',*,*,#9358,.F.);
#14004=ORIENTED_EDGE('',*,*,#9676,.F.);
#14005=ORIENTED_EDGE('',*,*,#9375,.T.);
#14006=ORIENTED_EDGE('',*,*,#9492,.F.);
#14007=ORIENTED_EDGE('',*,*,#9372,.F.);
#14008=ORIENTED_EDGE('',*,*,#9675,.F.);
#14009=ORIENTED_EDGE('',*,*,#9389,.T.);
#14010=ORIENTED_EDGE('',*,*,#9491,.F.);
#14011=ORIENTED_EDGE('',*,*,#9386,.F.);
#14012=ORIENTED_EDGE('',*,*,#9674,.F.);
#14013=ORIENTED_EDGE('',*,*,#9403,.T.);
#14014=ORIENTED_EDGE('',*,*,#9490,.F.);
#14015=ORIENTED_EDGE('',*,*,#9400,.F.);
#14016=ORIENTED_EDGE('',*,*,#9673,.F.);
#14017=ORIENTED_EDGE('',*,*,#9417,.T.);
#14018=ORIENTED_EDGE('',*,*,#9489,.F.);
#14019=ORIENTED_EDGE('',*,*,#9414,.F.);
#14020=ORIENTED_EDGE('',*,*,#9672,.F.);
#14021=ORIENTED_EDGE('',*,*,#9431,.T.);
#14022=ORIENTED_EDGE('',*,*,#9488,.F.);
#14023=ORIENTED_EDGE('',*,*,#9428,.F.);
#14024=ORIENTED_EDGE('',*,*,#9671,.F.);
#14025=ORIENTED_EDGE('',*,*,#9445,.T.);
#14026=ORIENTED_EDGE('',*,*,#9487,.F.);
#14027=ORIENTED_EDGE('',*,*,#9442,.F.);
#14028=ORIENTED_EDGE('',*,*,#9670,.F.);
#14029=ORIENTED_EDGE('',*,*,#9459,.T.);
#14030=ORIENTED_EDGE('',*,*,#9486,.F.);
#14031=ORIENTED_EDGE('',*,*,#9456,.F.);
#14032=ORIENTED_EDGE('',*,*,#9669,.F.);
#14033=ORIENTED_EDGE('',*,*,#9470,.T.);
#14034=ORIENTED_EDGE('',*,*,#9475,.F.);
#14035=ORIENTED_EDGE('',*,*,#9477,.F.);
#14036=ORIENTED_EDGE('',*,*,#9668,.F.);
#14037=ORIENTED_EDGE('',*,*,#9315,.T.);
#14038=ORIENTED_EDGE('',*,*,#9727,.F.);
#14039=ORIENTED_EDGE('',*,*,#8044,.F.);
#14040=ORIENTED_EDGE('',*,*,#8045,.F.);
#14041=ORIENTED_EDGE('',*,*,#9727,.T.);
#14042=ORIENTED_EDGE('',*,*,#9318,.F.);
#14043=ORIENTED_EDGE('',*,*,#9322,.T.);
#14044=ORIENTED_EDGE('',*,*,#8306,.F.);
#14045=ORIENTED_EDGE('',*,*,#8049,.T.);
#14046=ORIENTED_EDGE('',*,*,#9667,.F.);
#14047=ORIENTED_EDGE('',*,*,#9326,.T.);
#14048=ORIENTED_EDGE('',*,*,#9348,.F.);
#14049=ORIENTED_EDGE('',*,*,#9346,.F.);
#14050=ORIENTED_EDGE('',*,*,#9666,.F.);
#14051=ORIENTED_EDGE('',*,*,#9207,.T.);
#14052=ORIENTED_EDGE('',*,*,#9205,.F.);
#14053=ORIENTED_EDGE('',*,*,#9198,.F.);
#14054=ORIENTED_EDGE('',*,*,#9665,.F.);
#14055=ORIENTED_EDGE('',*,*,#9221,.T.);
#14056=ORIENTED_EDGE('',*,*,#9219,.F.);
#14057=ORIENTED_EDGE('',*,*,#9212,.F.);
#14058=ORIENTED_EDGE('',*,*,#9664,.F.);
#14059=ORIENTED_EDGE('',*,*,#9235,.T.);
#14060=ORIENTED_EDGE('',*,*,#9233,.F.);
#14061=ORIENTED_EDGE('',*,*,#9226,.F.);
#14062=ORIENTED_EDGE('',*,*,#9663,.F.);
#14063=ORIENTED_EDGE('',*,*,#9249,.T.);
#14064=ORIENTED_EDGE('',*,*,#9247,.F.);
#14065=ORIENTED_EDGE('',*,*,#9240,.F.);
#14066=ORIENTED_EDGE('',*,*,#9662,.F.);
#14067=ORIENTED_EDGE('',*,*,#9263,.T.);
#14068=ORIENTED_EDGE('',*,*,#9261,.F.);
#14069=ORIENTED_EDGE('',*,*,#9254,.F.);
#14070=ORIENTED_EDGE('',*,*,#9661,.F.);
#14071=ORIENTED_EDGE('',*,*,#9277,.T.);
#14072=ORIENTED_EDGE('',*,*,#9275,.F.);
#14073=ORIENTED_EDGE('',*,*,#9268,.F.);
#14074=ORIENTED_EDGE('',*,*,#9660,.F.);
#14075=ORIENTED_EDGE('',*,*,#9291,.T.);
#14076=ORIENTED_EDGE('',*,*,#9289,.F.);
#14077=ORIENTED_EDGE('',*,*,#9282,.F.);
#14078=ORIENTED_EDGE('',*,*,#9659,.F.);
#14079=ORIENTED_EDGE('',*,*,#9314,.T.);
#14080=ORIENTED_EDGE('',*,*,#9303,.F.);
#14081=ORIENTED_EDGE('',*,*,#9296,.F.);
#14082=ORIENTED_EDGE('',*,*,#9151,.F.);
#14083=ORIENTED_EDGE('',*,*,#9155,.T.);
#14084=ORIENTED_EDGE('',*,*,#8326,.F.);
#14085=ORIENTED_EDGE('',*,*,#9312,.T.);
#14086=ORIENTED_EDGE('',*,*,#9308,.F.);
#14087=ORIENTED_EDGE('',*,*,#9728,.T.);
#14088=ORIENTED_EDGE('',*,*,#9658,.F.);
#14089=ORIENTED_EDGE('',*,*,#9148,.T.);
#14090=ORIENTED_EDGE('',*,*,#9728,.F.);
#14091=ORIENTED_EDGE('',*,*,#9307,.F.);
#14092=ORIENTED_EDGE('',*,*,#9657,.F.);
#14093=ORIENTED_EDGE('',*,*,#9161,.T.);
#14094=ORIENTED_EDGE('',*,*,#9195,.F.);
#14095=ORIENTED_EDGE('',*,*,#9158,.F.);
#14096=ORIENTED_EDGE('',*,*,#9656,.F.);
#14097=ORIENTED_EDGE('',*,*,#9173,.T.);
#14098=ORIENTED_EDGE('',*,*,#9194,.F.);
#14099=ORIENTED_EDGE('',*,*,#9191,.F.);
#14100=ORIENTED_EDGE('',*,*,#9655,.F.);
#14101=ORIENTED_EDGE('',*,*,#9054,.T.);
#14102=ORIENTED_EDGE('',*,*,#9052,.F.);
#14103=ORIENTED_EDGE('',*,*,#9045,.F.);
#14104=ORIENTED_EDGE('',*,*,#9654,.F.);
#14105=ORIENTED_EDGE('',*,*,#9068,.T.);
#14106=ORIENTED_EDGE('',*,*,#9066,.F.);
#14107=ORIENTED_EDGE('',*,*,#9059,.F.);
#14108=ORIENTED_EDGE('',*,*,#9653,.F.);
#14109=ORIENTED_EDGE('',*,*,#9082,.T.);
#14110=ORIENTED_EDGE('',*,*,#9080,.F.);
#14111=ORIENTED_EDGE('',*,*,#9073,.F.);
#14112=ORIENTED_EDGE('',*,*,#9652,.F.);
#14113=ORIENTED_EDGE('',*,*,#9096,.T.);
#14114=ORIENTED_EDGE('',*,*,#9094,.F.);
#14115=ORIENTED_EDGE('',*,*,#9087,.F.);
#14116=ORIENTED_EDGE('',*,*,#9651,.F.);
#14117=ORIENTED_EDGE('',*,*,#9110,.T.);
#14118=ORIENTED_EDGE('',*,*,#9108,.F.);
#14119=ORIENTED_EDGE('',*,*,#9101,.F.);
#14120=ORIENTED_EDGE('',*,*,#9650,.F.);
#14121=ORIENTED_EDGE('',*,*,#9124,.T.);
#14122=ORIENTED_EDGE('',*,*,#9122,.F.);
#14123=ORIENTED_EDGE('',*,*,#9115,.F.);
#14124=ORIENTED_EDGE('',*,*,#9649,.F.);
#14125=ORIENTED_EDGE('',*,*,#9147,.T.);
#14126=ORIENTED_EDGE('',*,*,#9136,.F.);
#14127=ORIENTED_EDGE('',*,*,#9129,.F.);
#14128=ORIENTED_EDGE('',*,*,#8985,.F.);
#14129=ORIENTED_EDGE('',*,*,#8989,.T.);
#14130=ORIENTED_EDGE('',*,*,#8346,.F.);
#14131=ORIENTED_EDGE('',*,*,#9145,.T.);
#14132=ORIENTED_EDGE('',*,*,#9141,.F.);
#14133=ORIENTED_EDGE('',*,*,#9729,.T.);
#14134=ORIENTED_EDGE('',*,*,#9648,.F.);
#14135=ORIENTED_EDGE('',*,*,#8982,.T.);
#14136=ORIENTED_EDGE('',*,*,#9729,.F.);
#14137=ORIENTED_EDGE('',*,*,#9140,.F.);
#14138=ORIENTED_EDGE('',*,*,#9647,.F.);
#14139=ORIENTED_EDGE('',*,*,#8995,.T.);
#14140=ORIENTED_EDGE('',*,*,#9042,.F.);
#14141=ORIENTED_EDGE('',*,*,#8992,.F.);
#14142=ORIENTED_EDGE('',*,*,#9646,.F.);
#14143=ORIENTED_EDGE('',*,*,#9009,.T.);
#14144=ORIENTED_EDGE('',*,*,#9041,.F.);
#14145=ORIENTED_EDGE('',*,*,#9006,.F.);
#14146=ORIENTED_EDGE('',*,*,#9645,.F.);
#14147=ORIENTED_EDGE('',*,*,#9021,.T.);
#14148=ORIENTED_EDGE('',*,*,#9040,.F.);
#14149=ORIENTED_EDGE('',*,*,#9036,.F.);
#14150=ORIENTED_EDGE('',*,*,#9730,.F.);
#14151=ORIENTED_EDGE('',*,*,#9731,.T.);
#14152=ORIENTED_EDGE('',*,*,#9731,.F.);
#14153=ORIENTED_EDGE('',*,*,#9732,.F.);
#14154=ORIENTED_EDGE('',*,*,#9733,.T.);
#14155=ORIENTED_EDGE('',*,*,#9733,.F.);
#14156=ORIENTED_EDGE('',*,*,#9734,.F.);
#14157=ORIENTED_EDGE('',*,*,#9735,.T.);
#14158=ORIENTED_EDGE('',*,*,#9735,.F.);
#14159=ORIENTED_EDGE('',*,*,#9736,.F.);
#14160=ORIENTED_EDGE('',*,*,#9737,.T.);
#14161=ORIENTED_EDGE('',*,*,#9737,.F.);
#14162=ORIENTED_EDGE('',*,*,#9738,.F.);
#14163=ORIENTED_EDGE('',*,*,#9739,.T.);
#14164=ORIENTED_EDGE('',*,*,#9739,.F.);
#14165=ORIENTED_EDGE('',*,*,#9700,.F.);
#14166=ORIENTED_EDGE('',*,*,#9740,.T.);
#14167=ORIENTED_EDGE('',*,*,#9741,.F.);
#14168=ORIENTED_EDGE('',*,*,#9740,.F.);
#14169=ORIENTED_EDGE('',*,*,#9496,.T.);
#14170=ORIENTED_EDGE('',*,*,#9720,.T.);
#14171=ORIENTED_EDGE('',*,*,#9716,.T.);
#14172=ORIENTED_EDGE('',*,*,#9712,.T.);
#14173=ORIENTED_EDGE('',*,*,#9708,.T.);
#14174=ORIENTED_EDGE('',*,*,#9704,.T.);
#14175=ORIENTED_EDGE('',*,*,#9741,.T.);
#14176=ORIENTED_EDGE('',*,*,#9738,.T.);
#14177=ORIENTED_EDGE('',*,*,#9736,.T.);
#14178=ORIENTED_EDGE('',*,*,#9734,.T.);
#14179=ORIENTED_EDGE('',*,*,#9732,.T.);
#14180=ORIENTED_EDGE('',*,*,#9730,.T.);
#15672=PLANE('',#17324);
#15673=PLANE('',#17330);
#15674=PLANE('',#17336);
#15675=PLANE('',#17340);
#15676=PLANE('',#17346);
#15677=PLANE('',#17352);
#15678=PLANE('',#17358);
#15679=PLANE('',#17359);
#15680=PLANE('',#17360);
#15681=PLANE('',#17367);
#15682=PLANE('',#17373);
#15683=PLANE('',#17379);
#15684=PLANE('',#17380);
#15685=PLANE('',#17386);
#15686=PLANE('',#17387);
#15687=PLANE('',#17393);
#15688=PLANE('',#17394);
#15689=PLANE('',#17400);
#15690=PLANE('',#17401);
#15691=PLANE('',#17407);
#15692=PLANE('',#17408);
#15693=PLANE('',#17414);
#15694=PLANE('',#17415);
#15695=PLANE('',#17421);
#15696=PLANE('',#17422);
#15697=PLANE('',#17428);
#15698=PLANE('',#17441);
#15699=PLANE('',#17604);
#15700=PLANE('',#17605);
#15701=PLANE('',#17610);
#15702=PLANE('',#17611);
#15703=PLANE('',#17616);
#15704=PLANE('',#17617);
#15705=PLANE('',#17622);
#15706=PLANE('',#17627);
#15707=PLANE('',#17628);
#15708=PLANE('',#17633);
#15709=PLANE('',#17634);
#15710=PLANE('',#17639);
#15711=PLANE('',#17640);
#15712=PLANE('',#17645);
#15713=PLANE('',#17646);
#15714=PLANE('',#17651);
#15715=PLANE('',#17652);
#15716=PLANE('',#17657);
#15717=PLANE('',#17658);
#15718=PLANE('',#17663);
#15719=PLANE('',#17676);
#15720=PLANE('',#17699);
#15721=PLANE('',#17704);
#15722=PLANE('',#17707);
#15723=PLANE('',#17712);
#15724=PLANE('',#17713);
#15725=PLANE('',#17718);
#15726=PLANE('',#17719);
#15727=PLANE('',#17724);
#15728=PLANE('',#17729);
#15729=PLANE('',#17730);
#15730=PLANE('',#17735);
#15731=PLANE('',#17736);
#15732=PLANE('',#17741);
#15733=PLANE('',#17742);
#15734=PLANE('',#17747);
#15735=PLANE('',#17748);
#15736=PLANE('',#17753);
#15737=PLANE('',#17754);
#15738=PLANE('',#17759);
#15739=PLANE('',#17774);
#15740=PLANE('',#17793);
#15741=PLANE('',#17798);
#15742=PLANE('',#17799);
#15743=PLANE('',#17804);
#15744=PLANE('',#17805);
#15745=PLANE('',#17810);
#15746=PLANE('',#17811);
#15747=PLANE('',#17816);
#15748=PLANE('',#17817);
#15749=PLANE('',#17822);
#15750=PLANE('',#17827);
#15751=PLANE('',#17828);
#15752=PLANE('',#17833);
#15753=PLANE('',#17834);
#15754=PLANE('',#17839);
#15755=PLANE('',#17840);
#15756=PLANE('',#17845);
#15757=PLANE('',#17846);
#15758=PLANE('',#17851);
#15759=PLANE('',#17872);
#15760=PLANE('',#17887);
#15761=PLANE('',#17892);
#15762=PLANE('',#17895);
#15763=PLANE('',#17900);
#15764=PLANE('',#17901);
#15765=PLANE('',#17906);
#15766=PLANE('',#17907);
#15767=PLANE('',#17912);
#15768=PLANE('',#17913);
#15769=PLANE('',#17918);
#15770=PLANE('',#17919);
#15771=PLANE('',#17924);
#15772=PLANE('',#17929);
#15773=PLANE('',#17930);
#15774=PLANE('',#17935);
#15775=PLANE('',#17936);
#15776=PLANE('',#17941);
#15777=PLANE('',#17942);
#15778=PLANE('',#17947);
#15779=PLANE('',#17970);
#15780=PLANE('',#17981);
#15781=PLANE('',#17986);
#15782=PLANE('',#17987);
#15783=PLANE('',#17992);
#15784=PLANE('',#17993);
#15785=PLANE('',#17998);
#15786=PLANE('',#17999);
#15787=PLANE('',#18004);
#15788=PLANE('',#18005);
#15789=PLANE('',#18010);
#15790=PLANE('',#18011);
#15791=PLANE('',#18016);
#15792=PLANE('',#18017);
#15793=PLANE('',#18022);
#15794=PLANE('',#18027);
#15795=PLANE('',#18028);
#15796=PLANE('',#18033);
#15797=PLANE('',#18034);
#15798=PLANE('',#18039);
#15799=PLANE('',#18068);
#15800=PLANE('',#18075);
#15801=PLANE('',#18080);
#15802=PLANE('',#18081);
#15803=PLANE('',#18086);
#15804=PLANE('',#18087);
#15805=PLANE('',#18092);
#15806=PLANE('',#18093);
#15807=PLANE('',#18098);
#15808=PLANE('',#18099);
#15809=PLANE('',#18104);
#15810=PLANE('',#18105);
#15811=PLANE('',#18110);
#15812=PLANE('',#18111);
#15813=PLANE('',#18116);
#15814=PLANE('',#18117);
#15815=PLANE('',#18122);
#15816=PLANE('',#18127);
#15817=PLANE('',#18128);
#15818=PLANE('',#18133);
#15819=PLANE('',#18166);
#15820=PLANE('',#18169);
#15821=PLANE('',#18174);
#15822=PLANE('',#18175);
#15823=PLANE('',#18180);
#15824=PLANE('',#18181);
#15825=PLANE('',#18186);
#15826=PLANE('',#18187);
#15827=PLANE('',#18192);
#15828=PLANE('',#18193);
#15829=PLANE('',#18198);
#15830=PLANE('',#18199);
#15831=PLANE('',#18204);
#15832=PLANE('',#18205);
#15833=PLANE('',#18210);
#15834=PLANE('',#18211);
#15835=PLANE('',#18216);
#15836=PLANE('',#18217);
#15837=PLANE('',#18222);
#15838=PLANE('',#18227);
#15839=PLANE('',#18264);
#15840=PLANE('',#18299);
#15841=PLANE('',#18302);
#15842=PLANE('',#18305);
#15843=PLANE('',#18308);
#15844=PLANE('',#18311);
#15845=PLANE('',#18314);
#15846=PLANE('',#18317);
#15847=PLANE('',#18320);
#15848=PLANE('',#18323);
#15849=PLANE('',#18326);
#15850=PLANE('',#18329);
#15851=PLANE('',#18332);
#15852=PLANE('',#18335);
#15853=PLANE('',#18339);
#15854=PLANE('',#18446);
#15855=PLANE('',#18484);
#15856=PLANE('',#18485);
#15857=PLANE('',#18486);
#15858=PLANE('',#18487);
#15859=PLANE('',#18488);
#15860=PLANE('',#18489);
#15861=PLANE('',#18492);
#15862=PLANE('',#18493);
#15863=PLANE('',#18494);
#15864=PLANE('',#18495);
#15865=PLANE('',#18496);
#15866=PLANE('',#18497);
#15867=PLANE('',#18498);
#15868=PLANE('',#18499);
#15869=PLANE('',#18500);
#15870=PLANE('',#18501);
#15871=PLANE('',#18504);
#15872=PLANE('',#18505);
#15873=PLANE('',#18506);
#15874=PLANE('',#18507);
#15875=PLANE('',#18508);
#15876=PLANE('',#18509);
#15877=PLANE('',#18510);
#15878=PLANE('',#18511);
#15879=PLANE('',#18512);
#15880=PLANE('',#18513);
#15881=PLANE('',#18516);
#15882=PLANE('',#18517);
#15883=PLANE('',#18518);
#15884=PLANE('',#18519);
#15885=PLANE('',#18520);
#15886=PLANE('',#18521);
#15887=PLANE('',#18522);
#15888=PLANE('',#18523);
#15889=PLANE('',#18524);
#15890=PLANE('',#18525);
#15891=PLANE('',#18526);
#15892=PLANE('',#18527);
#15893=PLANE('',#18528);
#15894=PLANE('',#18529);
#15895=PLANE('',#18530);
#15896=PLANE('',#18531);
#15897=PLANE('',#18532);
#15898=PLANE('',#18533);
#15899=PLANE('',#18534);
#15900=PLANE('',#18535);
#15901=PLANE('',#18536);
#15902=PLANE('',#18537);
#15903=PLANE('',#18538);
#15904=PLANE('',#18539);
#15905=PLANE('',#18540);
#15906=PLANE('',#18541);
#15907=PLANE('',#18542);
#15908=PLANE('',#18543);
#15909=PLANE('',#18544);
#15910=PLANE('',#18545);
#15911=PLANE('',#18546);
#15912=PLANE('',#18547);
#15913=PLANE('',#18548);
#15914=PLANE('',#18549);
#15915=PLANE('',#18550);
#15916=PLANE('',#18551);
#15917=PLANE('',#18552);
#15918=PLANE('',#18553);
#15919=PLANE('',#18554);
#15920=PLANE('',#18555);
#15921=PLANE('',#18556);
#15922=PLANE('',#18559);
#15923=PLANE('',#18560);
#15924=PLANE('',#18561);
#15925=PLANE('',#18562);
#15926=PLANE('',#18563);
#15927=PLANE('',#18564);
#15928=PLANE('',#18565);
#15929=PLANE('',#18566);
#15930=PLANE('',#18567);
#15931=PLANE('',#18570);
#15932=PLANE('',#18571);
#15933=PLANE('',#18572);
#15934=PLANE('',#18573);
#15935=PLANE('',#18574);
#15936=PLANE('',#18575);
#15937=PLANE('',#18576);
#15938=PLANE('',#18577);
#15939=PLANE('',#18578);
#15940=PLANE('',#18579);
#15941=PLANE('',#18582);
#15942=PLANE('',#18583);
#15943=PLANE('',#18584);
#15944=PLANE('',#18585);
#15945=PLANE('',#18598);
#16161=ADVANCED_FACE('',(#2352),#15672,.T.);
#16162=ADVANCED_FACE('',(#2353),#146,.T.);
#16163=ADVANCED_FACE('',(#2354),#855,.T.);
#16164=ADVANCED_FACE('',(#2355),#15673,.T.);
#16165=ADVANCED_FACE('',(#2356),#147,.T.);
#16166=ADVANCED_FACE('',(#2357),#856,.T.);
#16167=ADVANCED_FACE('',(#2358),#15674,.T.);
#16168=ADVANCED_FACE('',(#2359),#148,.F.);
#16169=ADVANCED_FACE('',(#2360),#15675,.T.);
#16170=ADVANCED_FACE('',(#2361),#857,.F.);
#16171=ADVANCED_FACE('',(#2362),#149,.F.);
#16172=ADVANCED_FACE('',(#2363),#15676,.T.);
#16173=ADVANCED_FACE('',(#2364),#150,.F.);
#16174=ADVANCED_FACE('',(#2365),#858,.F.);
#16175=ADVANCED_FACE('',(#2366),#15677,.T.);
#16176=ADVANCED_FACE('',(#2367),#859,.F.);
#16177=ADVANCED_FACE('',(#2368),#151,.F.);
#16178=ADVANCED_FACE('',(#2369),#15678,.T.);
#16179=ADVANCED_FACE('',(#2370),#15679,.T.);
#16180=ADVANCED_FACE('',(#2371),#15680,.T.);
#16181=ADVANCED_FACE('',(#2372),#152,.F.);
#16182=ADVANCED_FACE('',(#2373),#860,.T.);
#16183=ADVANCED_FACE('',(#2374),#15681,.T.);
#16184=ADVANCED_FACE('',(#2375),#153,.T.);
#16185=ADVANCED_FACE('',(#2376),#861,.T.);
#16186=ADVANCED_FACE('',(#2377),#15682,.T.);
#16187=ADVANCED_FACE('',(#2378),#862,.T.);
#16188=ADVANCED_FACE('',(#2379),#154,.T.);
#16189=ADVANCED_FACE('',(#2380),#15683,.T.);
#16190=ADVANCED_FACE('',(#2381),#15684,.T.);
#16191=ADVANCED_FACE('',(#2382),#863,.T.);
#16192=ADVANCED_FACE('',(#2383),#155,.T.);
#16193=ADVANCED_FACE('',(#2384),#15685,.T.);
#16194=ADVANCED_FACE('',(#2385),#15686,.T.);
#16195=ADVANCED_FACE('',(#2386),#864,.T.);
#16196=ADVANCED_FACE('',(#2387),#156,.T.);
#16197=ADVANCED_FACE('',(#2388),#15687,.T.);
#16198=ADVANCED_FACE('',(#2389),#15688,.T.);
#16199=ADVANCED_FACE('',(#2390),#865,.T.);
#16200=ADVANCED_FACE('',(#2391),#157,.T.);
#16201=ADVANCED_FACE('',(#2392),#15689,.T.);
#16202=ADVANCED_FACE('',(#2393),#15690,.T.);
#16203=ADVANCED_FACE('',(#2394),#866,.T.);
#16204=ADVANCED_FACE('',(#2395),#158,.T.);
#16205=ADVANCED_FACE('',(#2396),#15691,.T.);
#16206=ADVANCED_FACE('',(#2397),#15692,.T.);
#16207=ADVANCED_FACE('',(#2398),#867,.T.);
#16208=ADVANCED_FACE('',(#2399),#159,.T.);
#16209=ADVANCED_FACE('',(#2400),#15693,.T.);
#16210=ADVANCED_FACE('',(#2401),#15694,.T.);
#16211=ADVANCED_FACE('',(#2402),#868,.T.);
#16212=ADVANCED_FACE('',(#2403),#160,.T.);
#16213=ADVANCED_FACE('',(#2404),#15695,.T.);
#16214=ADVANCED_FACE('',(#2405),#15696,.T.);
#16215=ADVANCED_FACE('',(#2406),#869,.T.);
#16216=ADVANCED_FACE('',(#2407),#161,.T.);
#16217=ADVANCED_FACE('',(#2408),#15697,.T.);
#16218=ADVANCED_FACE('',(#2409),#870,.F.);
#16219=ADVANCED_FACE('',(#2410),#871,.T.);
#16220=ADVANCED_FACE('',(#2411),#872,.T.);
#16221=ADVANCED_FACE('',(#2412),#873,.T.);
#16222=ADVANCED_FACE('',(#2413,#1443),#15698,.F.);
#16223=ADVANCED_FACE('',(#2414),#162,.F.);
#16224=ADVANCED_FACE('',(#2415),#15699,.T.);
#16225=ADVANCED_FACE('',(#2416),#15700,.T.);
#16226=ADVANCED_FACE('',(#2417),#874,.F.);
#16227=ADVANCED_FACE('',(#2418),#163,.F.);
#16228=ADVANCED_FACE('',(#2419),#15701,.T.);
#16229=ADVANCED_FACE('',(#2420),#15702,.T.);
#16230=ADVANCED_FACE('',(#2421),#875,.F.);
#16231=ADVANCED_FACE('',(#2422),#164,.F.);
#16232=ADVANCED_FACE('',(#2423),#15703,.T.);
#16233=ADVANCED_FACE('',(#2424),#15704,.T.);
#16234=ADVANCED_FACE('',(#2425),#876,.F.);
#16235=ADVANCED_FACE('',(#2426),#165,.F.);
#16236=ADVANCED_FACE('',(#2427),#15705,.T.);
#16237=ADVANCED_FACE('',(#2428),#166,.T.);
#16238=ADVANCED_FACE('',(#2429),#877,.T.);
#16239=ADVANCED_FACE('',(#2430),#15706,.T.);
#16240=ADVANCED_FACE('',(#2431),#15707,.T.);
#16241=ADVANCED_FACE('',(#2432),#878,.T.);
#16242=ADVANCED_FACE('',(#2433),#167,.T.);
#16243=ADVANCED_FACE('',(#2434),#15708,.T.);
#16244=ADVANCED_FACE('',(#2435),#15709,.T.);
#16245=ADVANCED_FACE('',(#2436),#879,.T.);
#16246=ADVANCED_FACE('',(#2437),#168,.T.);
#16247=ADVANCED_FACE('',(#2438),#15710,.T.);
#16248=ADVANCED_FACE('',(#2439),#15711,.T.);
#16249=ADVANCED_FACE('',(#2440),#880,.T.);
#16250=ADVANCED_FACE('',(#2441),#169,.T.);
#16251=ADVANCED_FACE('',(#2442),#15712,.T.);
#16252=ADVANCED_FACE('',(#2443),#15713,.T.);
#16253=ADVANCED_FACE('',(#2444),#881,.T.);
#16254=ADVANCED_FACE('',(#2445),#170,.T.);
#16255=ADVANCED_FACE('',(#2446),#15714,.T.);
#16256=ADVANCED_FACE('',(#2447),#15715,.T.);
#16257=ADVANCED_FACE('',(#2448),#882,.T.);
#16258=ADVANCED_FACE('',(#2449),#171,.T.);
#16259=ADVANCED_FACE('',(#2450),#15716,.T.);
#16260=ADVANCED_FACE('',(#2451),#15717,.T.);
#16261=ADVANCED_FACE('',(#2452),#883,.T.);
#16262=ADVANCED_FACE('',(#2453),#172,.T.);
#16263=ADVANCED_FACE('',(#2454),#15718,.T.);
#16264=ADVANCED_FACE('',(#2455),#884,.T.);
#16265=ADVANCED_FACE('',(#2456),#885,.T.);
#16266=ADVANCED_FACE('',(#2457),#886,.T.);
#16267=ADVANCED_FACE('',(#2458),#173,.T.);
#16268=ADVANCED_FACE('',(#2459),#174,.T.);
#16269=ADVANCED_FACE('',(#2460),#175,.T.);
#16270=ADVANCED_FACE('',(#2461),#15719,.T.);
#16271=ADVANCED_FACE('',(#2462),#887,.F.);
#16272=ADVANCED_FACE('',(#2463),#888,.F.);
#16273=ADVANCED_FACE('',(#2464),#889,.F.);
#16274=ADVANCED_FACE('',(#2465),#890,.F.);
#16275=ADVANCED_FACE('',(#2466),#891,.F.);
#16276=ADVANCED_FACE('',(#2467),#176,.F.);
#16277=ADVANCED_FACE('',(#2468),#177,.F.);
#16278=ADVANCED_FACE('',(#2469),#178,.F.);
#16279=ADVANCED_FACE('',(#2470),#179,.F.);
#16280=ADVANCED_FACE('',(#2471),#180,.F.);
#16281=ADVANCED_FACE('',(#2472),#181,.F.);
#16282=ADVANCED_FACE('',(#2473),#15720,.T.);
#16283=ADVANCED_FACE('',(#2474),#892,.F.);
#16284=ADVANCED_FACE('',(#2475),#182,.F.);
#16285=ADVANCED_FACE('',(#2476),#15721,.T.);
#16286=ADVANCED_FACE('',(#2477),#893,.T.);
#16287=ADVANCED_FACE('',(#2478),#15722,.T.);
#16288=ADVANCED_FACE('',(#2479),#894,.F.);
#16289=ADVANCED_FACE('',(#2480),#183,.F.);
#16290=ADVANCED_FACE('',(#2481),#15723,.T.);
#16291=ADVANCED_FACE('',(#2482),#15724,.T.);
#16292=ADVANCED_FACE('',(#2483),#895,.F.);
#16293=ADVANCED_FACE('',(#2484),#184,.F.);
#16294=ADVANCED_FACE('',(#2485),#15725,.T.);
#16295=ADVANCED_FACE('',(#2486),#15726,.T.);
#16296=ADVANCED_FACE('',(#2487),#896,.F.);
#16297=ADVANCED_FACE('',(#2488),#185,.F.);
#16298=ADVANCED_FACE('',(#2489),#15727,.T.);
#16299=ADVANCED_FACE('',(#2490),#186,.T.);
#16300=ADVANCED_FACE('',(#2491),#897,.T.);
#16301=ADVANCED_FACE('',(#2492),#15728,.T.);
#16302=ADVANCED_FACE('',(#2493),#15729,.T.);
#16303=ADVANCED_FACE('',(#2494),#898,.T.);
#16304=ADVANCED_FACE('',(#2495),#187,.T.);
#16305=ADVANCED_FACE('',(#2496),#15730,.T.);
#16306=ADVANCED_FACE('',(#2497),#15731,.T.);
#16307=ADVANCED_FACE('',(#2498),#899,.T.);
#16308=ADVANCED_FACE('',(#2499),#188,.T.);
#16309=ADVANCED_FACE('',(#2500),#15732,.T.);
#16310=ADVANCED_FACE('',(#2501),#15733,.T.);
#16311=ADVANCED_FACE('',(#2502),#900,.T.);
#16312=ADVANCED_FACE('',(#2503),#189,.T.);
#16313=ADVANCED_FACE('',(#2504),#15734,.T.);
#16314=ADVANCED_FACE('',(#2505),#15735,.T.);
#16315=ADVANCED_FACE('',(#2506),#901,.T.);
#16316=ADVANCED_FACE('',(#2507),#190,.T.);
#16317=ADVANCED_FACE('',(#2508),#15736,.T.);
#16318=ADVANCED_FACE('',(#2509),#15737,.T.);
#16319=ADVANCED_FACE('',(#2510),#902,.T.);
#16320=ADVANCED_FACE('',(#2511),#191,.T.);
#16321=ADVANCED_FACE('',(#2512),#15738,.T.);
#16322=ADVANCED_FACE('',(#2513),#903,.T.);
#16323=ADVANCED_FACE('',(#2514),#904,.T.);
#16324=ADVANCED_FACE('',(#2515),#905,.T.);
#16325=ADVANCED_FACE('',(#2516),#192,.T.);
#16326=ADVANCED_FACE('',(#2517),#193,.T.);
#16327=ADVANCED_FACE('',(#2518),#194,.T.);
#16328=ADVANCED_FACE('',(#2519),#195,.T.);
#16329=ADVANCED_FACE('',(#2520),#15739,.T.);
#16330=ADVANCED_FACE('',(#2521),#906,.F.);
#16331=ADVANCED_FACE('',(#2522),#907,.F.);
#16332=ADVANCED_FACE('',(#2523),#908,.F.);
#16333=ADVANCED_FACE('',(#2524),#909,.F.);
#16334=ADVANCED_FACE('',(#2525),#196,.F.);
#16335=ADVANCED_FACE('',(#2526),#197,.F.);
#16336=ADVANCED_FACE('',(#2527),#198,.F.);
#16337=ADVANCED_FACE('',(#2528),#199,.F.);
#16338=ADVANCED_FACE('',(#2529),#200,.F.);
#16339=ADVANCED_FACE('',(#2530),#15740,.T.);
#16340=ADVANCED_FACE('',(#2531),#910,.F.);
#16341=ADVANCED_FACE('',(#2532),#201,.F.);
#16342=ADVANCED_FACE('',(#2533),#15741,.T.);
#16343=ADVANCED_FACE('',(#2534),#15742,.T.);
#16344=ADVANCED_FACE('',(#2535),#911,.F.);
#16345=ADVANCED_FACE('',(#2536),#202,.F.);
#16346=ADVANCED_FACE('',(#2537),#15743,.T.);
#16347=ADVANCED_FACE('',(#2538),#15744,.T.);
#16348=ADVANCED_FACE('',(#2539),#912,.F.);
#16349=ADVANCED_FACE('',(#2540),#203,.F.);
#16350=ADVANCED_FACE('',(#2541),#15745,.T.);
#16351=ADVANCED_FACE('',(#2542),#15746,.T.);
#16352=ADVANCED_FACE('',(#2543),#913,.F.);
#16353=ADVANCED_FACE('',(#2544),#204,.F.);
#16354=ADVANCED_FACE('',(#2545),#15747,.T.);
#16355=ADVANCED_FACE('',(#2546),#15748,.T.);
#16356=ADVANCED_FACE('',(#2547),#914,.F.);
#16357=ADVANCED_FACE('',(#2548),#205,.F.);
#16358=ADVANCED_FACE('',(#2549),#15749,.T.);
#16359=ADVANCED_FACE('',(#2550),#206,.T.);
#16360=ADVANCED_FACE('',(#2551),#915,.T.);
#16361=ADVANCED_FACE('',(#2552),#15750,.T.);
#16362=ADVANCED_FACE('',(#2553),#15751,.T.);
#16363=ADVANCED_FACE('',(#2554),#916,.T.);
#16364=ADVANCED_FACE('',(#2555),#207,.T.);
#16365=ADVANCED_FACE('',(#2556),#15752,.T.);
#16366=ADVANCED_FACE('',(#2557),#15753,.T.);
#16367=ADVANCED_FACE('',(#2558),#917,.T.);
#16368=ADVANCED_FACE('',(#2559),#208,.T.);
#16369=ADVANCED_FACE('',(#2560),#15754,.T.);
#16370=ADVANCED_FACE('',(#2561),#15755,.T.);
#16371=ADVANCED_FACE('',(#2562),#918,.T.);
#16372=ADVANCED_FACE('',(#2563),#209,.T.);
#16373=ADVANCED_FACE('',(#2564),#15756,.T.);
#16374=ADVANCED_FACE('',(#2565),#15757,.T.);
#16375=ADVANCED_FACE('',(#2566),#919,.T.);
#16376=ADVANCED_FACE('',(#2567),#210,.T.);
#16377=ADVANCED_FACE('',(#2568),#15758,.T.);
#16378=ADVANCED_FACE('',(#2569),#920,.T.);
#16379=ADVANCED_FACE('',(#2570),#921,.T.);
#16380=ADVANCED_FACE('',(#2571),#922,.T.);
#16381=ADVANCED_FACE('',(#2572),#923,.T.);
#16382=ADVANCED_FACE('',(#2573),#924,.T.);
#16383=ADVANCED_FACE('',(#2574),#211,.T.);
#16384=ADVANCED_FACE('',(#2575),#212,.T.);
#16385=ADVANCED_FACE('',(#2576),#213,.T.);
#16386=ADVANCED_FACE('',(#2577),#214,.T.);
#16387=ADVANCED_FACE('',(#2578),#215,.T.);
#16388=ADVANCED_FACE('',(#2579),#15759,.T.);
#16389=ADVANCED_FACE('',(#2580),#925,.F.);
#16390=ADVANCED_FACE('',(#2581),#926,.F.);
#16391=ADVANCED_FACE('',(#2582),#927,.F.);
#16392=ADVANCED_FACE('',(#2583),#216,.F.);
#16393=ADVANCED_FACE('',(#2584),#217,.F.);
#16394=ADVANCED_FACE('',(#2585),#218,.F.);
#16395=ADVANCED_FACE('',(#2586),#219,.F.);
#16396=ADVANCED_FACE('',(#2587),#15760,.T.);
#16397=ADVANCED_FACE('',(#2588),#928,.F.);
#16398=ADVANCED_FACE('',(#2589),#220,.F.);
#16399=ADVANCED_FACE('',(#2590),#15761,.T.);
#16400=ADVANCED_FACE('',(#2591),#929,.T.);
#16401=ADVANCED_FACE('',(#2592),#15762,.T.);
#16402=ADVANCED_FACE('',(#2593),#930,.F.);
#16403=ADVANCED_FACE('',(#2594),#221,.F.);
#16404=ADVANCED_FACE('',(#2595),#15763,.T.);
#16405=ADVANCED_FACE('',(#2596),#15764,.T.);
#16406=ADVANCED_FACE('',(#2597),#931,.F.);
#16407=ADVANCED_FACE('',(#2598),#222,.F.);
#16408=ADVANCED_FACE('',(#2599),#15765,.T.);
#16409=ADVANCED_FACE('',(#2600),#15766,.T.);
#16410=ADVANCED_FACE('',(#2601),#932,.F.);
#16411=ADVANCED_FACE('',(#2602),#223,.F.);
#16412=ADVANCED_FACE('',(#2603),#15767,.T.);
#16413=ADVANCED_FACE('',(#2604),#15768,.T.);
#16414=ADVANCED_FACE('',(#2605),#933,.F.);
#16415=ADVANCED_FACE('',(#2606),#224,.F.);
#16416=ADVANCED_FACE('',(#2607),#15769,.T.);
#16417=ADVANCED_FACE('',(#2608),#15770,.T.);
#16418=ADVANCED_FACE('',(#2609),#934,.F.);
#16419=ADVANCED_FACE('',(#2610),#225,.F.);
#16420=ADVANCED_FACE('',(#2611),#15771,.T.);
#16421=ADVANCED_FACE('',(#2612),#226,.T.);
#16422=ADVANCED_FACE('',(#2613),#935,.T.);
#16423=ADVANCED_FACE('',(#2614),#15772,.T.);
#16424=ADVANCED_FACE('',(#2615),#15773,.T.);
#16425=ADVANCED_FACE('',(#2616),#936,.T.);
#16426=ADVANCED_FACE('',(#2617),#227,.T.);
#16427=ADVANCED_FACE('',(#2618),#15774,.T.);
#16428=ADVANCED_FACE('',(#2619),#15775,.T.);
#16429=ADVANCED_FACE('',(#2620),#937,.T.);
#16430=ADVANCED_FACE('',(#2621),#228,.T.);
#16431=ADVANCED_FACE('',(#2622),#15776,.T.);
#16432=ADVANCED_FACE('',(#2623),#15777,.T.);
#16433=ADVANCED_FACE('',(#2624),#938,.T.);
#16434=ADVANCED_FACE('',(#2625),#229,.T.);
#16435=ADVANCED_FACE('',(#2626),#15778,.T.);
#16436=ADVANCED_FACE('',(#2627),#939,.T.);
#16437=ADVANCED_FACE('',(#2628),#940,.T.);
#16438=ADVANCED_FACE('',(#2629),#941,.T.);
#16439=ADVANCED_FACE('',(#2630),#942,.T.);
#16440=ADVANCED_FACE('',(#2631),#943,.T.);
#16441=ADVANCED_FACE('',(#2632),#230,.T.);
#16442=ADVANCED_FACE('',(#2633),#231,.T.);
#16443=ADVANCED_FACE('',(#2634),#232,.T.);
#16444=ADVANCED_FACE('',(#2635),#233,.T.);
#16445=ADVANCED_FACE('',(#2636),#234,.T.);
#16446=ADVANCED_FACE('',(#2637),#235,.T.);
#16447=ADVANCED_FACE('',(#2638),#15779,.T.);
#16448=ADVANCED_FACE('',(#2639),#944,.F.);
#16449=ADVANCED_FACE('',(#2640),#945,.F.);
#16450=ADVANCED_FACE('',(#2641),#236,.F.);
#16451=ADVANCED_FACE('',(#2642),#237,.F.);
#16452=ADVANCED_FACE('',(#2643),#238,.F.);
#16453=ADVANCED_FACE('',(#2644),#15780,.T.);
#16454=ADVANCED_FACE('',(#2645),#946,.F.);
#16455=ADVANCED_FACE('',(#2646),#239,.F.);
#16456=ADVANCED_FACE('',(#2647),#15781,.T.);
#16457=ADVANCED_FACE('',(#2648),#15782,.T.);
#16458=ADVANCED_FACE('',(#2649),#947,.F.);
#16459=ADVANCED_FACE('',(#2650),#240,.F.);
#16460=ADVANCED_FACE('',(#2651),#15783,.T.);
#16461=ADVANCED_FACE('',(#2652),#15784,.T.);
#16462=ADVANCED_FACE('',(#2653),#948,.F.);
#16463=ADVANCED_FACE('',(#2654),#241,.F.);
#16464=ADVANCED_FACE('',(#2655),#15785,.T.);
#16465=ADVANCED_FACE('',(#2656),#15786,.T.);
#16466=ADVANCED_FACE('',(#2657),#949,.F.);
#16467=ADVANCED_FACE('',(#2658),#242,.F.);
#16468=ADVANCED_FACE('',(#2659),#15787,.T.);
#16469=ADVANCED_FACE('',(#2660),#15788,.T.);
#16470=ADVANCED_FACE('',(#2661),#950,.F.);
#16471=ADVANCED_FACE('',(#2662),#243,.F.);
#16472=ADVANCED_FACE('',(#2663),#15789,.T.);
#16473=ADVANCED_FACE('',(#2664),#15790,.T.);
#16474=ADVANCED_FACE('',(#2665),#951,.F.);
#16475=ADVANCED_FACE('',(#2666),#244,.F.);
#16476=ADVANCED_FACE('',(#2667),#15791,.T.);
#16477=ADVANCED_FACE('',(#2668),#15792,.T.);
#16478=ADVANCED_FACE('',(#2669),#952,.F.);
#16479=ADVANCED_FACE('',(#2670),#245,.F.);
#16480=ADVANCED_FACE('',(#2671),#15793,.T.);
#16481=ADVANCED_FACE('',(#2672),#246,.T.);
#16482=ADVANCED_FACE('',(#2673),#953,.T.);
#16483=ADVANCED_FACE('',(#2674),#15794,.T.);
#16484=ADVANCED_FACE('',(#2675),#15795,.T.);
#16485=ADVANCED_FACE('',(#2676),#954,.T.);
#16486=ADVANCED_FACE('',(#2677),#247,.T.);
#16487=ADVANCED_FACE('',(#2678),#15796,.T.);
#16488=ADVANCED_FACE('',(#2679),#15797,.T.);
#16489=ADVANCED_FACE('',(#2680),#955,.T.);
#16490=ADVANCED_FACE('',(#2681),#248,.T.);
#16491=ADVANCED_FACE('',(#2682),#15798,.T.);
#16492=ADVANCED_FACE('',(#2683),#956,.T.);
#16493=ADVANCED_FACE('',(#2684),#957,.T.);
#16494=ADVANCED_FACE('',(#2685),#958,.T.);
#16495=ADVANCED_FACE('',(#2686),#959,.T.);
#16496=ADVANCED_FACE('',(#2687),#960,.T.);
#16497=ADVANCED_FACE('',(#2688),#961,.T.);
#16498=ADVANCED_FACE('',(#2689),#962,.T.);
#16499=ADVANCED_FACE('',(#2690),#249,.T.);
#16500=ADVANCED_FACE('',(#2691),#250,.T.);
#16501=ADVANCED_FACE('',(#2692),#251,.T.);
#16502=ADVANCED_FACE('',(#2693),#252,.T.);
#16503=ADVANCED_FACE('',(#2694),#253,.T.);
#16504=ADVANCED_FACE('',(#2695),#254,.T.);
#16505=ADVANCED_FACE('',(#2696),#255,.T.);
#16506=ADVANCED_FACE('',(#2697),#15799,.T.);
#16507=ADVANCED_FACE('',(#2698),#963,.F.);
#16508=ADVANCED_FACE('',(#2699),#256,.F.);
#16509=ADVANCED_FACE('',(#2700),#257,.F.);
#16510=ADVANCED_FACE('',(#2701),#15800,.T.);
#16511=ADVANCED_FACE('',(#2702),#964,.F.);
#16512=ADVANCED_FACE('',(#2703),#258,.F.);
#16513=ADVANCED_FACE('',(#2704),#15801,.T.);
#16514=ADVANCED_FACE('',(#2705),#15802,.T.);
#16515=ADVANCED_FACE('',(#2706),#965,.F.);
#16516=ADVANCED_FACE('',(#2707),#259,.F.);
#16517=ADVANCED_FACE('',(#2708),#15803,.T.);
#16518=ADVANCED_FACE('',(#2709),#15804,.T.);
#16519=ADVANCED_FACE('',(#2710),#966,.F.);
#16520=ADVANCED_FACE('',(#2711),#260,.F.);
#16521=ADVANCED_FACE('',(#2712),#15805,.T.);
#16522=ADVANCED_FACE('',(#2713),#15806,.T.);
#16523=ADVANCED_FACE('',(#2714),#967,.F.);
#16524=ADVANCED_FACE('',(#2715),#261,.F.);
#16525=ADVANCED_FACE('',(#2716),#15807,.T.);
#16526=ADVANCED_FACE('',(#2717),#15808,.T.);
#16527=ADVANCED_FACE('',(#2718),#968,.F.);
#16528=ADVANCED_FACE('',(#2719),#262,.F.);
#16529=ADVANCED_FACE('',(#2720),#15809,.T.);
#16530=ADVANCED_FACE('',(#2721),#15810,.T.);
#16531=ADVANCED_FACE('',(#2722),#969,.F.);
#16532=ADVANCED_FACE('',(#2723),#263,.F.);
#16533=ADVANCED_FACE('',(#2724),#15811,.T.);
#16534=ADVANCED_FACE('',(#2725),#15812,.T.);
#16535=ADVANCED_FACE('',(#2726),#970,.F.);
#16536=ADVANCED_FACE('',(#2727),#264,.F.);
#16537=ADVANCED_FACE('',(#2728),#15813,.T.);
#16538=ADVANCED_FACE('',(#2729),#15814,.T.);
#16539=ADVANCED_FACE('',(#2730),#971,.F.);
#16540=ADVANCED_FACE('',(#2731),#265,.F.);
#16541=ADVANCED_FACE('',(#2732),#15815,.T.);
#16542=ADVANCED_FACE('',(#2733),#266,.T.);
#16543=ADVANCED_FACE('',(#2734),#972,.T.);
#16544=ADVANCED_FACE('',(#2735),#15816,.T.);
#16545=ADVANCED_FACE('',(#2736),#15817,.T.);
#16546=ADVANCED_FACE('',(#2737),#973,.T.);
#16547=ADVANCED_FACE('',(#2738),#267,.T.);
#16548=ADVANCED_FACE('',(#2739),#15818,.T.);
#16549=ADVANCED_FACE('',(#2740),#974,.T.);
#16550=ADVANCED_FACE('',(#2741),#975,.T.);
#16551=ADVANCED_FACE('',(#2742),#976,.T.);
#16552=ADVANCED_FACE('',(#2743),#977,.T.);
#16553=ADVANCED_FACE('',(#2744),#978,.T.);
#16554=ADVANCED_FACE('',(#2745),#979,.T.);
#16555=ADVANCED_FACE('',(#2746),#980,.T.);
#16556=ADVANCED_FACE('',(#2747),#981,.T.);
#16557=ADVANCED_FACE('',(#2748),#268,.T.);
#16558=ADVANCED_FACE('',(#2749),#269,.T.);
#16559=ADVANCED_FACE('',(#2750),#270,.T.);
#16560=ADVANCED_FACE('',(#2751),#271,.T.);
#16561=ADVANCED_FACE('',(#2752),#272,.T.);
#16562=ADVANCED_FACE('',(#2753),#273,.T.);
#16563=ADVANCED_FACE('',(#2754),#274,.T.);
#16564=ADVANCED_FACE('',(#2755),#275,.T.);
#16565=ADVANCED_FACE('',(#2756),#15819,.T.);
#16566=ADVANCED_FACE('',(#2757),#276,.F.);
#16567=ADVANCED_FACE('',(#2758),#15820,.T.);
#16568=ADVANCED_FACE('',(#2759),#982,.T.);
#16569=ADVANCED_FACE('',(#2760),#277,.T.);
#16570=ADVANCED_FACE('',(#2761),#15821,.T.);
#16571=ADVANCED_FACE('',(#2762),#15822,.T.);
#16572=ADVANCED_FACE('',(#2763),#983,.T.);
#16573=ADVANCED_FACE('',(#2764),#278,.T.);
#16574=ADVANCED_FACE('',(#2765),#15823,.T.);
#16575=ADVANCED_FACE('',(#2766),#15824,.T.);
#16576=ADVANCED_FACE('',(#2767),#984,.T.);
#16577=ADVANCED_FACE('',(#2768),#279,.T.);
#16578=ADVANCED_FACE('',(#2769),#15825,.T.);
#16579=ADVANCED_FACE('',(#2770),#15826,.T.);
#16580=ADVANCED_FACE('',(#2771),#985,.T.);
#16581=ADVANCED_FACE('',(#2772),#280,.T.);
#16582=ADVANCED_FACE('',(#2773),#15827,.T.);
#16583=ADVANCED_FACE('',(#2774),#15828,.T.);
#16584=ADVANCED_FACE('',(#2775),#986,.T.);
#16585=ADVANCED_FACE('',(#2776),#281,.T.);
#16586=ADVANCED_FACE('',(#2777),#15829,.T.);
#16587=ADVANCED_FACE('',(#2778),#15830,.T.);
#16588=ADVANCED_FACE('',(#2779),#987,.T.);
#16589=ADVANCED_FACE('',(#2780),#282,.T.);
#16590=ADVANCED_FACE('',(#2781),#15831,.T.);
#16591=ADVANCED_FACE('',(#2782),#15832,.T.);
#16592=ADVANCED_FACE('',(#2783),#988,.T.);
#16593=ADVANCED_FACE('',(#2784),#283,.T.);
#16594=ADVANCED_FACE('',(#2785),#15833,.T.);
#16595=ADVANCED_FACE('',(#2786),#15834,.T.);
#16596=ADVANCED_FACE('',(#2787),#989,.T.);
#16597=ADVANCED_FACE('',(#2788),#284,.T.);
#16598=ADVANCED_FACE('',(#2789),#15835,.T.);
#16599=ADVANCED_FACE('',(#2790),#15836,.T.);
#16600=ADVANCED_FACE('',(#2791),#990,.T.);
#16601=ADVANCED_FACE('',(#2792),#285,.T.);
#16602=ADVANCED_FACE('',(#2793),#15837,.T.);
#16603=ADVANCED_FACE('',(#2794),#286,.F.);
#16604=ADVANCED_FACE('',(#2795),#991,.F.);
#16605=ADVANCED_FACE('',(#2796),#15838,.T.);
#16606=ADVANCED_FACE('',(#2797),#992,.F.);
#16607=ADVANCED_FACE('',(#2798),#993,.F.);
#16608=ADVANCED_FACE('',(#2799),#994,.F.);
#16609=ADVANCED_FACE('',(#2800),#995,.F.);
#16610=ADVANCED_FACE('',(#2801),#996,.F.);
#16611=ADVANCED_FACE('',(#2802),#997,.F.);
#16612=ADVANCED_FACE('',(#2803),#998,.F.);
#16613=ADVANCED_FACE('',(#2804),#999,.F.);
#16614=ADVANCED_FACE('',(#2805),#287,.F.);
#16615=ADVANCED_FACE('',(#2806),#288,.F.);
#16616=ADVANCED_FACE('',(#2807),#289,.F.);
#16617=ADVANCED_FACE('',(#2808),#290,.F.);
#16618=ADVANCED_FACE('',(#2809),#291,.F.);
#16619=ADVANCED_FACE('',(#2810),#292,.F.);
#16620=ADVANCED_FACE('',(#2811),#293,.F.);
#16621=ADVANCED_FACE('',(#2812),#294,.F.);
#16622=ADVANCED_FACE('',(#2813),#1000,.F.);
#16623=ADVANCED_FACE('',(#2814),#295,.F.);
#16624=ADVANCED_FACE('',(#2815),#15839,.T.);
#16625=ADVANCED_FACE('',(#2816),#1001,.F.);
#16626=ADVANCED_FACE('',(#2817),#1002,.F.);
#16627=ADVANCED_FACE('',(#2818),#1003,.F.);
#16628=ADVANCED_FACE('',(#2819),#1004,.F.);
#16629=ADVANCED_FACE('',(#2820),#1005,.F.);
#16630=ADVANCED_FACE('',(#2821),#1006,.F.);
#16631=ADVANCED_FACE('',(#2822),#1007,.F.);
#16632=ADVANCED_FACE('',(#2823),#1008,.F.);
#16633=ADVANCED_FACE('',(#2824),#296,.F.);
#16634=ADVANCED_FACE('',(#2825),#297,.F.);
#16635=ADVANCED_FACE('',(#2826),#298,.F.);
#16636=ADVANCED_FACE('',(#2827),#299,.F.);
#16637=ADVANCED_FACE('',(#2828),#300,.F.);
#16638=ADVANCED_FACE('',(#2829),#301,.F.);
#16639=ADVANCED_FACE('',(#2830),#302,.F.);
#16640=ADVANCED_FACE('',(#2831),#303,.F.);
#16641=ADVANCED_FACE('',(#2832),#304,.F.);
#16642=ADVANCED_FACE('',(#2833),#15840,.T.);
#16643=ADVANCED_FACE('',(#2834),#305,.F.);
#16644=ADVANCED_FACE('',(#2835),#15841,.T.);
#16645=ADVANCED_FACE('',(#2836),#1009,.T.);
#16646=ADVANCED_FACE('',(#2837),#15842,.T.);
#16647=ADVANCED_FACE('',(#2838),#306,.F.);
#16648=ADVANCED_FACE('',(#2839),#15843,.T.);
#16649=ADVANCED_FACE('',(#2840),#1010,.T.);
#16650=ADVANCED_FACE('',(#2841),#15844,.T.);
#16651=ADVANCED_FACE('',(#2842),#307,.F.);
#16652=ADVANCED_FACE('',(#2843),#15845,.T.);
#16653=ADVANCED_FACE('',(#2844),#1011,.T.);
#16654=ADVANCED_FACE('',(#2845),#15846,.T.);
#16655=ADVANCED_FACE('',(#2846),#308,.F.);
#16656=ADVANCED_FACE('',(#2847),#15847,.T.);
#16657=ADVANCED_FACE('',(#2848),#1012,.T.);
#16658=ADVANCED_FACE('',(#2849),#15848,.T.);
#16659=ADVANCED_FACE('',(#2850),#309,.F.);
#16660=ADVANCED_FACE('',(#2851),#15849,.T.);
#16661=ADVANCED_FACE('',(#2852),#1013,.T.);
#16662=ADVANCED_FACE('',(#2853),#15850,.T.);
#16663=ADVANCED_FACE('',(#2854),#310,.F.);
#16664=ADVANCED_FACE('',(#2855),#15851,.T.);
#16665=ADVANCED_FACE('',(#2856),#1014,.T.);
#16666=ADVANCED_FACE('',(#2857),#15852,.T.);
#16667=ADVANCED_FACE('',(#2858),#1015,.T.);
#16668=ADVANCED_FACE('',(#2859,#1444),#15853,.T.);
#16669=ADVANCED_FACE('',(#2860),#1016,.T.);
#16670=ADVANCED_FACE('',(#2861),#1017,.F.);
#16671=ADVANCED_FACE('',(#2862,#1445,#1446,#1447,#1448,#1449,#1450),#15854,
 .T.);
#16672=ADVANCED_FACE('',(#2863),#311,.F.);
#16673=ADVANCED_FACE('',(#2864),#1018,.F.);
#16674=ADVANCED_FACE('',(#2865),#312,.F.);
#16675=ADVANCED_FACE('',(#2866),#1019,.F.);
#16676=ADVANCED_FACE('',(#2867),#313,.F.);
#16677=ADVANCED_FACE('',(#2868),#1020,.F.);
#16678=ADVANCED_FACE('',(#2869),#314,.F.);
#16679=ADVANCED_FACE('',(#2870),#1021,.F.);
#16680=ADVANCED_FACE('',(#2871),#315,.F.);
#16681=ADVANCED_FACE('',(#2872),#1022,.F.);
#16682=ADVANCED_FACE('',(#2873),#316,.F.);
#16683=ADVANCED_FACE('',(#2874),#317,.T.);
#16684=ADVANCED_FACE('',(#2875),#318,.T.);
#16685=ADVANCED_FACE('',(#2876),#319,.T.);
#16686=ADVANCED_FACE('',(#2877),#320,.T.);
#16687=ADVANCED_FACE('',(#2878),#321,.T.);
#16688=ADVANCED_FACE('',(#2879),#322,.T.);
#16689=ADVANCED_FACE('',(#2880),#323,.T.);
#16690=ADVANCED_FACE('',(#2881),#324,.T.);
#16691=ADVANCED_FACE('',(#2882),#325,.T.);
#16692=ADVANCED_FACE('',(#2883),#326,.T.);
#16693=ADVANCED_FACE('',(#2884),#15855,.F.);
#16694=ADVANCED_FACE('',(#2885),#15856,.F.);
#16695=ADVANCED_FACE('',(#2886),#15857,.F.);
#16696=ADVANCED_FACE('',(#2887),#15858,.F.);
#16697=ADVANCED_FACE('',(#2888),#15859,.F.);
#16698=ADVANCED_FACE('',(#2889),#15860,.F.);
#16699=ADVANCED_FACE('',(#2890),#327,.F.);
#16700=ADVANCED_FACE('',(#2891),#15861,.F.);
#16701=ADVANCED_FACE('',(#2892),#15862,.F.);
#16702=ADVANCED_FACE('',(#2893),#15863,.F.);
#16703=ADVANCED_FACE('',(#2894),#15864,.F.);
#16704=ADVANCED_FACE('',(#2895),#15865,.F.);
#16705=ADVANCED_FACE('',(#2896),#15866,.F.);
#16706=ADVANCED_FACE('',(#2897),#15867,.F.);
#16707=ADVANCED_FACE('',(#2898),#15868,.F.);
#16708=ADVANCED_FACE('',(#2899),#15869,.F.);
#16709=ADVANCED_FACE('',(#2900),#15870,.F.);
#16710=ADVANCED_FACE('',(#2901),#328,.F.);
#16711=ADVANCED_FACE('',(#2902),#15871,.F.);
#16712=ADVANCED_FACE('',(#2903),#15872,.F.);
#16713=ADVANCED_FACE('',(#2904),#15873,.F.);
#16714=ADVANCED_FACE('',(#2905),#15874,.F.);
#16715=ADVANCED_FACE('',(#2906),#15875,.F.);
#16716=ADVANCED_FACE('',(#2907),#15876,.F.);
#16717=ADVANCED_FACE('',(#2908),#15877,.F.);
#16718=ADVANCED_FACE('',(#2909),#15878,.F.);
#16719=ADVANCED_FACE('',(#2910),#15879,.F.);
#16720=ADVANCED_FACE('',(#2911),#15880,.F.);
#16721=ADVANCED_FACE('',(#2912),#329,.F.);
#16722=ADVANCED_FACE('',(#2913),#15881,.F.);
#16723=ADVANCED_FACE('',(#2914),#15882,.F.);
#16724=ADVANCED_FACE('',(#2915),#15883,.F.);
#16725=ADVANCED_FACE('',(#2916),#15884,.F.);
#16726=ADVANCED_FACE('',(#2917),#15885,.F.);
#16727=ADVANCED_FACE('',(#2918),#15886,.F.);
#16728=ADVANCED_FACE('',(#2919),#15887,.F.);
#16729=ADVANCED_FACE('',(#2920),#15888,.F.);
#16730=ADVANCED_FACE('',(#2921),#15889,.F.);
#16731=ADVANCED_FACE('',(#2922),#15890,.F.);
#16732=ADVANCED_FACE('',(#2923),#15891,.F.);
#16733=ADVANCED_FACE('',(#2924),#15892,.F.);
#16734=ADVANCED_FACE('',(#2925),#15893,.F.);
#16735=ADVANCED_FACE('',(#2926),#15894,.F.);
#16736=ADVANCED_FACE('',(#2927),#15895,.F.);
#16737=ADVANCED_FACE('',(#2928),#15896,.F.);
#16738=ADVANCED_FACE('',(#2929),#15897,.F.);
#16739=ADVANCED_FACE('',(#2930),#15898,.F.);
#16740=ADVANCED_FACE('',(#2931),#15899,.F.);
#16741=ADVANCED_FACE('',(#2932),#15900,.F.);
#16742=ADVANCED_FACE('',(#2933),#15901,.F.);
#16743=ADVANCED_FACE('',(#2934),#15902,.F.);
#16744=ADVANCED_FACE('',(#2935),#15903,.F.);
#16745=ADVANCED_FACE('',(#2936),#15904,.F.);
#16746=ADVANCED_FACE('',(#2937),#15905,.F.);
#16747=ADVANCED_FACE('',(#2938),#15906,.F.);
#16748=ADVANCED_FACE('',(#2939),#15907,.F.);
#16749=ADVANCED_FACE('',(#2940),#15908,.F.);
#16750=ADVANCED_FACE('',(#2941),#15909,.F.);
#16751=ADVANCED_FACE('',(#2942),#15910,.F.);
#16752=ADVANCED_FACE('',(#2943),#15911,.F.);
#16753=ADVANCED_FACE('',(#2944),#15912,.F.);
#16754=ADVANCED_FACE('',(#2945),#15913,.F.);
#16755=ADVANCED_FACE('',(#2946),#15914,.F.);
#16756=ADVANCED_FACE('',(#2947),#15915,.F.);
#16757=ADVANCED_FACE('',(#2948),#15916,.F.);
#16758=ADVANCED_FACE('',(#2949),#15917,.F.);
#16759=ADVANCED_FACE('',(#2950),#15918,.F.);
#16760=ADVANCED_FACE('',(#2951),#15919,.F.);
#16761=ADVANCED_FACE('',(#2952),#15920,.F.);
#16762=ADVANCED_FACE('',(#2953),#15921,.F.);
#16763=ADVANCED_FACE('',(#2954),#330,.F.);
#16764=ADVANCED_FACE('',(#2955),#15922,.F.);
#16765=ADVANCED_FACE('',(#2956),#15923,.F.);
#16766=ADVANCED_FACE('',(#2957),#15924,.F.);
#16767=ADVANCED_FACE('',(#2958),#15925,.F.);
#16768=ADVANCED_FACE('',(#2959),#15926,.F.);
#16769=ADVANCED_FACE('',(#2960),#15927,.F.);
#16770=ADVANCED_FACE('',(#2961),#15928,.F.);
#16771=ADVANCED_FACE('',(#2962),#15929,.F.);
#16772=ADVANCED_FACE('',(#2963),#15930,.F.);
#16773=ADVANCED_FACE('',(#2964),#331,.F.);
#16774=ADVANCED_FACE('',(#2965),#15931,.F.);
#16775=ADVANCED_FACE('',(#2966),#15932,.F.);
#16776=ADVANCED_FACE('',(#2967),#15933,.F.);
#16777=ADVANCED_FACE('',(#2968),#15934,.F.);
#16778=ADVANCED_FACE('',(#2969),#15935,.F.);
#16779=ADVANCED_FACE('',(#2970),#15936,.F.);
#16780=ADVANCED_FACE('',(#2971),#15937,.F.);
#16781=ADVANCED_FACE('',(#2972),#15938,.F.);
#16782=ADVANCED_FACE('',(#2973),#15939,.F.);
#16783=ADVANCED_FACE('',(#2974),#15940,.F.);
#16784=ADVANCED_FACE('',(#2975),#332,.F.);
#16785=ADVANCED_FACE('',(#2976),#15941,.F.);
#16786=ADVANCED_FACE('',(#2977),#15942,.F.);
#16787=ADVANCED_FACE('',(#2978),#15943,.F.);
#16788=ADVANCED_FACE('',(#2979),#15944,.F.);
#16789=ADVANCED_FACE('',(#2980),#1023,.F.);
#16790=ADVANCED_FACE('',(#2981),#1024,.F.);
#16791=ADVANCED_FACE('',(#2982),#1025,.F.);
#16792=ADVANCED_FACE('',(#2983),#1026,.F.);
#16793=ADVANCED_FACE('',(#2984),#1027,.F.);
#16794=ADVANCED_FACE('',(#2985),#333,.F.);
#16795=ADVANCED_FACE('',(#2986,#1451,#1452,#1453,#1454,#1455,#1456,#1457,
#1458,#1459,#1460,#1461),#15945,.F.);
#17073=CLOSED_SHELL('',(#16161,#16162,#16163,#16164,#16165,#16166,#16167,
#16168,#16169,#16170,#16171,#16172,#16173,#16174,#16175,#16176,#16177,#16178,
#16179,#16180,#16181,#16182,#16183,#16184,#16185,#16186,#16187,#16188,#16189,
#16190,#16191,#16192,#16193,#16194,#16195,#16196,#16197,#16198,#16199,#16200,
#16201,#16202,#16203,#16204,#16205,#16206,#16207,#16208,#16209,#16210,#16211,
#16212,#16213,#16214,#16215,#16216,#16217,#16218,#16219,#16220,#16221,#16222,
#16223,#16224,#16225,#16226,#16227,#16228,#16229,#16230,#16231,#16232,#16233,
#16234,#16235,#16236,#16237,#16238,#16239,#16240,#16241,#16242,#16243,#16244,
#16245,#16246,#16247,#16248,#16249,#16250,#16251,#16252,#16253,#16254,#16255,
#16256,#16257,#16258,#16259,#16260,#16261,#16262,#16263,#16264,#16265,#16266,
#16267,#16268,#16269,#16270,#16271,#16272,#16273,#16274,#16275,#16276,#16277,
#16278,#16279,#16280,#16281,#16282,#16283,#16284,#16285,#16286,#16287,#16288,
#16289,#16290,#16291,#16292,#16293,#16294,#16295,#16296,#16297,#16298,#16299,
#16300,#16301,#16302,#16303,#16304,#16305,#16306,#16307,#16308,#16309,#16310,
#16311,#16312,#16313,#16314,#16315,#16316,#16317,#16318,#16319,#16320,#16321,
#16322,#16323,#16324,#16325,#16326,#16327,#16328,#16329,#16330,#16331,#16332,
#16333,#16334,#16335,#16336,#16337,#16338,#16339,#16340,#16341,#16342,#16343,
#16344,#16345,#16346,#16347,#16348,#16349,#16350,#16351,#16352,#16353,#16354,
#16355,#16356,#16357,#16358,#16359,#16360,#16361,#16362,#16363,#16364,#16365,
#16366,#16367,#16368,#16369,#16370,#16371,#16372,#16373,#16374,#16375,#16376,
#16377,#16378,#16379,#16380,#16381,#16382,#16383,#16384,#16385,#16386,#16387,
#16388,#16389,#16390,#16391,#16392,#16393,#16394,#16395,#16396,#16397,#16398,
#16399,#16400,#16401,#16402,#16403,#16404,#16405,#16406,#16407,#16408,#16409,
#16410,#16411,#16412,#16413,#16414,#16415,#16416,#16417,#16418,#16419,#16420,
#16421,#16422,#16423,#16424,#16425,#16426,#16427,#16428,#16429,#16430,#16431,
#16432,#16433,#16434,#16435,#16436,#16437,#16438,#16439,#16440,#16441,#16442,
#16443,#16444,#16445,#16446,#16447,#16448,#16449,#16450,#16451,#16452,#16453,
#16454,#16455,#16456,#16457,#16458,#16459,#16460,#16461,#16462,#16463,#16464,
#16465,#16466,#16467,#16468,#16469,#16470,#16471,#16472,#16473,#16474,#16475,
#16476,#16477,#16478,#16479,#16480,#16481,#16482,#16483,#16484,#16485,#16486,
#16487,#16488,#16489,#16490,#16491,#16492,#16493,#16494,#16495,#16496,#16497,
#16498,#16499,#16500,#16501,#16502,#16503,#16504,#16505,#16506,#16507,#16508,
#16509,#16510,#16511,#16512,#16513,#16514,#16515,#16516,#16517,#16518,#16519,
#16520,#16521,#16522,#16523,#16524,#16525,#16526,#16527,#16528,#16529,#16530,
#16531,#16532,#16533,#16534,#16535,#16536,#16537,#16538,#16539,#16540,#16541,
#16542,#16543,#16544,#16545,#16546,#16547,#16548,#16549,#16550,#16551,#16552,
#16553,#16554,#16555,#16556,#16557,#16558,#16559,#16560,#16561,#16562,#16563,
#16564,#16565,#16566,#16567,#16568,#16569,#16570,#16571,#16572,#16573,#16574,
#16575,#16576,#16577,#16578,#16579,#16580,#16581,#16582,#16583,#16584,#16585,
#16586,#16587,#16588,#16589,#16590,#16591,#16592,#16593,#16594,#16595,#16596,
#16597,#16598,#16599,#16600,#16601,#16602,#16603,#16604,#16605,#16606,#16607,
#16608,#16609,#16610,#16611,#16612,#16613,#16614,#16615,#16616,#16617,#16618,
#16619,#16620,#16621,#16622,#16623,#16624,#16625,#16626,#16627,#16628,#16629,
#16630,#16631,#16632,#16633,#16634,#16635,#16636,#16637,#16638,#16639,#16640,
#16641,#16642,#16643,#16644,#16645,#16646,#16647,#16648,#16649,#16650,#16651,
#16652,#16653,#16654,#16655,#16656,#16657,#16658,#16659,#16660,#16661,#16662,
#16663,#16664,#16665,#16666,#16667,#16668,#16669,#16670,#16671,#16672,#16673,
#16674,#16675,#16676,#16677,#16678,#16679,#16680,#16681,#16682,#16683,#16684,
#16685,#16686,#16687,#16688,#16689,#16690,#16691,#16692,#16693,#16694,#16695,
#16696,#16697,#16698,#16699,#16700,#16701,#16702,#16703,#16704,#16705,#16706,
#16707,#16708,#16709,#16710,#16711,#16712,#16713,#16714,#16715,#16716,#16717,
#16718,#16719,#16720,#16721,#16722,#16723,#16724,#16725,#16726,#16727,#16728,
#16729,#16730,#16731,#16732,#16733,#16734,#16735,#16736,#16737,#16738,#16739,
#16740,#16741,#16742,#16743,#16744,#16745,#16746,#16747,#16748,#16749,#16750,
#16751,#16752,#16753,#16754,#16755,#16756,#16757,#16758,#16759,#16760,#16761,
#16762,#16763,#16764,#16765,#16766,#16767,#16768,#16769,#16770,#16771,#16772,
#16773,#16774,#16775,#16776,#16777,#16778,#16779,#16780,#16781,#16782,#16783,
#16784,#16785,#16786,#16787,#16788,#16789,#16790,#16791,#16792,#16793,#16794,
#16795));
#17323=AXIS2_PLACEMENT_3D('',#23993,#19361,#19362);
#17324=AXIS2_PLACEMENT_3D('',#23994,#19363,#19364);
#17325=AXIS2_PLACEMENT_3D('',#24005,#19368,#19369);
#17326=AXIS2_PLACEMENT_3D('',#24007,#19370,#19371);
#17327=AXIS2_PLACEMENT_3D('',#24010,#19373,#19374);
#17328=AXIS2_PLACEMENT_3D('',#24011,#19375,#19376);
#17329=AXIS2_PLACEMENT_3D('',#24018,#19377,#19378);
#17330=AXIS2_PLACEMENT_3D('',#24027,#19379,#19380);
#17331=AXIS2_PLACEMENT_3D('',#24042,#19384,#19385);
#17332=AXIS2_PLACEMENT_3D('',#24044,#19386,#19387);
#17333=AXIS2_PLACEMENT_3D('',#24047,#19389,#19390);
#17334=AXIS2_PLACEMENT_3D('',#24048,#19391,#19392);
#17335=AXIS2_PLACEMENT_3D('',#24055,#19393,#19394);
#17336=AXIS2_PLACEMENT_3D('',#24064,#19395,#19396);
#17337=AXIS2_PLACEMENT_3D('',#24068,#19399,#19400);
#17338=AXIS2_PLACEMENT_3D('',#24070,#19401,#19402);
#17339=AXIS2_PLACEMENT_3D('',#24078,#19404,#19405);
#17340=AXIS2_PLACEMENT_3D('',#24079,#19406,#19407);
#17341=AXIS2_PLACEMENT_3D('',#24094,#19411,#19412);
#17342=AXIS2_PLACEMENT_3D('',#24096,#19413,#19414);
#17343=AXIS2_PLACEMENT_3D('',#24107,#19415,#19416);
#17344=AXIS2_PLACEMENT_3D('',#24112,#19417,#19418);
#17345=AXIS2_PLACEMENT_3D('',#24114,#19419,#19420);
#17346=AXIS2_PLACEMENT_3D('',#24116,#19422,#19423);
#17347=AXIS2_PLACEMENT_3D('',#24131,#19427,#19428);
#17348=AXIS2_PLACEMENT_3D('',#24132,#19429,#19430);
#17349=AXIS2_PLACEMENT_3D('',#24133,#19431,#19432);
#17350=AXIS2_PLACEMENT_3D('',#24134,#19433,#19434);
#17351=AXIS2_PLACEMENT_3D('',#24140,#19435,#19436);
#17352=AXIS2_PLACEMENT_3D('',#24141,#19437,#19438);
#17353=AXIS2_PLACEMENT_3D('',#24156,#19442,#19443);
#17354=AXIS2_PLACEMENT_3D('',#24158,#19444,#19445);
#17355=AXIS2_PLACEMENT_3D('',#24169,#19446,#19447);
#17356=AXIS2_PLACEMENT_3D('',#24174,#19448,#19449);
#17357=AXIS2_PLACEMENT_3D('',#24176,#19450,#19451);
#17358=AXIS2_PLACEMENT_3D('',#24178,#19453,#19454);
#17359=AXIS2_PLACEMENT_3D('',#24186,#19457,#19458);
#17360=AXIS2_PLACEMENT_3D('',#24194,#19461,#19462);
#17361=AXIS2_PLACEMENT_3D('',#24205,#19466,#19467);
#17362=AXIS2_PLACEMENT_3D('',#24212,#19468,#19469);
#17363=AXIS2_PLACEMENT_3D('',#24220,#19471,#19472);
#17364=AXIS2_PLACEMENT_3D('',#24221,#19473,#19474);
#17365=AXIS2_PLACEMENT_3D('',#24223,#19475,#19476);
#17366=AXIS2_PLACEMENT_3D('',#24234,#19477,#19478);
#17367=AXIS2_PLACEMENT_3D('',#24235,#19479,#19480);
#17368=AXIS2_PLACEMENT_3D('',#24250,#19484,#19485);
#17369=AXIS2_PLACEMENT_3D('',#24252,#19486,#19487);
#17370=AXIS2_PLACEMENT_3D('',#24255,#19489,#19490);
#17371=AXIS2_PLACEMENT_3D('',#24256,#19491,#19492);
#17372=AXIS2_PLACEMENT_3D('',#24263,#19493,#19494);
#17373=AXIS2_PLACEMENT_3D('',#24273,#19495,#19496);
#17374=AXIS2_PLACEMENT_3D('',#24288,#19500,#19501);
#17375=AXIS2_PLACEMENT_3D('',#24290,#19502,#19503);
#17376=AXIS2_PLACEMENT_3D('',#24301,#19504,#19505);
#17377=AXIS2_PLACEMENT_3D('',#24306,#19506,#19507);
#17378=AXIS2_PLACEMENT_3D('',#24308,#19508,#19509);
#17379=AXIS2_PLACEMENT_3D('',#24310,#19511,#19512);
#17380=AXIS2_PLACEMENT_3D('',#24318,#19515,#19516);
#17381=AXIS2_PLACEMENT_3D('',#24333,#19520,#19521);
#17382=AXIS2_PLACEMENT_3D('',#24335,#19522,#19523);
#17383=AXIS2_PLACEMENT_3D('',#24346,#19524,#19525);
#17384=AXIS2_PLACEMENT_3D('',#24351,#19526,#19527);
#17385=AXIS2_PLACEMENT_3D('',#24353,#19528,#19529);
#17386=AXIS2_PLACEMENT_3D('',#24355,#19531,#19532);
#17387=AXIS2_PLACEMENT_3D('',#24363,#19535,#19536);
#17388=AXIS2_PLACEMENT_3D('',#24378,#19540,#19541);
#17389=AXIS2_PLACEMENT_3D('',#24380,#19542,#19543);
#17390=AXIS2_PLACEMENT_3D('',#24391,#19544,#19545);
#17391=AXIS2_PLACEMENT_3D('',#24396,#19546,#19547);
#17392=AXIS2_PLACEMENT_3D('',#24398,#19548,#19549);
#17393=AXIS2_PLACEMENT_3D('',#24400,#19551,#19552);
#17394=AXIS2_PLACEMENT_3D('',#24408,#19555,#19556);
#17395=AXIS2_PLACEMENT_3D('',#24423,#19560,#19561);
#17396=AXIS2_PLACEMENT_3D('',#24425,#19562,#19563);
#17397=AXIS2_PLACEMENT_3D('',#24436,#19564,#19565);
#17398=AXIS2_PLACEMENT_3D('',#24441,#19566,#19567);
#17399=AXIS2_PLACEMENT_3D('',#24443,#19568,#19569);
#17400=AXIS2_PLACEMENT_3D('',#24445,#19571,#19572);
#17401=AXIS2_PLACEMENT_3D('',#24453,#19575,#19576);
#17402=AXIS2_PLACEMENT_3D('',#24468,#19580,#19581);
#17403=AXIS2_PLACEMENT_3D('',#24470,#19582,#19583);
#17404=AXIS2_PLACEMENT_3D('',#24481,#19584,#19585);
#17405=AXIS2_PLACEMENT_3D('',#24486,#19586,#19587);
#17406=AXIS2_PLACEMENT_3D('',#24488,#19588,#19589);
#17407=AXIS2_PLACEMENT_3D('',#24490,#19591,#19592);
#17408=AXIS2_PLACEMENT_3D('',#24498,#19595,#19596);
#17409=AXIS2_PLACEMENT_3D('',#24513,#19600,#19601);
#17410=AXIS2_PLACEMENT_3D('',#24515,#19602,#19603);
#17411=AXIS2_PLACEMENT_3D('',#24526,#19604,#19605);
#17412=AXIS2_PLACEMENT_3D('',#24531,#19606,#19607);
#17413=AXIS2_PLACEMENT_3D('',#24533,#19608,#19609);
#17414=AXIS2_PLACEMENT_3D('',#24535,#19611,#19612);
#17415=AXIS2_PLACEMENT_3D('',#24543,#19615,#19616);
#17416=AXIS2_PLACEMENT_3D('',#24558,#19620,#19621);
#17417=AXIS2_PLACEMENT_3D('',#24560,#19622,#19623);
#17418=AXIS2_PLACEMENT_3D('',#24571,#19624,#19625);
#17419=AXIS2_PLACEMENT_3D('',#24576,#19626,#19627);
#17420=AXIS2_PLACEMENT_3D('',#24578,#19628,#19629);
#17421=AXIS2_PLACEMENT_3D('',#24580,#19631,#19632);
#17422=AXIS2_PLACEMENT_3D('',#24588,#19635,#19636);
#17423=AXIS2_PLACEMENT_3D('',#24603,#19640,#19641);
#17424=AXIS2_PLACEMENT_3D('',#24605,#19642,#19643);
#17425=AXIS2_PLACEMENT_3D('',#24616,#19644,#19645);
#17426=AXIS2_PLACEMENT_3D('',#24621,#19646,#19647);
#17427=AXIS2_PLACEMENT_3D('',#24623,#19648,#19649);
#17428=AXIS2_PLACEMENT_3D('',#24625,#19651,#19652);
#17429=AXIS2_PLACEMENT_3D('',#24633,#19655,#19656);
#17430=AXIS2_PLACEMENT_3D('',#24635,#19657,#19658);
#17431=AXIS2_PLACEMENT_3D('',#24647,#19659,#19660);
#17432=AXIS2_PLACEMENT_3D('',#24648,#19661,#19662);
#17433=AXIS2_PLACEMENT_3D('',#24649,#19663,#19664);
#17434=AXIS2_PLACEMENT_3D('',#24650,#19665,#19666);
#17435=AXIS2_PLACEMENT_3D('',#24651,#19667,#19668);
#17436=AXIS2_PLACEMENT_3D('',#24652,#19669,#19670);
#17437=AXIS2_PLACEMENT_3D('',#24653,#19671,#19672);
#17438=AXIS2_PLACEMENT_3D('',#24654,#19673,#19674);
#17439=AXIS2_PLACEMENT_3D('',#24656,#19675,#19676);
#17440=AXIS2_PLACEMENT_3D('',#24666,#19677,#19678);
#17441=AXIS2_PLACEMENT_3D('',#24667,#19679,#19680);
#17442=AXIS2_PLACEMENT_3D('',#24669,#19681,#19682);
#17443=AXIS2_PLACEMENT_3D('',#24671,#19683,#19684);
#17444=AXIS2_PLACEMENT_3D('',#24673,#19685,#19686);
#17445=AXIS2_PLACEMENT_3D('',#24675,#19687,#19688);
#17446=AXIS2_PLACEMENT_3D('',#24677,#19689,#19690);
#17447=AXIS2_PLACEMENT_3D('',#24679,#19691,#19692);
#17448=AXIS2_PLACEMENT_3D('',#24681,#19693,#19694);
#17449=AXIS2_PLACEMENT_3D('',#24683,#19695,#19696);
#17450=AXIS2_PLACEMENT_3D('',#24685,#19697,#19698);
#17451=AXIS2_PLACEMENT_3D('',#24687,#19699,#19700);
#17452=AXIS2_PLACEMENT_3D('',#24689,#19701,#19702);
#17453=AXIS2_PLACEMENT_3D('',#24690,#19703,#19704);
#17454=AXIS2_PLACEMENT_3D('',#24691,#19705,#19706);
#17455=AXIS2_PLACEMENT_3D('',#24692,#19707,#19708);
#17456=AXIS2_PLACEMENT_3D('',#24693,#19709,#19710);
#17457=AXIS2_PLACEMENT_3D('',#24694,#19711,#19712);
#17458=AXIS2_PLACEMENT_3D('',#24695,#19713,#19714);
#17459=AXIS2_PLACEMENT_3D('',#24696,#19715,#19716);
#17460=AXIS2_PLACEMENT_3D('',#24697,#19717,#19718);
#17461=AXIS2_PLACEMENT_3D('',#24698,#19719,#19720);
#17462=AXIS2_PLACEMENT_3D('',#24699,#19721,#19722);
#17463=AXIS2_PLACEMENT_3D('',#24701,#19723,#19724);
#17464=AXIS2_PLACEMENT_3D('',#24703,#19725,#19726);
#17465=AXIS2_PLACEMENT_3D('',#24705,#19727,#19728);
#17466=AXIS2_PLACEMENT_3D('',#24707,#19729,#19730);
#17467=AXIS2_PLACEMENT_3D('',#24709,#19731,#19732);
#17468=AXIS2_PLACEMENT_3D('',#24711,#19733,#19734);
#17469=AXIS2_PLACEMENT_3D('',#24713,#19735,#19736);
#17470=AXIS2_PLACEMENT_3D('',#24715,#19737,#19738);
#17471=AXIS2_PLACEMENT_3D('',#24717,#19739,#19740);
#17472=AXIS2_PLACEMENT_3D('',#24719,#19741,#19742);
#17473=AXIS2_PLACEMENT_3D('',#24721,#19743,#19744);
#17474=AXIS2_PLACEMENT_3D('',#24723,#19745,#19746);
#17475=AXIS2_PLACEMENT_3D('',#24725,#19747,#19748);
#17476=AXIS2_PLACEMENT_3D('',#24727,#19749,#19750);
#17477=AXIS2_PLACEMENT_3D('',#24729,#19751,#19752);
#17478=AXIS2_PLACEMENT_3D('',#24731,#19753,#19754);
#17479=AXIS2_PLACEMENT_3D('',#24733,#19755,#19756);
#17480=AXIS2_PLACEMENT_3D('',#24734,#19757,#19758);
#17481=AXIS2_PLACEMENT_3D('',#24736,#19759,#19760);
#17482=AXIS2_PLACEMENT_3D('',#24738,#19761,#19762);
#17483=AXIS2_PLACEMENT_3D('',#24740,#19763,#19764);
#17484=AXIS2_PLACEMENT_3D('',#24742,#19765,#19766);
#17485=AXIS2_PLACEMENT_3D('',#24744,#19767,#19768);
#17486=AXIS2_PLACEMENT_3D('',#24746,#19769,#19770);
#17487=AXIS2_PLACEMENT_3D('',#24748,#19771,#19772);
#17488=AXIS2_PLACEMENT_3D('',#24750,#19773,#19774);
#17489=AXIS2_PLACEMENT_3D('',#24752,#19775,#19776);
#17490=AXIS2_PLACEMENT_3D('',#24754,#19777,#19778);
#17491=AXIS2_PLACEMENT_3D('',#24756,#19779,#19780);
#17492=AXIS2_PLACEMENT_3D('',#24758,#19781,#19782);
#17493=AXIS2_PLACEMENT_3D('',#24760,#19783,#19784);
#17494=AXIS2_PLACEMENT_3D('',#24762,#19785,#19786);
#17495=AXIS2_PLACEMENT_3D('',#24764,#19787,#19788);
#17496=AXIS2_PLACEMENT_3D('',#24766,#19789,#19790);
#17497=AXIS2_PLACEMENT_3D('',#24768,#19791,#19792);
#17498=AXIS2_PLACEMENT_3D('',#24770,#19793,#19794);
#17499=AXIS2_PLACEMENT_3D('',#24772,#19795,#19796);
#17500=AXIS2_PLACEMENT_3D('',#24774,#19797,#19798);
#17501=AXIS2_PLACEMENT_3D('',#24776,#19799,#19800);
#17502=AXIS2_PLACEMENT_3D('',#24778,#19801,#19802);
#17503=AXIS2_PLACEMENT_3D('',#24780,#19803,#19804);
#17504=AXIS2_PLACEMENT_3D('',#24782,#19805,#19806);
#17505=AXIS2_PLACEMENT_3D('',#24784,#19807,#19808);
#17506=AXIS2_PLACEMENT_3D('',#24786,#19809,#19810);
#17507=AXIS2_PLACEMENT_3D('',#24788,#19811,#19812);
#17508=AXIS2_PLACEMENT_3D('',#24790,#19813,#19814);
#17509=AXIS2_PLACEMENT_3D('',#24792,#19815,#19816);
#17510=AXIS2_PLACEMENT_3D('',#24794,#19817,#19818);
#17511=AXIS2_PLACEMENT_3D('',#24796,#19819,#19820);
#17512=AXIS2_PLACEMENT_3D('',#24798,#19821,#19822);
#17513=AXIS2_PLACEMENT_3D('',#24800,#19823,#19824);
#17514=AXIS2_PLACEMENT_3D('',#24802,#19825,#19826);
#17515=AXIS2_PLACEMENT_3D('',#24804,#19827,#19828);
#17516=AXIS2_PLACEMENT_3D('',#24806,#19829,#19830);
#17517=AXIS2_PLACEMENT_3D('',#24808,#19831,#19832);
#17518=AXIS2_PLACEMENT_3D('',#24810,#19833,#19834);
#17519=AXIS2_PLACEMENT_3D('',#24812,#19835,#19836);
#17520=AXIS2_PLACEMENT_3D('',#24814,#19837,#19838);
#17521=AXIS2_PLACEMENT_3D('',#24816,#19839,#19840);
#17522=AXIS2_PLACEMENT_3D('',#24818,#19841,#19842);
#17523=AXIS2_PLACEMENT_3D('',#24820,#19843,#19844);
#17524=AXIS2_PLACEMENT_3D('',#24822,#19845,#19846);
#17525=AXIS2_PLACEMENT_3D('',#24824,#19847,#19848);
#17526=AXIS2_PLACEMENT_3D('',#24826,#19849,#19850);
#17527=AXIS2_PLACEMENT_3D('',#24828,#19851,#19852);
#17528=AXIS2_PLACEMENT_3D('',#24830,#19853,#19854);
#17529=AXIS2_PLACEMENT_3D('',#24832,#19855,#19856);
#17530=AXIS2_PLACEMENT_3D('',#24834,#19857,#19858);
#17531=AXIS2_PLACEMENT_3D('',#24836,#19859,#19860);
#17532=AXIS2_PLACEMENT_3D('',#24838,#19861,#19862);
#17533=AXIS2_PLACEMENT_3D('',#24840,#19863,#19864);
#17534=AXIS2_PLACEMENT_3D('',#24842,#19865,#19866);
#17535=AXIS2_PLACEMENT_3D('',#24844,#19867,#19868);
#17536=AXIS2_PLACEMENT_3D('',#24846,#19869,#19870);
#17537=AXIS2_PLACEMENT_3D('',#24848,#19871,#19872);
#17538=AXIS2_PLACEMENT_3D('',#24850,#19873,#19874);
#17539=AXIS2_PLACEMENT_3D('',#24852,#19875,#19876);
#17540=AXIS2_PLACEMENT_3D('',#24854,#19877,#19878);
#17541=AXIS2_PLACEMENT_3D('',#24856,#19879,#19880);
#17542=AXIS2_PLACEMENT_3D('',#24858,#19881,#19882);
#17543=AXIS2_PLACEMENT_3D('',#24860,#19883,#19884);
#17544=AXIS2_PLACEMENT_3D('',#24862,#19885,#19886);
#17545=AXIS2_PLACEMENT_3D('',#24864,#19887,#19888);
#17546=AXIS2_PLACEMENT_3D('',#24866,#19889,#19890);
#17547=AXIS2_PLACEMENT_3D('',#24868,#19891,#19892);
#17548=AXIS2_PLACEMENT_3D('',#24870,#19893,#19894);
#17549=AXIS2_PLACEMENT_3D('',#24872,#19895,#19896);
#17550=AXIS2_PLACEMENT_3D('',#24874,#19897,#19898);
#17551=AXIS2_PLACEMENT_3D('',#24876,#19899,#19900);
#17552=AXIS2_PLACEMENT_3D('',#24878,#19901,#19902);
#17553=AXIS2_PLACEMENT_3D('',#24880,#19903,#19904);
#17554=AXIS2_PLACEMENT_3D('',#24882,#19905,#19906);
#17555=AXIS2_PLACEMENT_3D('',#24884,#19907,#19908);
#17556=AXIS2_PLACEMENT_3D('',#24886,#19909,#19910);
#17557=AXIS2_PLACEMENT_3D('',#24888,#19911,#19912);
#17558=AXIS2_PLACEMENT_3D('',#24890,#19913,#19914);
#17559=AXIS2_PLACEMENT_3D('',#24892,#19915,#19916);
#17560=AXIS2_PLACEMENT_3D('',#24894,#19917,#19918);
#17561=AXIS2_PLACEMENT_3D('',#24896,#19919,#19920);
#17562=AXIS2_PLACEMENT_3D('',#24898,#19921,#19922);
#17563=AXIS2_PLACEMENT_3D('',#24900,#19923,#19924);
#17564=AXIS2_PLACEMENT_3D('',#24902,#19925,#19926);
#17565=AXIS2_PLACEMENT_3D('',#24904,#19927,#19928);
#17566=AXIS2_PLACEMENT_3D('',#24906,#19929,#19930);
#17567=AXIS2_PLACEMENT_3D('',#24908,#19931,#19932);
#17568=AXIS2_PLACEMENT_3D('',#24910,#19933,#19934);
#17569=AXIS2_PLACEMENT_3D('',#24912,#19935,#19936);
#17570=AXIS2_PLACEMENT_3D('',#24914,#19937,#19938);
#17571=AXIS2_PLACEMENT_3D('',#24916,#19939,#19940);
#17572=AXIS2_PLACEMENT_3D('',#24918,#19941,#19942);
#17573=AXIS2_PLACEMENT_3D('',#24920,#19943,#19944);
#17574=AXIS2_PLACEMENT_3D('',#24922,#19945,#19946);
#17575=AXIS2_PLACEMENT_3D('',#24924,#19947,#19948);
#17576=AXIS2_PLACEMENT_3D('',#24926,#19949,#19950);
#17577=AXIS2_PLACEMENT_3D('',#24928,#19951,#19952);
#17578=AXIS2_PLACEMENT_3D('',#24930,#19953,#19954);
#17579=AXIS2_PLACEMENT_3D('',#24932,#19955,#19956);
#17580=AXIS2_PLACEMENT_3D('',#24934,#19957,#19958);
#17581=AXIS2_PLACEMENT_3D('',#24936,#19959,#19960);
#17582=AXIS2_PLACEMENT_3D('',#24938,#19961,#19962);
#17583=AXIS2_PLACEMENT_3D('',#24940,#19963,#19964);
#17584=AXIS2_PLACEMENT_3D('',#24942,#19965,#19966);
#17585=AXIS2_PLACEMENT_3D('',#24944,#19967,#19968);
#17586=AXIS2_PLACEMENT_3D('',#24946,#19969,#19970);
#17587=AXIS2_PLACEMENT_3D('',#24948,#19971,#19972);
#17588=AXIS2_PLACEMENT_3D('',#24950,#19973,#19974);
#17589=AXIS2_PLACEMENT_3D('',#24952,#19975,#19976);
#17590=AXIS2_PLACEMENT_3D('',#24954,#19977,#19978);
#17591=AXIS2_PLACEMENT_3D('',#24956,#19979,#19980);
#17592=AXIS2_PLACEMENT_3D('',#24958,#19981,#19982);
#17593=AXIS2_PLACEMENT_3D('',#24960,#19983,#19984);
#17594=AXIS2_PLACEMENT_3D('',#24962,#19985,#19986);
#17595=AXIS2_PLACEMENT_3D('',#24964,#19987,#19988);
#17596=AXIS2_PLACEMENT_3D('',#24966,#19989,#19990);
#17597=AXIS2_PLACEMENT_3D('',#24968,#19991,#19992);
#17598=AXIS2_PLACEMENT_3D('',#24970,#19993,#19994);
#17599=AXIS2_PLACEMENT_3D('',#24972,#19995,#19996);
#17600=AXIS2_PLACEMENT_3D('',#24973,#19997,#19998);
#17601=AXIS2_PLACEMENT_3D('',#24975,#19999,#20000);
#17602=AXIS2_PLACEMENT_3D('',#24976,#20001,#20002);
#17603=AXIS2_PLACEMENT_3D('',#24980,#20004,#20005);
#17604=AXIS2_PLACEMENT_3D('',#24987,#20007,#20008);
#17605=AXIS2_PLACEMENT_3D('',#24991,#20011,#20012);
#17606=AXIS2_PLACEMENT_3D('',#25006,#20016,#20017);
#17607=AXIS2_PLACEMENT_3D('',#25008,#20018,#20019);
#17608=AXIS2_PLACEMENT_3D('',#25021,#20020,#20021);
#17609=AXIS2_PLACEMENT_3D('',#25023,#20022,#20023);
#17610=AXIS2_PLACEMENT_3D('',#25025,#20025,#20026);
#17611=AXIS2_PLACEMENT_3D('',#25033,#20029,#20030);
#17612=AXIS2_PLACEMENT_3D('',#25048,#20034,#20035);
#17613=AXIS2_PLACEMENT_3D('',#25050,#20036,#20037);
#17614=AXIS2_PLACEMENT_3D('',#25063,#20038,#20039);
#17615=AXIS2_PLACEMENT_3D('',#25065,#20040,#20041);
#17616=AXIS2_PLACEMENT_3D('',#25067,#20043,#20044);
#17617=AXIS2_PLACEMENT_3D('',#25075,#20047,#20048);
#17618=AXIS2_PLACEMENT_3D('',#25090,#20052,#20053);
#17619=AXIS2_PLACEMENT_3D('',#25092,#20054,#20055);
#17620=AXIS2_PLACEMENT_3D('',#25105,#20056,#20057);
#17621=AXIS2_PLACEMENT_3D('',#25107,#20058,#20059);
#17622=AXIS2_PLACEMENT_3D('',#25109,#20061,#20062);
#17623=AXIS2_PLACEMENT_3D('',#25117,#20065,#20066);
#17624=AXIS2_PLACEMENT_3D('',#25119,#20067,#20068);
#17625=AXIS2_PLACEMENT_3D('',#25122,#20070,#20071);
#17626=AXIS2_PLACEMENT_3D('',#25123,#20072,#20073);
#17627=AXIS2_PLACEMENT_3D('',#25127,#20074,#20075);
#17628=AXIS2_PLACEMENT_3D('',#25129,#20077,#20078);
#17629=AXIS2_PLACEMENT_3D('',#25140,#20082,#20083);
#17630=AXIS2_PLACEMENT_3D('',#25142,#20084,#20085);
#17631=AXIS2_PLACEMENT_3D('',#25155,#20086,#20087);
#17632=AXIS2_PLACEMENT_3D('',#25157,#20088,#20089);
#17633=AXIS2_PLACEMENT_3D('',#25159,#20091,#20092);
#17634=AXIS2_PLACEMENT_3D('',#25167,#20095,#20096);
#17635=AXIS2_PLACEMENT_3D('',#25182,#20100,#20101);
#17636=AXIS2_PLACEMENT_3D('',#25184,#20102,#20103);
#17637=AXIS2_PLACEMENT_3D('',#25197,#20104,#20105);
#17638=AXIS2_PLACEMENT_3D('',#25199,#20106,#20107);
#17639=AXIS2_PLACEMENT_3D('',#25201,#20109,#20110);
#17640=AXIS2_PLACEMENT_3D('',#25209,#20113,#20114);
#17641=AXIS2_PLACEMENT_3D('',#25224,#20118,#20119);
#17642=AXIS2_PLACEMENT_3D('',#25226,#20120,#20121);
#17643=AXIS2_PLACEMENT_3D('',#25239,#20122,#20123);
#17644=AXIS2_PLACEMENT_3D('',#25241,#20124,#20125);
#17645=AXIS2_PLACEMENT_3D('',#25243,#20127,#20128);
#17646=AXIS2_PLACEMENT_3D('',#25251,#20131,#20132);
#17647=AXIS2_PLACEMENT_3D('',#25266,#20136,#20137);
#17648=AXIS2_PLACEMENT_3D('',#25268,#20138,#20139);
#17649=AXIS2_PLACEMENT_3D('',#25281,#20140,#20141);
#17650=AXIS2_PLACEMENT_3D('',#25283,#20142,#20143);
#17651=AXIS2_PLACEMENT_3D('',#25285,#20145,#20146);
#17652=AXIS2_PLACEMENT_3D('',#25293,#20149,#20150);
#17653=AXIS2_PLACEMENT_3D('',#25308,#20154,#20155);
#17654=AXIS2_PLACEMENT_3D('',#25310,#20156,#20157);
#17655=AXIS2_PLACEMENT_3D('',#25323,#20158,#20159);
#17656=AXIS2_PLACEMENT_3D('',#25325,#20160,#20161);
#17657=AXIS2_PLACEMENT_3D('',#25327,#20163,#20164);
#17658=AXIS2_PLACEMENT_3D('',#25335,#20167,#20168);
#17659=AXIS2_PLACEMENT_3D('',#25350,#20172,#20173);
#17660=AXIS2_PLACEMENT_3D('',#25352,#20174,#20175);
#17661=AXIS2_PLACEMENT_3D('',#25365,#20176,#20177);
#17662=AXIS2_PLACEMENT_3D('',#25367,#20178,#20179);
#17663=AXIS2_PLACEMENT_3D('',#25369,#20181,#20182);
#17664=AXIS2_PLACEMENT_3D('',#25381,#20186,#20187);
#17665=AXIS2_PLACEMENT_3D('',#25386,#20188,#20189);
#17666=AXIS2_PLACEMENT_3D('',#25387,#20190,#20191);
#17667=AXIS2_PLACEMENT_3D('',#25388,#20192,#20193);
#17668=AXIS2_PLACEMENT_3D('',#25389,#20194,#20195);
#17669=AXIS2_PLACEMENT_3D('',#25390,#20196,#20197);
#17670=AXIS2_PLACEMENT_3D('',#25391,#20198,#20199);
#17671=AXIS2_PLACEMENT_3D('',#25392,#20200,#20201);
#17672=AXIS2_PLACEMENT_3D('',#25393,#20202,#20203);
#17673=AXIS2_PLACEMENT_3D('',#25394,#20204,#20205);
#17674=AXIS2_PLACEMENT_3D('',#25395,#20206,#20207);
#17675=AXIS2_PLACEMENT_3D('',#25396,#20208,#20209);
#17676=AXIS2_PLACEMENT_3D('',#25397,#20210,#20211);
#17677=AXIS2_PLACEMENT_3D('',#25401,#20214,#20215);
#17678=AXIS2_PLACEMENT_3D('',#25402,#20216,#20217);
#17679=AXIS2_PLACEMENT_3D('',#25403,#20218,#20219);
#17680=AXIS2_PLACEMENT_3D('',#25404,#20220,#20221);
#17681=AXIS2_PLACEMENT_3D('',#25405,#20222,#20223);
#17682=AXIS2_PLACEMENT_3D('',#25406,#20224,#20225);
#17683=AXIS2_PLACEMENT_3D('',#25407,#20226,#20227);
#17684=AXIS2_PLACEMENT_3D('',#25408,#20228,#20229);
#17685=AXIS2_PLACEMENT_3D('',#25409,#20230,#20231);
#17686=AXIS2_PLACEMENT_3D('',#25410,#20232,#20233);
#17687=AXIS2_PLACEMENT_3D('',#25411,#20234,#20235);
#17688=AXIS2_PLACEMENT_3D('',#25412,#20236,#20237);
#17689=AXIS2_PLACEMENT_3D('',#25413,#20238,#20239);
#17690=AXIS2_PLACEMENT_3D('',#25414,#20240,#20241);
#17691=AXIS2_PLACEMENT_3D('',#25415,#20242,#20243);
#17692=AXIS2_PLACEMENT_3D('',#25416,#20244,#20245);
#17693=AXIS2_PLACEMENT_3D('',#25417,#20246,#20247);
#17694=AXIS2_PLACEMENT_3D('',#25418,#20248,#20249);
#17695=AXIS2_PLACEMENT_3D('',#25419,#20250,#20251);
#17696=AXIS2_PLACEMENT_3D('',#25420,#20252,#20253);
#17697=AXIS2_PLACEMENT_3D('',#25421,#20254,#20255);
#17698=AXIS2_PLACEMENT_3D('',#25422,#20256,#20257);
#17699=AXIS2_PLACEMENT_3D('',#25423,#20258,#20259);
#17700=AXIS2_PLACEMENT_3D('',#25438,#20263,#20264);
#17701=AXIS2_PLACEMENT_3D('',#25440,#20265,#20266);
#17702=AXIS2_PLACEMENT_3D('',#25453,#20267,#20268);
#17703=AXIS2_PLACEMENT_3D('',#25455,#20269,#20270);
#17704=AXIS2_PLACEMENT_3D('',#25457,#20272,#20273);
#17705=AXIS2_PLACEMENT_3D('',#25465,#20276,#20277);
#17706=AXIS2_PLACEMENT_3D('',#25467,#20278,#20279);
#17707=AXIS2_PLACEMENT_3D('',#25476,#20280,#20281);
#17708=AXIS2_PLACEMENT_3D('',#25486,#20285,#20286);
#17709=AXIS2_PLACEMENT_3D('',#25488,#20287,#20288);
#17710=AXIS2_PLACEMENT_3D('',#25497,#20289,#20290);
#17711=AXIS2_PLACEMENT_3D('',#25499,#20291,#20292);
#17712=AXIS2_PLACEMENT_3D('',#25501,#20294,#20295);
#17713=AXIS2_PLACEMENT_3D('',#25509,#20298,#20299);
#17714=AXIS2_PLACEMENT_3D('',#25524,#20303,#20304);
#17715=AXIS2_PLACEMENT_3D('',#25526,#20305,#20306);
#17716=AXIS2_PLACEMENT_3D('',#25539,#20307,#20308);
#17717=AXIS2_PLACEMENT_3D('',#25541,#20309,#20310);
#17718=AXIS2_PLACEMENT_3D('',#25543,#20312,#20313);
#17719=AXIS2_PLACEMENT_3D('',#25551,#20316,#20317);
#17720=AXIS2_PLACEMENT_3D('',#25566,#20321,#20322);
#17721=AXIS2_PLACEMENT_3D('',#25568,#20323,#20324);
#17722=AXIS2_PLACEMENT_3D('',#25581,#20325,#20326);
#17723=AXIS2_PLACEMENT_3D('',#25583,#20327,#20328);
#17724=AXIS2_PLACEMENT_3D('',#25585,#20330,#20331);
#17725=AXIS2_PLACEMENT_3D('',#25596,#20335,#20336);
#17726=AXIS2_PLACEMENT_3D('',#25598,#20337,#20338);
#17727=AXIS2_PLACEMENT_3D('',#25601,#20340,#20341);
#17728=AXIS2_PLACEMENT_3D('',#25602,#20342,#20343);
#17729=AXIS2_PLACEMENT_3D('',#25610,#20344,#20345);
#17730=AXIS2_PLACEMENT_3D('',#25612,#20347,#20348);
#17731=AXIS2_PLACEMENT_3D('',#25623,#20352,#20353);
#17732=AXIS2_PLACEMENT_3D('',#25625,#20354,#20355);
#17733=AXIS2_PLACEMENT_3D('',#25638,#20356,#20357);
#17734=AXIS2_PLACEMENT_3D('',#25640,#20358,#20359);
#17735=AXIS2_PLACEMENT_3D('',#25642,#20361,#20362);
#17736=AXIS2_PLACEMENT_3D('',#25650,#20365,#20366);
#17737=AXIS2_PLACEMENT_3D('',#25665,#20370,#20371);
#17738=AXIS2_PLACEMENT_3D('',#25667,#20372,#20373);
#17739=AXIS2_PLACEMENT_3D('',#25680,#20374,#20375);
#17740=AXIS2_PLACEMENT_3D('',#25682,#20376,#20377);
#17741=AXIS2_PLACEMENT_3D('',#25684,#20379,#20380);
#17742=AXIS2_PLACEMENT_3D('',#25692,#20383,#20384);
#17743=AXIS2_PLACEMENT_3D('',#25707,#20388,#20389);
#17744=AXIS2_PLACEMENT_3D('',#25709,#20390,#20391);
#17745=AXIS2_PLACEMENT_3D('',#25722,#20392,#20393);
#17746=AXIS2_PLACEMENT_3D('',#25724,#20394,#20395);
#17747=AXIS2_PLACEMENT_3D('',#25726,#20397,#20398);
#17748=AXIS2_PLACEMENT_3D('',#25734,#20401,#20402);
#17749=AXIS2_PLACEMENT_3D('',#25749,#20406,#20407);
#17750=AXIS2_PLACEMENT_3D('',#25751,#20408,#20409);
#17751=AXIS2_PLACEMENT_3D('',#25764,#20410,#20411);
#17752=AXIS2_PLACEMENT_3D('',#25766,#20412,#20413);
#17753=AXIS2_PLACEMENT_3D('',#25768,#20415,#20416);
#17754=AXIS2_PLACEMENT_3D('',#25776,#20419,#20420);
#17755=AXIS2_PLACEMENT_3D('',#25791,#20424,#20425);
#17756=AXIS2_PLACEMENT_3D('',#25793,#20426,#20427);
#17757=AXIS2_PLACEMENT_3D('',#25806,#20428,#20429);
#17758=AXIS2_PLACEMENT_3D('',#25808,#20430,#20431);
#17759=AXIS2_PLACEMENT_3D('',#25810,#20433,#20434);
#17760=AXIS2_PLACEMENT_3D('',#25822,#20438,#20439);
#17761=AXIS2_PLACEMENT_3D('',#25827,#20440,#20441);
#17762=AXIS2_PLACEMENT_3D('',#25828,#20442,#20443);
#17763=AXIS2_PLACEMENT_3D('',#25829,#20444,#20445);
#17764=AXIS2_PLACEMENT_3D('',#25830,#20446,#20447);
#17765=AXIS2_PLACEMENT_3D('',#25831,#20448,#20449);
#17766=AXIS2_PLACEMENT_3D('',#25832,#20450,#20451);
#17767=AXIS2_PLACEMENT_3D('',#25833,#20452,#20453);
#17768=AXIS2_PLACEMENT_3D('',#25834,#20454,#20455);
#17769=AXIS2_PLACEMENT_3D('',#25835,#20456,#20457);
#17770=AXIS2_PLACEMENT_3D('',#25836,#20458,#20459);
#17771=AXIS2_PLACEMENT_3D('',#25837,#20460,#20461);
#17772=AXIS2_PLACEMENT_3D('',#25838,#20462,#20463);
#17773=AXIS2_PLACEMENT_3D('',#25839,#20464,#20465);
#17774=AXIS2_PLACEMENT_3D('',#25840,#20466,#20467);
#17775=AXIS2_PLACEMENT_3D('',#25844,#20470,#20471);
#17776=AXIS2_PLACEMENT_3D('',#25845,#20472,#20473);
#17777=AXIS2_PLACEMENT_3D('',#25846,#20474,#20475);
#17778=AXIS2_PLACEMENT_3D('',#25847,#20476,#20477);
#17779=AXIS2_PLACEMENT_3D('',#25848,#20478,#20479);
#17780=AXIS2_PLACEMENT_3D('',#25849,#20480,#20481);
#17781=AXIS2_PLACEMENT_3D('',#25850,#20482,#20483);
#17782=AXIS2_PLACEMENT_3D('',#25851,#20484,#20485);
#17783=AXIS2_PLACEMENT_3D('',#25852,#20486,#20487);
#17784=AXIS2_PLACEMENT_3D('',#25853,#20488,#20489);
#17785=AXIS2_PLACEMENT_3D('',#25854,#20490,#20491);
#17786=AXIS2_PLACEMENT_3D('',#25855,#20492,#20493);
#17787=AXIS2_PLACEMENT_3D('',#25856,#20494,#20495);
#17788=AXIS2_PLACEMENT_3D('',#25857,#20496,#20497);
#17789=AXIS2_PLACEMENT_3D('',#25858,#20498,#20499);
#17790=AXIS2_PLACEMENT_3D('',#25859,#20500,#20501);
#17791=AXIS2_PLACEMENT_3D('',#25860,#20502,#20503);
#17792=AXIS2_PLACEMENT_3D('',#25861,#20504,#20505);
#17793=AXIS2_PLACEMENT_3D('',#25862,#20506,#20507);
#17794=AXIS2_PLACEMENT_3D('',#25877,#20511,#20512);
#17795=AXIS2_PLACEMENT_3D('',#25879,#20513,#20514);
#17796=AXIS2_PLACEMENT_3D('',#25892,#20515,#20516);
#17797=AXIS2_PLACEMENT_3D('',#25894,#20517,#20518);
#17798=AXIS2_PLACEMENT_3D('',#25896,#20520,#20521);
#17799=AXIS2_PLACEMENT_3D('',#25904,#20524,#20525);
#17800=AXIS2_PLACEMENT_3D('',#25919,#20529,#20530);
#17801=AXIS2_PLACEMENT_3D('',#25921,#20531,#20532);
#17802=AXIS2_PLACEMENT_3D('',#25934,#20533,#20534);
#17803=AXIS2_PLACEMENT_3D('',#25936,#20535,#20536);
#17804=AXIS2_PLACEMENT_3D('',#25938,#20538,#20539);
#17805=AXIS2_PLACEMENT_3D('',#25946,#20542,#20543);
#17806=AXIS2_PLACEMENT_3D('',#25961,#20547,#20548);
#17807=AXIS2_PLACEMENT_3D('',#25963,#20549,#20550);
#17808=AXIS2_PLACEMENT_3D('',#25976,#20551,#20552);
#17809=AXIS2_PLACEMENT_3D('',#25978,#20553,#20554);
#17810=AXIS2_PLACEMENT_3D('',#25980,#20556,#20557);
#17811=AXIS2_PLACEMENT_3D('',#25988,#20560,#20561);
#17812=AXIS2_PLACEMENT_3D('',#26003,#20565,#20566);
#17813=AXIS2_PLACEMENT_3D('',#26005,#20567,#20568);
#17814=AXIS2_PLACEMENT_3D('',#26018,#20569,#20570);
#17815=AXIS2_PLACEMENT_3D('',#26020,#20571,#20572);
#17816=AXIS2_PLACEMENT_3D('',#26022,#20574,#20575);
#17817=AXIS2_PLACEMENT_3D('',#26030,#20578,#20579);
#17818=AXIS2_PLACEMENT_3D('',#26045,#20583,#20584);
#17819=AXIS2_PLACEMENT_3D('',#26047,#20585,#20586);
#17820=AXIS2_PLACEMENT_3D('',#26060,#20587,#20588);
#17821=AXIS2_PLACEMENT_3D('',#26062,#20589,#20590);
#17822=AXIS2_PLACEMENT_3D('',#26064,#20592,#20593);
#17823=AXIS2_PLACEMENT_3D('',#26075,#20597,#20598);
#17824=AXIS2_PLACEMENT_3D('',#26077,#20599,#20600);
#17825=AXIS2_PLACEMENT_3D('',#26080,#20602,#20603);
#17826=AXIS2_PLACEMENT_3D('',#26081,#20604,#20605);
#17827=AXIS2_PLACEMENT_3D('',#26089,#20606,#20607);
#17828=AXIS2_PLACEMENT_3D('',#26091,#20609,#20610);
#17829=AXIS2_PLACEMENT_3D('',#26102,#20614,#20615);
#17830=AXIS2_PLACEMENT_3D('',#26104,#20616,#20617);
#17831=AXIS2_PLACEMENT_3D('',#26117,#20618,#20619);
#17832=AXIS2_PLACEMENT_3D('',#26119,#20620,#20621);
#17833=AXIS2_PLACEMENT_3D('',#26121,#20623,#20624);
#17834=AXIS2_PLACEMENT_3D('',#26129,#20627,#20628);
#17835=AXIS2_PLACEMENT_3D('',#26144,#20632,#20633);
#17836=AXIS2_PLACEMENT_3D('',#26146,#20634,#20635);
#17837=AXIS2_PLACEMENT_3D('',#26159,#20636,#20637);
#17838=AXIS2_PLACEMENT_3D('',#26161,#20638,#20639);
#17839=AXIS2_PLACEMENT_3D('',#26163,#20641,#20642);
#17840=AXIS2_PLACEMENT_3D('',#26171,#20645,#20646);
#17841=AXIS2_PLACEMENT_3D('',#26186,#20650,#20651);
#17842=AXIS2_PLACEMENT_3D('',#26188,#20652,#20653);
#17843=AXIS2_PLACEMENT_3D('',#26201,#20654,#20655);
#17844=AXIS2_PLACEMENT_3D('',#26203,#20656,#20657);
#17845=AXIS2_PLACEMENT_3D('',#26205,#20659,#20660);
#17846=AXIS2_PLACEMENT_3D('',#26213,#20663,#20664);
#17847=AXIS2_PLACEMENT_3D('',#26228,#20668,#20669);
#17848=AXIS2_PLACEMENT_3D('',#26230,#20670,#20671);
#17849=AXIS2_PLACEMENT_3D('',#26243,#20672,#20673);
#17850=AXIS2_PLACEMENT_3D('',#26245,#20674,#20675);
#17851=AXIS2_PLACEMENT_3D('',#26247,#20677,#20678);
#17852=AXIS2_PLACEMENT_3D('',#26259,#20682,#20683);
#17853=AXIS2_PLACEMENT_3D('',#26264,#20684,#20685);
#17854=AXIS2_PLACEMENT_3D('',#26265,#20686,#20687);
#17855=AXIS2_PLACEMENT_3D('',#26266,#20688,#20689);
#17856=AXIS2_PLACEMENT_3D('',#26267,#20690,#20691);
#17857=AXIS2_PLACEMENT_3D('',#26268,#20692,#20693);
#17858=AXIS2_PLACEMENT_3D('',#26269,#20694,#20695);
#17859=AXIS2_PLACEMENT_3D('',#26270,#20696,#20697);
#17860=AXIS2_PLACEMENT_3D('',#26271,#20698,#20699);
#17861=AXIS2_PLACEMENT_3D('',#26272,#20700,#20701);
#17862=AXIS2_PLACEMENT_3D('',#26273,#20702,#20703);
#17863=AXIS2_PLACEMENT_3D('',#26274,#20704,#20705);
#17864=AXIS2_PLACEMENT_3D('',#26275,#20706,#20707);
#17865=AXIS2_PLACEMENT_3D('',#26276,#20708,#20709);
#17866=AXIS2_PLACEMENT_3D('',#26277,#20710,#20711);
#17867=AXIS2_PLACEMENT_3D('',#26278,#20712,#20713);
#17868=AXIS2_PLACEMENT_3D('',#26279,#20714,#20715);
#17869=AXIS2_PLACEMENT_3D('',#26280,#20716,#20717);
#17870=AXIS2_PLACEMENT_3D('',#26281,#20718,#20719);
#17871=AXIS2_PLACEMENT_3D('',#26282,#20720,#20721);
#17872=AXIS2_PLACEMENT_3D('',#26283,#20722,#20723);
#17873=AXIS2_PLACEMENT_3D('',#26287,#20726,#20727);
#17874=AXIS2_PLACEMENT_3D('',#26288,#20728,#20729);
#17875=AXIS2_PLACEMENT_3D('',#26289,#20730,#20731);
#17876=AXIS2_PLACEMENT_3D('',#26290,#20732,#20733);
#17877=AXIS2_PLACEMENT_3D('',#26291,#20734,#20735);
#17878=AXIS2_PLACEMENT_3D('',#26292,#20736,#20737);
#17879=AXIS2_PLACEMENT_3D('',#26293,#20738,#20739);
#17880=AXIS2_PLACEMENT_3D('',#26294,#20740,#20741);
#17881=AXIS2_PLACEMENT_3D('',#26295,#20742,#20743);
#17882=AXIS2_PLACEMENT_3D('',#26296,#20744,#20745);
#17883=AXIS2_PLACEMENT_3D('',#26297,#20746,#20747);
#17884=AXIS2_PLACEMENT_3D('',#26298,#20748,#20749);
#17885=AXIS2_PLACEMENT_3D('',#26299,#20750,#20751);
#17886=AXIS2_PLACEMENT_3D('',#26300,#20752,#20753);
#17887=AXIS2_PLACEMENT_3D('',#26301,#20754,#20755);
#17888=AXIS2_PLACEMENT_3D('',#26316,#20759,#20760);
#17889=AXIS2_PLACEMENT_3D('',#26318,#20761,#20762);
#17890=AXIS2_PLACEMENT_3D('',#26331,#20763,#20764);
#17891=AXIS2_PLACEMENT_3D('',#26333,#20765,#20766);
#17892=AXIS2_PLACEMENT_3D('',#26335,#20768,#20769);
#17893=AXIS2_PLACEMENT_3D('',#26343,#20772,#20773);
#17894=AXIS2_PLACEMENT_3D('',#26345,#20774,#20775);
#17895=AXIS2_PLACEMENT_3D('',#26354,#20776,#20777);
#17896=AXIS2_PLACEMENT_3D('',#26364,#20781,#20782);
#17897=AXIS2_PLACEMENT_3D('',#26366,#20783,#20784);
#17898=AXIS2_PLACEMENT_3D('',#26375,#20785,#20786);
#17899=AXIS2_PLACEMENT_3D('',#26377,#20787,#20788);
#17900=AXIS2_PLACEMENT_3D('',#26379,#20790,#20791);
#17901=AXIS2_PLACEMENT_3D('',#26387,#20794,#20795);
#17902=AXIS2_PLACEMENT_3D('',#26402,#20799,#20800);
#17903=AXIS2_PLACEMENT_3D('',#26404,#20801,#20802);
#17904=AXIS2_PLACEMENT_3D('',#26417,#20803,#20804);
#17905=AXIS2_PLACEMENT_3D('',#26419,#20805,#20806);
#17906=AXIS2_PLACEMENT_3D('',#26421,#20808,#20809);
#17907=AXIS2_PLACEMENT_3D('',#26429,#20812,#20813);
#17908=AXIS2_PLACEMENT_3D('',#26444,#20817,#20818);
#17909=AXIS2_PLACEMENT_3D('',#26446,#20819,#20820);
#17910=AXIS2_PLACEMENT_3D('',#26459,#20821,#20822);
#17911=AXIS2_PLACEMENT_3D('',#26461,#20823,#20824);
#17912=AXIS2_PLACEMENT_3D('',#26463,#20826,#20827);
#17913=AXIS2_PLACEMENT_3D('',#26471,#20830,#20831);
#17914=AXIS2_PLACEMENT_3D('',#26486,#20835,#20836);
#17915=AXIS2_PLACEMENT_3D('',#26488,#20837,#20838);
#17916=AXIS2_PLACEMENT_3D('',#26501,#20839,#20840);
#17917=AXIS2_PLACEMENT_3D('',#26503,#20841,#20842);
#17918=AXIS2_PLACEMENT_3D('',#26505,#20844,#20845);
#17919=AXIS2_PLACEMENT_3D('',#26513,#20848,#20849);
#17920=AXIS2_PLACEMENT_3D('',#26528,#20853,#20854);
#17921=AXIS2_PLACEMENT_3D('',#26530,#20855,#20856);
#17922=AXIS2_PLACEMENT_3D('',#26543,#20857,#20858);
#17923=AXIS2_PLACEMENT_3D('',#26545,#20859,#20860);
#17924=AXIS2_PLACEMENT_3D('',#26547,#20862,#20863);
#17925=AXIS2_PLACEMENT_3D('',#26558,#20867,#20868);
#17926=AXIS2_PLACEMENT_3D('',#26560,#20869,#20870);
#17927=AXIS2_PLACEMENT_3D('',#26563,#20872,#20873);
#17928=AXIS2_PLACEMENT_3D('',#26564,#20874,#20875);
#17929=AXIS2_PLACEMENT_3D('',#26572,#20876,#20877);
#17930=AXIS2_PLACEMENT_3D('',#26574,#20879,#20880);
#17931=AXIS2_PLACEMENT_3D('',#26585,#20884,#20885);
#17932=AXIS2_PLACEMENT_3D('',#26587,#20886,#20887);
#17933=AXIS2_PLACEMENT_3D('',#26600,#20888,#20889);
#17934=AXIS2_PLACEMENT_3D('',#26602,#20890,#20891);
#17935=AXIS2_PLACEMENT_3D('',#26604,#20893,#20894);
#17936=AXIS2_PLACEMENT_3D('',#26612,#20897,#20898);
#17937=AXIS2_PLACEMENT_3D('',#26627,#20902,#20903);
#17938=AXIS2_PLACEMENT_3D('',#26629,#20904,#20905);
#17939=AXIS2_PLACEMENT_3D('',#26642,#20906,#20907);
#17940=AXIS2_PLACEMENT_3D('',#26644,#20908,#20909);
#17941=AXIS2_PLACEMENT_3D('',#26646,#20911,#20912);
#17942=AXIS2_PLACEMENT_3D('',#26654,#20915,#20916);
#17943=AXIS2_PLACEMENT_3D('',#26669,#20920,#20921);
#17944=AXIS2_PLACEMENT_3D('',#26671,#20922,#20923);
#17945=AXIS2_PLACEMENT_3D('',#26684,#20924,#20925);
#17946=AXIS2_PLACEMENT_3D('',#26686,#20926,#20927);
#17947=AXIS2_PLACEMENT_3D('',#26688,#20929,#20930);
#17948=AXIS2_PLACEMENT_3D('',#26700,#20934,#20935);
#17949=AXIS2_PLACEMENT_3D('',#26705,#20936,#20937);
#17950=AXIS2_PLACEMENT_3D('',#26706,#20938,#20939);
#17951=AXIS2_PLACEMENT_3D('',#26707,#20940,#20941);
#17952=AXIS2_PLACEMENT_3D('',#26708,#20942,#20943);
#17953=AXIS2_PLACEMENT_3D('',#26709,#20944,#20945);
#17954=AXIS2_PLACEMENT_3D('',#26710,#20946,#20947);
#17955=AXIS2_PLACEMENT_3D('',#26711,#20948,#20949);
#17956=AXIS2_PLACEMENT_3D('',#26712,#20950,#20951);
#17957=AXIS2_PLACEMENT_3D('',#26713,#20952,#20953);
#17958=AXIS2_PLACEMENT_3D('',#26714,#20954,#20955);
#17959=AXIS2_PLACEMENT_3D('',#26715,#20956,#20957);
#17960=AXIS2_PLACEMENT_3D('',#26716,#20958,#20959);
#17961=AXIS2_PLACEMENT_3D('',#26717,#20960,#20961);
#17962=AXIS2_PLACEMENT_3D('',#26718,#20962,#20963);
#17963=AXIS2_PLACEMENT_3D('',#26719,#20964,#20965);
#17964=AXIS2_PLACEMENT_3D('',#26720,#20966,#20967);
#17965=AXIS2_PLACEMENT_3D('',#26721,#20968,#20969);
#17966=AXIS2_PLACEMENT_3D('',#26722,#20970,#20971);
#17967=AXIS2_PLACEMENT_3D('',#26723,#20972,#20973);
#17968=AXIS2_PLACEMENT_3D('',#26724,#20974,#20975);
#17969=AXIS2_PLACEMENT_3D('',#26725,#20976,#20977);
#17970=AXIS2_PLACEMENT_3D('',#26726,#20978,#20979);
#17971=AXIS2_PLACEMENT_3D('',#26730,#20982,#20983);
#17972=AXIS2_PLACEMENT_3D('',#26731,#20984,#20985);
#17973=AXIS2_PLACEMENT_3D('',#26732,#20986,#20987);
#17974=AXIS2_PLACEMENT_3D('',#26733,#20988,#20989);
#17975=AXIS2_PLACEMENT_3D('',#26734,#20990,#20991);
#17976=AXIS2_PLACEMENT_3D('',#26735,#20992,#20993);
#17977=AXIS2_PLACEMENT_3D('',#26736,#20994,#20995);
#17978=AXIS2_PLACEMENT_3D('',#26737,#20996,#20997);
#17979=AXIS2_PLACEMENT_3D('',#26738,#20998,#20999);
#17980=AXIS2_PLACEMENT_3D('',#26739,#21000,#21001);
#17981=AXIS2_PLACEMENT_3D('',#26740,#21002,#21003);
#17982=AXIS2_PLACEMENT_3D('',#26755,#21007,#21008);
#17983=AXIS2_PLACEMENT_3D('',#26757,#21009,#21010);
#17984=AXIS2_PLACEMENT_3D('',#26770,#21011,#21012);
#17985=AXIS2_PLACEMENT_3D('',#26772,#21013,#21014);
#17986=AXIS2_PLACEMENT_3D('',#26774,#21016,#21017);
#17987=AXIS2_PLACEMENT_3D('',#26782,#21020,#21021);
#17988=AXIS2_PLACEMENT_3D('',#26797,#21025,#21026);
#17989=AXIS2_PLACEMENT_3D('',#26799,#21027,#21028);
#17990=AXIS2_PLACEMENT_3D('',#26812,#21029,#21030);
#17991=AXIS2_PLACEMENT_3D('',#26814,#21031,#21032);
#17992=AXIS2_PLACEMENT_3D('',#26816,#21034,#21035);
#17993=AXIS2_PLACEMENT_3D('',#26824,#21038,#21039);
#17994=AXIS2_PLACEMENT_3D('',#26839,#21043,#21044);
#17995=AXIS2_PLACEMENT_3D('',#26841,#21045,#21046);
#17996=AXIS2_PLACEMENT_3D('',#26854,#21047,#21048);
#17997=AXIS2_PLACEMENT_3D('',#26856,#21049,#21050);
#17998=AXIS2_PLACEMENT_3D('',#26858,#21052,#21053);
#17999=AXIS2_PLACEMENT_3D('',#26866,#21056,#21057);
#18000=AXIS2_PLACEMENT_3D('',#26881,#21061,#21062);
#18001=AXIS2_PLACEMENT_3D('',#26883,#21063,#21064);
#18002=AXIS2_PLACEMENT_3D('',#26896,#21065,#21066);
#18003=AXIS2_PLACEMENT_3D('',#26898,#21067,#21068);
#18004=AXIS2_PLACEMENT_3D('',#26900,#21070,#21071);
#18005=AXIS2_PLACEMENT_3D('',#26908,#21074,#21075);
#18006=AXIS2_PLACEMENT_3D('',#26923,#21079,#21080);
#18007=AXIS2_PLACEMENT_3D('',#26925,#21081,#21082);
#18008=AXIS2_PLACEMENT_3D('',#26938,#21083,#21084);
#18009=AXIS2_PLACEMENT_3D('',#26940,#21085,#21086);
#18010=AXIS2_PLACEMENT_3D('',#26942,#21088,#21089);
#18011=AXIS2_PLACEMENT_3D('',#26950,#21092,#21093);
#18012=AXIS2_PLACEMENT_3D('',#26965,#21097,#21098);
#18013=AXIS2_PLACEMENT_3D('',#26967,#21099,#21100);
#18014=AXIS2_PLACEMENT_3D('',#26980,#21101,#21102);
#18015=AXIS2_PLACEMENT_3D('',#26982,#21103,#21104);
#18016=AXIS2_PLACEMENT_3D('',#26984,#21106,#21107);
#18017=AXIS2_PLACEMENT_3D('',#26992,#21110,#21111);
#18018=AXIS2_PLACEMENT_3D('',#27007,#21115,#21116);
#18019=AXIS2_PLACEMENT_3D('',#27009,#21117,#21118);
#18020=AXIS2_PLACEMENT_3D('',#27022,#21119,#21120);
#18021=AXIS2_PLACEMENT_3D('',#27024,#21121,#21122);
#18022=AXIS2_PLACEMENT_3D('',#27026,#21124,#21125);
#18023=AXIS2_PLACEMENT_3D('',#27037,#21129,#21130);
#18024=AXIS2_PLACEMENT_3D('',#27039,#21131,#21132);
#18025=AXIS2_PLACEMENT_3D('',#27042,#21134,#21135);
#18026=AXIS2_PLACEMENT_3D('',#27043,#21136,#21137);
#18027=AXIS2_PLACEMENT_3D('',#27051,#21138,#21139);
#18028=AXIS2_PLACEMENT_3D('',#27053,#21141,#21142);
#18029=AXIS2_PLACEMENT_3D('',#27064,#21146,#21147);
#18030=AXIS2_PLACEMENT_3D('',#27066,#21148,#21149);
#18031=AXIS2_PLACEMENT_3D('',#27079,#21150,#21151);
#18032=AXIS2_PLACEMENT_3D('',#27081,#21152,#21153);
#18033=AXIS2_PLACEMENT_3D('',#27083,#21155,#21156);
#18034=AXIS2_PLACEMENT_3D('',#27091,#21159,#21160);
#18035=AXIS2_PLACEMENT_3D('',#27106,#21164,#21165);
#18036=AXIS2_PLACEMENT_3D('',#27108,#21166,#21167);
#18037=AXIS2_PLACEMENT_3D('',#27121,#21168,#21169);
#18038=AXIS2_PLACEMENT_3D('',#27123,#21170,#21171);
#18039=AXIS2_PLACEMENT_3D('',#27125,#21173,#21174);
#18040=AXIS2_PLACEMENT_3D('',#27137,#21178,#21179);
#18041=AXIS2_PLACEMENT_3D('',#27142,#21180,#21181);
#18042=AXIS2_PLACEMENT_3D('',#27143,#21182,#21183);
#18043=AXIS2_PLACEMENT_3D('',#27144,#21184,#21185);
#18044=AXIS2_PLACEMENT_3D('',#27145,#21186,#21187);
#18045=AXIS2_PLACEMENT_3D('',#27146,#21188,#21189);
#18046=AXIS2_PLACEMENT_3D('',#27147,#21190,#21191);
#18047=AXIS2_PLACEMENT_3D('',#27148,#21192,#21193);
#18048=AXIS2_PLACEMENT_3D('',#27149,#21194,#21195);
#18049=AXIS2_PLACEMENT_3D('',#27150,#21196,#21197);
#18050=AXIS2_PLACEMENT_3D('',#27151,#21198,#21199);
#18051=AXIS2_PLACEMENT_3D('',#27152,#21200,#21201);
#18052=AXIS2_PLACEMENT_3D('',#27153,#21202,#21203);
#18053=AXIS2_PLACEMENT_3D('',#27154,#21204,#21205);
#18054=AXIS2_PLACEMENT_3D('',#27155,#21206,#21207);
#18055=AXIS2_PLACEMENT_3D('',#27156,#21208,#21209);
#18056=AXIS2_PLACEMENT_3D('',#27157,#21210,#21211);
#18057=AXIS2_PLACEMENT_3D('',#27158,#21212,#21213);
#18058=AXIS2_PLACEMENT_3D('',#27159,#21214,#21215);
#18059=AXIS2_PLACEMENT_3D('',#27160,#21216,#21217);
#18060=AXIS2_PLACEMENT_3D('',#27161,#21218,#21219);
#18061=AXIS2_PLACEMENT_3D('',#27162,#21220,#21221);
#18062=AXIS2_PLACEMENT_3D('',#27163,#21222,#21223);
#18063=AXIS2_PLACEMENT_3D('',#27164,#21224,#21225);
#18064=AXIS2_PLACEMENT_3D('',#27165,#21226,#21227);
#18065=AXIS2_PLACEMENT_3D('',#27166,#21228,#21229);
#18066=AXIS2_PLACEMENT_3D('',#27167,#21230,#21231);
#18067=AXIS2_PLACEMENT_3D('',#27168,#21232,#21233);
#18068=AXIS2_PLACEMENT_3D('',#27169,#21234,#21235);
#18069=AXIS2_PLACEMENT_3D('',#27173,#21238,#21239);
#18070=AXIS2_PLACEMENT_3D('',#27174,#21240,#21241);
#18071=AXIS2_PLACEMENT_3D('',#27175,#21242,#21243);
#18072=AXIS2_PLACEMENT_3D('',#27176,#21244,#21245);
#18073=AXIS2_PLACEMENT_3D('',#27177,#21246,#21247);
#18074=AXIS2_PLACEMENT_3D('',#27178,#21248,#21249);
#18075=AXIS2_PLACEMENT_3D('',#27179,#21250,#21251);
#18076=AXIS2_PLACEMENT_3D('',#27194,#21255,#21256);
#18077=AXIS2_PLACEMENT_3D('',#27196,#21257,#21258);
#18078=AXIS2_PLACEMENT_3D('',#27209,#21259,#21260);
#18079=AXIS2_PLACEMENT_3D('',#27211,#21261,#21262);
#18080=AXIS2_PLACEMENT_3D('',#27213,#21264,#21265);
#18081=AXIS2_PLACEMENT_3D('',#27221,#21268,#21269);
#18082=AXIS2_PLACEMENT_3D('',#27236,#21273,#21274);
#18083=AXIS2_PLACEMENT_3D('',#27238,#21275,#21276);
#18084=AXIS2_PLACEMENT_3D('',#27251,#21277,#21278);
#18085=AXIS2_PLACEMENT_3D('',#27253,#21279,#21280);
#18086=AXIS2_PLACEMENT_3D('',#27255,#21282,#21283);
#18087=AXIS2_PLACEMENT_3D('',#27263,#21286,#21287);
#18088=AXIS2_PLACEMENT_3D('',#27278,#21291,#21292);
#18089=AXIS2_PLACEMENT_3D('',#27280,#21293,#21294);
#18090=AXIS2_PLACEMENT_3D('',#27293,#21295,#21296);
#18091=AXIS2_PLACEMENT_3D('',#27295,#21297,#21298);
#18092=AXIS2_PLACEMENT_3D('',#27297,#21300,#21301);
#18093=AXIS2_PLACEMENT_3D('',#27305,#21304,#21305);
#18094=AXIS2_PLACEMENT_3D('',#27320,#21309,#21310);
#18095=AXIS2_PLACEMENT_3D('',#27322,#21311,#21312);
#18096=AXIS2_PLACEMENT_3D('',#27335,#21313,#21314);
#18097=AXIS2_PLACEMENT_3D('',#27337,#21315,#21316);
#18098=AXIS2_PLACEMENT_3D('',#27339,#21318,#21319);
#18099=AXIS2_PLACEMENT_3D('',#27347,#21322,#21323);
#18100=AXIS2_PLACEMENT_3D('',#27362,#21327,#21328);
#18101=AXIS2_PLACEMENT_3D('',#27364,#21329,#21330);
#18102=AXIS2_PLACEMENT_3D('',#27377,#21331,#21332);
#18103=AXIS2_PLACEMENT_3D('',#27379,#21333,#21334);
#18104=AXIS2_PLACEMENT_3D('',#27381,#21336,#21337);
#18105=AXIS2_PLACEMENT_3D('',#27389,#21340,#21341);
#18106=AXIS2_PLACEMENT_3D('',#27404,#21345,#21346);
#18107=AXIS2_PLACEMENT_3D('',#27406,#21347,#21348);
#18108=AXIS2_PLACEMENT_3D('',#27419,#21349,#21350);
#18109=AXIS2_PLACEMENT_3D('',#27421,#21351,#21352);
#18110=AXIS2_PLACEMENT_3D('',#27423,#21354,#21355);
#18111=AXIS2_PLACEMENT_3D('',#27431,#21358,#21359);
#18112=AXIS2_PLACEMENT_3D('',#27446,#21363,#21364);
#18113=AXIS2_PLACEMENT_3D('',#27448,#21365,#21366);
#18114=AXIS2_PLACEMENT_3D('',#27461,#21367,#21368);
#18115=AXIS2_PLACEMENT_3D('',#27463,#21369,#21370);
#18116=AXIS2_PLACEMENT_3D('',#27465,#21372,#21373);
#18117=AXIS2_PLACEMENT_3D('',#27473,#21376,#21377);
#18118=AXIS2_PLACEMENT_3D('',#27488,#21381,#21382);
#18119=AXIS2_PLACEMENT_3D('',#27490,#21383,#21384);
#18120=AXIS2_PLACEMENT_3D('',#27503,#21385,#21386);
#18121=AXIS2_PLACEMENT_3D('',#27505,#21387,#21388);
#18122=AXIS2_PLACEMENT_3D('',#27507,#21390,#21391);
#18123=AXIS2_PLACEMENT_3D('',#27518,#21395,#21396);
#18124=AXIS2_PLACEMENT_3D('',#27520,#21397,#21398);
#18125=AXIS2_PLACEMENT_3D('',#27523,#21400,#21401);
#18126=AXIS2_PLACEMENT_3D('',#27524,#21402,#21403);
#18127=AXIS2_PLACEMENT_3D('',#27532,#21404,#21405);
#18128=AXIS2_PLACEMENT_3D('',#27534,#21407,#21408);
#18129=AXIS2_PLACEMENT_3D('',#27545,#21412,#21413);
#18130=AXIS2_PLACEMENT_3D('',#27547,#21414,#21415);
#18131=AXIS2_PLACEMENT_3D('',#27560,#21416,#21417);
#18132=AXIS2_PLACEMENT_3D('',#27562,#21418,#21419);
#18133=AXIS2_PLACEMENT_3D('',#27564,#21421,#21422);
#18134=AXIS2_PLACEMENT_3D('',#27576,#21426,#21427);
#18135=AXIS2_PLACEMENT_3D('',#27581,#21428,#21429);
#18136=AXIS2_PLACEMENT_3D('',#27582,#21430,#21431);
#18137=AXIS2_PLACEMENT_3D('',#27583,#21432,#21433);
#18138=AXIS2_PLACEMENT_3D('',#27584,#21434,#21435);
#18139=AXIS2_PLACEMENT_3D('',#27585,#21436,#21437);
#18140=AXIS2_PLACEMENT_3D('',#27586,#21438,#21439);
#18141=AXIS2_PLACEMENT_3D('',#27587,#21440,#21441);
#18142=AXIS2_PLACEMENT_3D('',#27588,#21442,#21443);
#18143=AXIS2_PLACEMENT_3D('',#27589,#21444,#21445);
#18144=AXIS2_PLACEMENT_3D('',#27590,#21446,#21447);
#18145=AXIS2_PLACEMENT_3D('',#27591,#21448,#21449);
#18146=AXIS2_PLACEMENT_3D('',#27592,#21450,#21451);
#18147=AXIS2_PLACEMENT_3D('',#27593,#21452,#21453);
#18148=AXIS2_PLACEMENT_3D('',#27594,#21454,#21455);
#18149=AXIS2_PLACEMENT_3D('',#27595,#21456,#21457);
#18150=AXIS2_PLACEMENT_3D('',#27596,#21458,#21459);
#18151=AXIS2_PLACEMENT_3D('',#27597,#21460,#21461);
#18152=AXIS2_PLACEMENT_3D('',#27598,#21462,#21463);
#18153=AXIS2_PLACEMENT_3D('',#27599,#21464,#21465);
#18154=AXIS2_PLACEMENT_3D('',#27600,#21466,#21467);
#18155=AXIS2_PLACEMENT_3D('',#27601,#21468,#21469);
#18156=AXIS2_PLACEMENT_3D('',#27602,#21470,#21471);
#18157=AXIS2_PLACEMENT_3D('',#27603,#21472,#21473);
#18158=AXIS2_PLACEMENT_3D('',#27604,#21474,#21475);
#18159=AXIS2_PLACEMENT_3D('',#27605,#21476,#21477);
#18160=AXIS2_PLACEMENT_3D('',#27606,#21478,#21479);
#18161=AXIS2_PLACEMENT_3D('',#27607,#21480,#21481);
#18162=AXIS2_PLACEMENT_3D('',#27608,#21482,#21483);
#18163=AXIS2_PLACEMENT_3D('',#27609,#21484,#21485);
#18164=AXIS2_PLACEMENT_3D('',#27610,#21486,#21487);
#18165=AXIS2_PLACEMENT_3D('',#27611,#21488,#21489);
#18166=AXIS2_PLACEMENT_3D('',#27612,#21490,#21491);
#18167=AXIS2_PLACEMENT_3D('',#27616,#21494,#21495);
#18168=AXIS2_PLACEMENT_3D('',#27617,#21496,#21497);
#18169=AXIS2_PLACEMENT_3D('',#27618,#21498,#21499);
#18170=AXIS2_PLACEMENT_3D('',#27628,#21503,#21504);
#18171=AXIS2_PLACEMENT_3D('',#27630,#21505,#21506);
#18172=AXIS2_PLACEMENT_3D('',#27639,#21507,#21508);
#18173=AXIS2_PLACEMENT_3D('',#27641,#21509,#21510);
#18174=AXIS2_PLACEMENT_3D('',#27643,#21512,#21513);
#18175=AXIS2_PLACEMENT_3D('',#27651,#21516,#21517);
#18176=AXIS2_PLACEMENT_3D('',#27666,#21521,#21522);
#18177=AXIS2_PLACEMENT_3D('',#27668,#21523,#21524);
#18178=AXIS2_PLACEMENT_3D('',#27681,#21525,#21526);
#18179=AXIS2_PLACEMENT_3D('',#27683,#21527,#21528);
#18180=AXIS2_PLACEMENT_3D('',#27685,#21530,#21531);
#18181=AXIS2_PLACEMENT_3D('',#27693,#21534,#21535);
#18182=AXIS2_PLACEMENT_3D('',#27708,#21539,#21540);
#18183=AXIS2_PLACEMENT_3D('',#27710,#21541,#21542);
#18184=AXIS2_PLACEMENT_3D('',#27723,#21543,#21544);
#18185=AXIS2_PLACEMENT_3D('',#27725,#21545,#21546);
#18186=AXIS2_PLACEMENT_3D('',#27727,#21548,#21549);
#18187=AXIS2_PLACEMENT_3D('',#27735,#21552,#21553);
#18188=AXIS2_PLACEMENT_3D('',#27750,#21557,#21558);
#18189=AXIS2_PLACEMENT_3D('',#27752,#21559,#21560);
#18190=AXIS2_PLACEMENT_3D('',#27765,#21561,#21562);
#18191=AXIS2_PLACEMENT_3D('',#27767,#21563,#21564);
#18192=AXIS2_PLACEMENT_3D('',#27769,#21566,#21567);
#18193=AXIS2_PLACEMENT_3D('',#27777,#21570,#21571);
#18194=AXIS2_PLACEMENT_3D('',#27792,#21575,#21576);
#18195=AXIS2_PLACEMENT_3D('',#27794,#21577,#21578);
#18196=AXIS2_PLACEMENT_3D('',#27807,#21579,#21580);
#18197=AXIS2_PLACEMENT_3D('',#27809,#21581,#21582);
#18198=AXIS2_PLACEMENT_3D('',#27811,#21584,#21585);
#18199=AXIS2_PLACEMENT_3D('',#27819,#21588,#21589);
#18200=AXIS2_PLACEMENT_3D('',#27834,#21593,#21594);
#18201=AXIS2_PLACEMENT_3D('',#27836,#21595,#21596);
#18202=AXIS2_PLACEMENT_3D('',#27849,#21597,#21598);
#18203=AXIS2_PLACEMENT_3D('',#27851,#21599,#21600);
#18204=AXIS2_PLACEMENT_3D('',#27853,#21602,#21603);
#18205=AXIS2_PLACEMENT_3D('',#27861,#21606,#21607);
#18206=AXIS2_PLACEMENT_3D('',#27876,#21611,#21612);
#18207=AXIS2_PLACEMENT_3D('',#27878,#21613,#21614);
#18208=AXIS2_PLACEMENT_3D('',#27891,#21615,#21616);
#18209=AXIS2_PLACEMENT_3D('',#27893,#21617,#21618);
#18210=AXIS2_PLACEMENT_3D('',#27895,#21620,#21621);
#18211=AXIS2_PLACEMENT_3D('',#27903,#21624,#21625);
#18212=AXIS2_PLACEMENT_3D('',#27918,#21629,#21630);
#18213=AXIS2_PLACEMENT_3D('',#27920,#21631,#21632);
#18214=AXIS2_PLACEMENT_3D('',#27933,#21633,#21634);
#18215=AXIS2_PLACEMENT_3D('',#27935,#21635,#21636);
#18216=AXIS2_PLACEMENT_3D('',#27937,#21638,#21639);
#18217=AXIS2_PLACEMENT_3D('',#27945,#21642,#21643);
#18218=AXIS2_PLACEMENT_3D('',#27960,#21647,#21648);
#18219=AXIS2_PLACEMENT_3D('',#27962,#21649,#21650);
#18220=AXIS2_PLACEMENT_3D('',#27975,#21651,#21652);
#18221=AXIS2_PLACEMENT_3D('',#27977,#21653,#21654);
#18222=AXIS2_PLACEMENT_3D('',#27979,#21656,#21657);
#18223=AXIS2_PLACEMENT_3D('',#27987,#21660,#21661);
#18224=AXIS2_PLACEMENT_3D('',#27989,#21662,#21663);
#18225=AXIS2_PLACEMENT_3D('',#27992,#21665,#21666);
#18226=AXIS2_PLACEMENT_3D('',#27993,#21667,#21668);
#18227=AXIS2_PLACEMENT_3D('',#27997,#21669,#21670);
#18228=AXIS2_PLACEMENT_3D('',#27999,#21672,#21673);
#18229=AXIS2_PLACEMENT_3D('',#28000,#21674,#21675);
#18230=AXIS2_PLACEMENT_3D('',#28001,#21676,#21677);
#18231=AXIS2_PLACEMENT_3D('',#28002,#21678,#21679);
#18232=AXIS2_PLACEMENT_3D('',#28003,#21680,#21681);
#18233=AXIS2_PLACEMENT_3D('',#28004,#21682,#21683);
#18234=AXIS2_PLACEMENT_3D('',#28005,#21684,#21685);
#18235=AXIS2_PLACEMENT_3D('',#28006,#21686,#21687);
#18236=AXIS2_PLACEMENT_3D('',#28007,#21688,#21689);
#18237=AXIS2_PLACEMENT_3D('',#28008,#21690,#21691);
#18238=AXIS2_PLACEMENT_3D('',#28009,#21692,#21693);
#18239=AXIS2_PLACEMENT_3D('',#28010,#21694,#21695);
#18240=AXIS2_PLACEMENT_3D('',#28011,#21696,#21697);
#18241=AXIS2_PLACEMENT_3D('',#28012,#21698,#21699);
#18242=AXIS2_PLACEMENT_3D('',#28013,#21700,#21701);
#18243=AXIS2_PLACEMENT_3D('',#28014,#21702,#21703);
#18244=AXIS2_PLACEMENT_3D('',#28015,#21704,#21705);
#18245=AXIS2_PLACEMENT_3D('',#28016,#21706,#21707);
#18246=AXIS2_PLACEMENT_3D('',#28017,#21708,#21709);
#18247=AXIS2_PLACEMENT_3D('',#28018,#21710,#21711);
#18248=AXIS2_PLACEMENT_3D('',#28019,#21712,#21713);
#18249=AXIS2_PLACEMENT_3D('',#28020,#21714,#21715);
#18250=AXIS2_PLACEMENT_3D('',#28021,#21716,#21717);
#18251=AXIS2_PLACEMENT_3D('',#28022,#21718,#21719);
#18252=AXIS2_PLACEMENT_3D('',#28023,#21720,#21721);
#18253=AXIS2_PLACEMENT_3D('',#28024,#21722,#21723);
#18254=AXIS2_PLACEMENT_3D('',#28025,#21724,#21725);
#18255=AXIS2_PLACEMENT_3D('',#28026,#21726,#21727);
#18256=AXIS2_PLACEMENT_3D('',#28027,#21728,#21729);
#18257=AXIS2_PLACEMENT_3D('',#28028,#21730,#21731);
#18258=AXIS2_PLACEMENT_3D('',#28029,#21732,#21733);
#18259=AXIS2_PLACEMENT_3D('',#28030,#21734,#21735);
#18260=AXIS2_PLACEMENT_3D('',#28031,#21736,#21737);
#18261=AXIS2_PLACEMENT_3D('',#28033,#21738,#21739);
#18262=AXIS2_PLACEMENT_3D('',#28035,#21741,#21742);
#18263=AXIS2_PLACEMENT_3D('',#28037,#21743,#21744);
#18264=AXIS2_PLACEMENT_3D('',#28039,#21746,#21747);
#18265=AXIS2_PLACEMENT_3D('',#28043,#21750,#21751);
#18266=AXIS2_PLACEMENT_3D('',#28044,#21752,#21753);
#18267=AXIS2_PLACEMENT_3D('',#28045,#21754,#21755);
#18268=AXIS2_PLACEMENT_3D('',#28046,#21756,#21757);
#18269=AXIS2_PLACEMENT_3D('',#28047,#21758,#21759);
#18270=AXIS2_PLACEMENT_3D('',#28048,#21760,#21761);
#18271=AXIS2_PLACEMENT_3D('',#28049,#21762,#21763);
#18272=AXIS2_PLACEMENT_3D('',#28050,#21764,#21765);
#18273=AXIS2_PLACEMENT_3D('',#28051,#21766,#21767);
#18274=AXIS2_PLACEMENT_3D('',#28052,#21768,#21769);
#18275=AXIS2_PLACEMENT_3D('',#28053,#21770,#21771);
#18276=AXIS2_PLACEMENT_3D('',#28054,#21772,#21773);
#18277=AXIS2_PLACEMENT_3D('',#28055,#21774,#21775);
#18278=AXIS2_PLACEMENT_3D('',#28056,#21776,#21777);
#18279=AXIS2_PLACEMENT_3D('',#28057,#21778,#21779);
#18280=AXIS2_PLACEMENT_3D('',#28058,#21780,#21781);
#18281=AXIS2_PLACEMENT_3D('',#28059,#21782,#21783);
#18282=AXIS2_PLACEMENT_3D('',#28060,#21784,#21785);
#18283=AXIS2_PLACEMENT_3D('',#28061,#21786,#21787);
#18284=AXIS2_PLACEMENT_3D('',#28062,#21788,#21789);
#18285=AXIS2_PLACEMENT_3D('',#28063,#21790,#21791);
#18286=AXIS2_PLACEMENT_3D('',#28064,#21792,#21793);
#18287=AXIS2_PLACEMENT_3D('',#28065,#21794,#21795);
#18288=AXIS2_PLACEMENT_3D('',#28066,#21796,#21797);
#18289=AXIS2_PLACEMENT_3D('',#28067,#21798,#21799);
#18290=AXIS2_PLACEMENT_3D('',#28068,#21800,#21801);
#18291=AXIS2_PLACEMENT_3D('',#28069,#21802,#21803);
#18292=AXIS2_PLACEMENT_3D('',#28070,#21804,#21805);
#18293=AXIS2_PLACEMENT_3D('',#28071,#21806,#21807);
#18294=AXIS2_PLACEMENT_3D('',#28072,#21808,#21809);
#18295=AXIS2_PLACEMENT_3D('',#28073,#21810,#21811);
#18296=AXIS2_PLACEMENT_3D('',#28074,#21812,#21813);
#18297=AXIS2_PLACEMENT_3D('',#28075,#21814,#21815);
#18298=AXIS2_PLACEMENT_3D('',#28076,#21816,#21817);
#18299=AXIS2_PLACEMENT_3D('',#28077,#21818,#21819);
#18300=AXIS2_PLACEMENT_3D('',#28083,#21823,#21824);
#18301=AXIS2_PLACEMENT_3D('',#28084,#21825,#21826);
#18302=AXIS2_PLACEMENT_3D('',#28085,#21827,#21828);
#18303=AXIS2_PLACEMENT_3D('',#28094,#21831,#21832);
#18304=AXIS2_PLACEMENT_3D('',#28096,#21833,#21834);
#18305=AXIS2_PLACEMENT_3D('',#28106,#21835,#21836);
#18306=AXIS2_PLACEMENT_3D('',#28112,#21840,#21841);
#18307=AXIS2_PLACEMENT_3D('',#28114,#21842,#21843);
#18308=AXIS2_PLACEMENT_3D('',#28121,#21845,#21846);
#18309=AXIS2_PLACEMENT_3D('',#28133,#21850,#21851);
#18310=AXIS2_PLACEMENT_3D('',#28135,#21852,#21853);
#18311=AXIS2_PLACEMENT_3D('',#28144,#21854,#21855);
#18312=AXIS2_PLACEMENT_3D('',#28148,#21858,#21859);
#18313=AXIS2_PLACEMENT_3D('',#28156,#21861,#21862);
#18314=AXIS2_PLACEMENT_3D('',#28157,#21863,#21864);
#18315=AXIS2_PLACEMENT_3D('',#28166,#21867,#21868);
#18316=AXIS2_PLACEMENT_3D('',#28168,#21869,#21870);
#18317=AXIS2_PLACEMENT_3D('',#28178,#21871,#21872);
#18318=AXIS2_PLACEMENT_3D('',#28184,#21876,#21877);
#18319=AXIS2_PLACEMENT_3D('',#28186,#21878,#21879);
#18320=AXIS2_PLACEMENT_3D('',#28193,#21881,#21882);
#18321=AXIS2_PLACEMENT_3D('',#28205,#21886,#21887);
#18322=AXIS2_PLACEMENT_3D('',#28207,#21888,#21889);
#18323=AXIS2_PLACEMENT_3D('',#28216,#21890,#21891);
#18324=AXIS2_PLACEMENT_3D('',#28220,#21894,#21895);
#18325=AXIS2_PLACEMENT_3D('',#28228,#21897,#21898);
#18326=AXIS2_PLACEMENT_3D('',#28229,#21899,#21900);
#18327=AXIS2_PLACEMENT_3D('',#28238,#21903,#21904);
#18328=AXIS2_PLACEMENT_3D('',#28240,#21905,#21906);
#18329=AXIS2_PLACEMENT_3D('',#28250,#21907,#21908);
#18330=AXIS2_PLACEMENT_3D('',#28256,#21912,#21913);
#18331=AXIS2_PLACEMENT_3D('',#28258,#21914,#21915);
#18332=AXIS2_PLACEMENT_3D('',#28265,#21917,#21918);
#18333=AXIS2_PLACEMENT_3D('',#28274,#21921,#21922);
#18334=AXIS2_PLACEMENT_3D('',#28276,#21923,#21924);
#18335=AXIS2_PLACEMENT_3D('',#28281,#21925,#21926);
#18336=AXIS2_PLACEMENT_3D('',#28285,#21929,#21930);
#18337=AXIS2_PLACEMENT_3D('',#28287,#21931,#21932);
#18338=AXIS2_PLACEMENT_3D('',#28290,#21934,#21935);
#18339=AXIS2_PLACEMENT_3D('',#28291,#21936,#21937);
#18340=AXIS2_PLACEMENT_3D('',#28293,#21938,#21939);
#18341=AXIS2_PLACEMENT_3D('',#28294,#21940,#21941);
#18342=AXIS2_PLACEMENT_3D('',#28297,#21943,#21944);
#18343=AXIS2_PLACEMENT_3D('',#28298,#21945,#21946);
#18344=AXIS2_PLACEMENT_3D('',#28299,#21947,#21948);
#18345=AXIS2_PLACEMENT_3D('',#28300,#21949,#21950);
#18346=AXIS2_PLACEMENT_3D('',#28301,#21951,#21952);
#18347=AXIS2_PLACEMENT_3D('',#28302,#21953,#21954);
#18348=AXIS2_PLACEMENT_3D('',#28303,#21955,#21956);
#18349=AXIS2_PLACEMENT_3D('',#28304,#21957,#21958);
#18350=AXIS2_PLACEMENT_3D('',#28305,#21959,#21960);
#18351=AXIS2_PLACEMENT_3D('',#28306,#21961,#21962);
#18352=AXIS2_PLACEMENT_3D('',#28307,#21963,#21964);
#18353=AXIS2_PLACEMENT_3D('',#28308,#21965,#21966);
#18354=AXIS2_PLACEMENT_3D('',#28309,#21967,#21968);
#18355=AXIS2_PLACEMENT_3D('',#28310,#21969,#21970);
#18356=AXIS2_PLACEMENT_3D('',#28311,#21971,#21972);
#18357=AXIS2_PLACEMENT_3D('',#28312,#21973,#21974);
#18358=AXIS2_PLACEMENT_3D('',#28313,#21975,#21976);
#18359=AXIS2_PLACEMENT_3D('',#28314,#21977,#21978);
#18360=AXIS2_PLACEMENT_3D('',#28315,#21979,#21980);
#18361=AXIS2_PLACEMENT_3D('',#28316,#21981,#21982);
#18362=AXIS2_PLACEMENT_3D('',#28317,#21983,#21984);
#18363=AXIS2_PLACEMENT_3D('',#28318,#21985,#21986);
#18364=AXIS2_PLACEMENT_3D('',#28319,#21987,#21988);
#18365=AXIS2_PLACEMENT_3D('',#28320,#21989,#21990);
#18366=AXIS2_PLACEMENT_3D('',#28321,#21991,#21992);
#18367=AXIS2_PLACEMENT_3D('',#28322,#21993,#21994);
#18368=AXIS2_PLACEMENT_3D('',#28323,#21995,#21996);
#18369=AXIS2_PLACEMENT_3D('',#28324,#21997,#21998);
#18370=AXIS2_PLACEMENT_3D('',#28325,#21999,#22000);
#18371=AXIS2_PLACEMENT_3D('',#28326,#22001,#22002);
#18372=AXIS2_PLACEMENT_3D('',#28327,#22003,#22004);
#18373=AXIS2_PLACEMENT_3D('',#28328,#22005,#22006);
#18374=AXIS2_PLACEMENT_3D('',#28329,#22007,#22008);
#18375=AXIS2_PLACEMENT_3D('',#28330,#22009,#22010);
#18376=AXIS2_PLACEMENT_3D('',#28331,#22011,#22012);
#18377=AXIS2_PLACEMENT_3D('',#28332,#22013,#22014);
#18378=AXIS2_PLACEMENT_3D('',#28333,#22015,#22016);
#18379=AXIS2_PLACEMENT_3D('',#28334,#22017,#22018);
#18380=AXIS2_PLACEMENT_3D('',#28335,#22019,#22020);
#18381=AXIS2_PLACEMENT_3D('',#28336,#22021,#22022);
#18382=AXIS2_PLACEMENT_3D('',#28337,#22023,#22024);
#18383=AXIS2_PLACEMENT_3D('',#28338,#22025,#22026);
#18384=AXIS2_PLACEMENT_3D('',#28339,#22027,#22028);
#18385=AXIS2_PLACEMENT_3D('',#28340,#22029,#22030);
#18386=AXIS2_PLACEMENT_3D('',#28341,#22031,#22032);
#18387=AXIS2_PLACEMENT_3D('',#28342,#22033,#22034);
#18388=AXIS2_PLACEMENT_3D('',#28343,#22035,#22036);
#18389=AXIS2_PLACEMENT_3D('',#28344,#22037,#22038);
#18390=AXIS2_PLACEMENT_3D('',#28345,#22039,#22040);
#18391=AXIS2_PLACEMENT_3D('',#28346,#22041,#22042);
#18392=AXIS2_PLACEMENT_3D('',#28347,#22043,#22044);
#18393=AXIS2_PLACEMENT_3D('',#28348,#22045,#22046);
#18394=AXIS2_PLACEMENT_3D('',#28349,#22047,#22048);
#18395=AXIS2_PLACEMENT_3D('',#28350,#22049,#22050);
#18396=AXIS2_PLACEMENT_3D('',#28351,#22051,#22052);
#18397=AXIS2_PLACEMENT_3D('',#28352,#22053,#22054);
#18398=AXIS2_PLACEMENT_3D('',#28353,#22055,#22056);
#18399=AXIS2_PLACEMENT_3D('',#28354,#22057,#22058);
#18400=AXIS2_PLACEMENT_3D('',#28355,#22059,#22060);
#18401=AXIS2_PLACEMENT_3D('',#28356,#22061,#22062);
#18402=AXIS2_PLACEMENT_3D('',#28357,#22063,#22064);
#18403=AXIS2_PLACEMENT_3D('',#28358,#22065,#22066);
#18404=AXIS2_PLACEMENT_3D('',#28359,#22067,#22068);
#18405=AXIS2_PLACEMENT_3D('',#28360,#22069,#22070);
#18406=AXIS2_PLACEMENT_3D('',#28361,#22071,#22072);
#18407=AXIS2_PLACEMENT_3D('',#28362,#22073,#22074);
#18408=AXIS2_PLACEMENT_3D('',#28363,#22075,#22076);
#18409=AXIS2_PLACEMENT_3D('',#28364,#22077,#22078);
#18410=AXIS2_PLACEMENT_3D('',#28365,#22079,#22080);
#18411=AXIS2_PLACEMENT_3D('',#28366,#22081,#22082);
#18412=AXIS2_PLACEMENT_3D('',#28367,#22083,#22084);
#18413=AXIS2_PLACEMENT_3D('',#28368,#22085,#22086);
#18414=AXIS2_PLACEMENT_3D('',#28369,#22087,#22088);
#18415=AXIS2_PLACEMENT_3D('',#28370,#22089,#22090);
#18416=AXIS2_PLACEMENT_3D('',#28371,#22091,#22092);
#18417=AXIS2_PLACEMENT_3D('',#28372,#22093,#22094);
#18418=AXIS2_PLACEMENT_3D('',#28373,#22095,#22096);
#18419=AXIS2_PLACEMENT_3D('',#28374,#22097,#22098);
#18420=AXIS2_PLACEMENT_3D('',#28375,#22099,#22100);
#18421=AXIS2_PLACEMENT_3D('',#28376,#22101,#22102);
#18422=AXIS2_PLACEMENT_3D('',#28377,#22103,#22104);
#18423=AXIS2_PLACEMENT_3D('',#28378,#22105,#22106);
#18424=AXIS2_PLACEMENT_3D('',#28379,#22107,#22108);
#18425=AXIS2_PLACEMENT_3D('',#28380,#22109,#22110);
#18426=AXIS2_PLACEMENT_3D('',#28381,#22111,#22112);
#18427=AXIS2_PLACEMENT_3D('',#28382,#22113,#22114);
#18428=AXIS2_PLACEMENT_3D('',#28383,#22115,#22116);
#18429=AXIS2_PLACEMENT_3D('',#28384,#22117,#22118);
#18430=AXIS2_PLACEMENT_3D('',#28385,#22119,#22120);
#18431=AXIS2_PLACEMENT_3D('',#28386,#22121,#22122);
#18432=AXIS2_PLACEMENT_3D('',#28387,#22123,#22124);
#18433=AXIS2_PLACEMENT_3D('',#28388,#22125,#22126);
#18434=AXIS2_PLACEMENT_3D('',#28389,#22127,#22128);
#18435=AXIS2_PLACEMENT_3D('',#28390,#22129,#22130);
#18436=AXIS2_PLACEMENT_3D('',#28391,#22131,#22132);
#18437=AXIS2_PLACEMENT_3D('',#28392,#22133,#22134);
#18438=AXIS2_PLACEMENT_3D('',#28393,#22135,#22136);
#18439=AXIS2_PLACEMENT_3D('',#28394,#22137,#22138);
#18440=AXIS2_PLACEMENT_3D('',#28395,#22139,#22140);
#18441=AXIS2_PLACEMENT_3D('',#28396,#22141,#22142);
#18442=AXIS2_PLACEMENT_3D('',#28397,#22143,#22144);
#18443=AXIS2_PLACEMENT_3D('',#28398,#22145,#22146);
#18444=AXIS2_PLACEMENT_3D('',#28400,#22147,#22148);
#18445=AXIS2_PLACEMENT_3D('',#28403,#22150,#22151);
#18446=AXIS2_PLACEMENT_3D('',#28404,#22152,#22153);
#18447=AXIS2_PLACEMENT_3D('',#28406,#22154,#22155);
#18448=AXIS2_PLACEMENT_3D('',#28408,#22156,#22157);
#18449=AXIS2_PLACEMENT_3D('',#28410,#22158,#22159);
#18450=AXIS2_PLACEMENT_3D('',#28412,#22160,#22161);
#18451=AXIS2_PLACEMENT_3D('',#28414,#22162,#22163);
#18452=AXIS2_PLACEMENT_3D('',#28416,#22164,#22165);
#18453=AXIS2_PLACEMENT_3D('',#28417,#22166,#22167);
#18454=AXIS2_PLACEMENT_3D('',#28420,#22169,#22170);
#18455=AXIS2_PLACEMENT_3D('',#28421,#22171,#22172);
#18456=AXIS2_PLACEMENT_3D('',#28424,#22174,#22175);
#18457=AXIS2_PLACEMENT_3D('',#28425,#22176,#22177);
#18458=AXIS2_PLACEMENT_3D('',#28428,#22179,#22180);
#18459=AXIS2_PLACEMENT_3D('',#28429,#22181,#22182);
#18460=AXIS2_PLACEMENT_3D('',#28432,#22184,#22185);
#18461=AXIS2_PLACEMENT_3D('',#28433,#22186,#22187);
#18462=AXIS2_PLACEMENT_3D('',#28436,#22189,#22190);
#18463=AXIS2_PLACEMENT_3D('',#28437,#22191,#22192);
#18464=AXIS2_PLACEMENT_3D('',#28440,#22194,#22195);
#18465=AXIS2_PLACEMENT_3D('',#28441,#22196,#22197);
#18466=AXIS2_PLACEMENT_3D('',#28444,#22199,#22200);
#18467=AXIS2_PLACEMENT_3D('',#28445,#22201,#22202);
#18468=AXIS2_PLACEMENT_3D('',#28448,#22204,#22205);
#18469=AXIS2_PLACEMENT_3D('',#28449,#22206,#22207);
#18470=AXIS2_PLACEMENT_3D('',#28452,#22209,#22210);
#18471=AXIS2_PLACEMENT_3D('',#28453,#22211,#22212);
#18472=AXIS2_PLACEMENT_3D('',#28456,#22214,#22215);
#18473=AXIS2_PLACEMENT_3D('',#28457,#22216,#22217);
#18474=AXIS2_PLACEMENT_3D('',#28459,#22219,#22220);
#18475=AXIS2_PLACEMENT_3D('',#28460,#22221,#22222);
#18476=AXIS2_PLACEMENT_3D('',#28461,#22223,#22224);
#18477=AXIS2_PLACEMENT_3D('',#28462,#22225,#22226);
#18478=AXIS2_PLACEMENT_3D('',#28463,#22227,#22228);
#18479=AXIS2_PLACEMENT_3D('',#28464,#22229,#22230);
#18480=AXIS2_PLACEMENT_3D('',#28465,#22231,#22232);
#18481=AXIS2_PLACEMENT_3D('',#28466,#22233,#22234);
#18482=AXIS2_PLACEMENT_3D('',#28467,#22235,#22236);
#18483=AXIS2_PLACEMENT_3D('',#28468,#22237,#22238);
#18484=AXIS2_PLACEMENT_3D('',#28469,#22239,#22240);
#18485=AXIS2_PLACEMENT_3D('',#28470,#22241,#22242);
#18486=AXIS2_PLACEMENT_3D('',#28471,#22243,#22244);
#18487=AXIS2_PLACEMENT_3D('',#28472,#22245,#22246);
#18488=AXIS2_PLACEMENT_3D('',#28473,#22247,#22248);
#18489=AXIS2_PLACEMENT_3D('',#28474,#22249,#22250);
#18490=AXIS2_PLACEMENT_3D('',#28475,#22251,#22252);
#18491=AXIS2_PLACEMENT_3D('',#28476,#22253,#22254);
#18492=AXIS2_PLACEMENT_3D('',#28477,#22255,#22256);
#18493=AXIS2_PLACEMENT_3D('',#28478,#22257,#22258);
#18494=AXIS2_PLACEMENT_3D('',#28479,#22259,#22260);
#18495=AXIS2_PLACEMENT_3D('',#28480,#22261,#22262);
#18496=AXIS2_PLACEMENT_3D('',#28481,#22263,#22264);
#18497=AXIS2_PLACEMENT_3D('',#28482,#22265,#22266);
#18498=AXIS2_PLACEMENT_3D('',#28483,#22267,#22268);
#18499=AXIS2_PLACEMENT_3D('',#28484,#22269,#22270);
#18500=AXIS2_PLACEMENT_3D('',#28485,#22271,#22272);
#18501=AXIS2_PLACEMENT_3D('',#28486,#22273,#22274);
#18502=AXIS2_PLACEMENT_3D('',#28487,#22275,#22276);
#18503=AXIS2_PLACEMENT_3D('',#28488,#22277,#22278);
#18504=AXIS2_PLACEMENT_3D('',#28489,#22279,#22280);
#18505=AXIS2_PLACEMENT_3D('',#28490,#22281,#22282);
#18506=AXIS2_PLACEMENT_3D('',#28491,#22283,#22284);
#18507=AXIS2_PLACEMENT_3D('',#28492,#22285,#22286);
#18508=AXIS2_PLACEMENT_3D('',#28493,#22287,#22288);
#18509=AXIS2_PLACEMENT_3D('',#28494,#22289,#22290);
#18510=AXIS2_PLACEMENT_3D('',#28495,#22291,#22292);
#18511=AXIS2_PLACEMENT_3D('',#28496,#22293,#22294);
#18512=AXIS2_PLACEMENT_3D('',#28497,#22295,#22296);
#18513=AXIS2_PLACEMENT_3D('',#28498,#22297,#22298);
#18514=AXIS2_PLACEMENT_3D('',#28499,#22299,#22300);
#18515=AXIS2_PLACEMENT_3D('',#28500,#22301,#22302);
#18516=AXIS2_PLACEMENT_3D('',#28501,#22303,#22304);
#18517=AXIS2_PLACEMENT_3D('',#28502,#22305,#22306);
#18518=AXIS2_PLACEMENT_3D('',#28503,#22307,#22308);
#18519=AXIS2_PLACEMENT_3D('',#28504,#22309,#22310);
#18520=AXIS2_PLACEMENT_3D('',#28505,#22311,#22312);
#18521=AXIS2_PLACEMENT_3D('',#28506,#22313,#22314);
#18522=AXIS2_PLACEMENT_3D('',#28507,#22315,#22316);
#18523=AXIS2_PLACEMENT_3D('',#28508,#22317,#22318);
#18524=AXIS2_PLACEMENT_3D('',#28509,#22319,#22320);
#18525=AXIS2_PLACEMENT_3D('',#28510,#22321,#22322);
#18526=AXIS2_PLACEMENT_3D('',#28511,#22323,#22324);
#18527=AXIS2_PLACEMENT_3D('',#28512,#22325,#22326);
#18528=AXIS2_PLACEMENT_3D('',#28513,#22327,#22328);
#18529=AXIS2_PLACEMENT_3D('',#28514,#22329,#22330);
#18530=AXIS2_PLACEMENT_3D('',#28515,#22331,#22332);
#18531=AXIS2_PLACEMENT_3D('',#28516,#22333,#22334);
#18532=AXIS2_PLACEMENT_3D('',#28517,#22335,#22336);
#18533=AXIS2_PLACEMENT_3D('',#28518,#22337,#22338);
#18534=AXIS2_PLACEMENT_3D('',#28519,#22339,#22340);
#18535=AXIS2_PLACEMENT_3D('',#28520,#22341,#22342);
#18536=AXIS2_PLACEMENT_3D('',#28521,#22343,#22344);
#18537=AXIS2_PLACEMENT_3D('',#28522,#22345,#22346);
#18538=AXIS2_PLACEMENT_3D('',#28523,#22347,#22348);
#18539=AXIS2_PLACEMENT_3D('',#28524,#22349,#22350);
#18540=AXIS2_PLACEMENT_3D('',#28525,#22351,#22352);
#18541=AXIS2_PLACEMENT_3D('',#28526,#22353,#22354);
#18542=AXIS2_PLACEMENT_3D('',#28527,#22355,#22356);
#18543=AXIS2_PLACEMENT_3D('',#28528,#22357,#22358);
#18544=AXIS2_PLACEMENT_3D('',#28529,#22359,#22360);
#18545=AXIS2_PLACEMENT_3D('',#28530,#22361,#22362);
#18546=AXIS2_PLACEMENT_3D('',#28531,#22363,#22364);
#18547=AXIS2_PLACEMENT_3D('',#28532,#22365,#22366);
#18548=AXIS2_PLACEMENT_3D('',#28533,#22367,#22368);
#18549=AXIS2_PLACEMENT_3D('',#28534,#22369,#22370);
#18550=AXIS2_PLACEMENT_3D('',#28535,#22371,#22372);
#18551=AXIS2_PLACEMENT_3D('',#28536,#22373,#22374);
#18552=AXIS2_PLACEMENT_3D('',#28537,#22375,#22376);
#18553=AXIS2_PLACEMENT_3D('',#28538,#22377,#22378);
#18554=AXIS2_PLACEMENT_3D('',#28539,#22379,#22380);
#18555=AXIS2_PLACEMENT_3D('',#28540,#22381,#22382);
#18556=AXIS2_PLACEMENT_3D('',#28541,#22383,#22384);
#18557=AXIS2_PLACEMENT_3D('',#28542,#22385,#22386);
#18558=AXIS2_PLACEMENT_3D('',#28543,#22387,#22388);
#18559=AXIS2_PLACEMENT_3D('',#28544,#22389,#22390);
#18560=AXIS2_PLACEMENT_3D('',#28545,#22391,#22392);
#18561=AXIS2_PLACEMENT_3D('',#28546,#22393,#22394);
#18562=AXIS2_PLACEMENT_3D('',#28547,#22395,#22396);
#18563=AXIS2_PLACEMENT_3D('',#28548,#22397,#22398);
#18564=AXIS2_PLACEMENT_3D('',#28549,#22399,#22400);
#18565=AXIS2_PLACEMENT_3D('',#28550,#22401,#22402);
#18566=AXIS2_PLACEMENT_3D('',#28551,#22403,#22404);
#18567=AXIS2_PLACEMENT_3D('',#28552,#22405,#22406);
#18568=AXIS2_PLACEMENT_3D('',#28553,#22407,#22408);
#18569=AXIS2_PLACEMENT_3D('',#28554,#22409,#22410);
#18570=AXIS2_PLACEMENT_3D('',#28555,#22411,#22412);
#18571=AXIS2_PLACEMENT_3D('',#28556,#22413,#22414);
#18572=AXIS2_PLACEMENT_3D('',#28557,#22415,#22416);
#18573=AXIS2_PLACEMENT_3D('',#28558,#22417,#22418);
#18574=AXIS2_PLACEMENT_3D('',#28559,#22419,#22420);
#18575=AXIS2_PLACEMENT_3D('',#28560,#22421,#22422);
#18576=AXIS2_PLACEMENT_3D('',#28561,#22423,#22424);
#18577=AXIS2_PLACEMENT_3D('',#28562,#22425,#22426);
#18578=AXIS2_PLACEMENT_3D('',#28563,#22427,#22428);
#18579=AXIS2_PLACEMENT_3D('',#28564,#22429,#22430);
#18580=AXIS2_PLACEMENT_3D('',#28565,#22431,#22432);
#18581=AXIS2_PLACEMENT_3D('',#28566,#22433,#22434);
#18582=AXIS2_PLACEMENT_3D('',#28567,#22435,#22436);
#18583=AXIS2_PLACEMENT_3D('',#28568,#22437,#22438);
#18584=AXIS2_PLACEMENT_3D('',#28569,#22439,#22440);
#18585=AXIS2_PLACEMENT_3D('',#28570,#22441,#22442);
#18586=AXIS2_PLACEMENT_3D('',#28571,#22443,#22444);
#18587=AXIS2_PLACEMENT_3D('',#28573,#22445,#22446);
#18588=AXIS2_PLACEMENT_3D('',#28576,#22448,#22449);
#18589=AXIS2_PLACEMENT_3D('',#28578,#22450,#22451);
#18590=AXIS2_PLACEMENT_3D('',#28581,#22453,#22454);
#18591=AXIS2_PLACEMENT_3D('',#28583,#22455,#22456);
#18592=AXIS2_PLACEMENT_3D('',#28586,#22458,#22459);
#18593=AXIS2_PLACEMENT_3D('',#28588,#22460,#22461);
#18594=AXIS2_PLACEMENT_3D('',#28591,#22463,#22464);
#18595=AXIS2_PLACEMENT_3D('',#28593,#22465,#22466);
#18596=AXIS2_PLACEMENT_3D('',#28596,#22468,#22469);
#18597=AXIS2_PLACEMENT_3D('',#28599,#22471,#22472);
#18598=AXIS2_PLACEMENT_3D('',#28600,#22473,#22474);
#19361=DIRECTION('axis',(0.,0.,1.));
#19362=DIRECTION('refdir',(1.,0.,0.));
#19363=DIRECTION('center_axis',(0.465479050687347,0.885058898249832,0.));
#19364=DIRECTION('ref_axis',(0.,0.,1.));
#19365=DIRECTION('',(0.,0.,1.));
#19366=DIRECTION('',(-0.885058898249832,0.465479050687346,0.));
#19367=DIRECTION('',(0.,0.,-1.));
#19368=DIRECTION('center_axis',(0.,0.,1.));
#19369=DIRECTION('ref_axis',(1.,0.,0.));
#19370=DIRECTION('center_axis',(0.,0.,-1.));
#19371=DIRECTION('ref_axis',(-1.,0.,0.));
#19372=DIRECTION('',(0.,0.,-1.));
#19373=DIRECTION('center_axis',(0.,0.,1.));
#19374=DIRECTION('ref_axis',(1.,0.,0.));
#19375=DIRECTION('center_axis',(0.,0.,1.));
#19376=DIRECTION('ref_axis',(-1.,0.,0.));
#19377=DIRECTION('center_axis',(0.,0.,1.));
#19378=DIRECTION('ref_axis',(-1.,0.,0.));
#19379=DIRECTION('center_axis',(-0.999538253627158,0.0303855152329365,0.));
#19380=DIRECTION('ref_axis',(0.,0.,1.));
#19381=DIRECTION('',(0.,0.,1.));
#19382=DIRECTION('',(-0.0303855152329365,-0.999538253627158,0.));
#19383=DIRECTION('',(0.,0.,-1.));
#19384=DIRECTION('center_axis',(0.,0.,1.));
#19385=DIRECTION('ref_axis',(1.,0.,0.));
#19386=DIRECTION('center_axis',(0.,0.,-1.));
#19387=DIRECTION('ref_axis',(-1.,0.,0.));
#19388=DIRECTION('',(0.,0.,-1.));
#19389=DIRECTION('center_axis',(0.,0.,1.));
#19390=DIRECTION('ref_axis',(1.,0.,0.));
#19391=DIRECTION('center_axis',(0.,0.,1.));
#19392=DIRECTION('ref_axis',(-1.,0.,0.));
#19393=DIRECTION('center_axis',(0.,0.,1.));
#19394=DIRECTION('ref_axis',(-1.,0.,0.));
#19395=DIRECTION('center_axis',(-0.473454498714793,-0.880818277311912,0.));
#19396=DIRECTION('ref_axis',(0.,0.,-1.));
#19397=DIRECTION('',(0.880818277311912,-0.473454498714793,0.));
#19398=DIRECTION('',(0.,0.,1.));
#19399=DIRECTION('center_axis',(0.,0.,1.));
#19400=DIRECTION('ref_axis',(0.848048096156423,0.529919264233209,0.));
#19401=DIRECTION('center_axis',(0.,0.,1.));
#19402=DIRECTION('ref_axis',(-0.848048096156426,-0.529919264233205,0.));
#19403=DIRECTION('',(0.,0.,-1.));
#19404=DIRECTION('center_axis',(0.,0.,1.));
#19405=DIRECTION('ref_axis',(-0.848048096156426,-0.529919264233205,0.));
#19406=DIRECTION('center_axis',(-0.994983842282394,0.100035761590367,0.));
#19407=DIRECTION('ref_axis',(0.,0.,1.));
#19408=DIRECTION('',(0.,0.,1.));
#19409=DIRECTION('',(-0.100035761590367,-0.994983842282394,0.));
#19410=DIRECTION('',(0.,0.,-1.));
#19411=DIRECTION('center_axis',(0.,0.,-1.));
#19412=DIRECTION('ref_axis',(0.913545457642601,0.4067366430758,0.));
#19413=DIRECTION('center_axis',(0.,0.,1.));
#19414=DIRECTION('ref_axis',(0.913545457642601,0.4067366430758,0.));
#19415=DIRECTION('center_axis',(0.,0.,-1.));
#19416=DIRECTION('ref_axis',(0.913545457642601,0.4067366430758,0.));
#19417=DIRECTION('center_axis',(0.,0.,1.));
#19418=DIRECTION('ref_axis',(0.913545457642598,0.406736643075806,0.));
#19419=DIRECTION('center_axis',(0.,0.,1.));
#19420=DIRECTION('ref_axis',(-0.913545457642601,-0.4067366430758,0.));
#19421=DIRECTION('',(0.,0.,1.));
#19422=DIRECTION('center_axis',(-0.533743964386135,-0.845646131949631,0.));
#19423=DIRECTION('ref_axis',(0.,0.,1.));
#19424=DIRECTION('',(0.84564613194963,-0.533743964386135,0.));
#19425=DIRECTION('',(0.,0.,-1.));
#19426=DIRECTION('',(0.,0.,1.));
#19427=DIRECTION('center_axis',(0.,0.,1.));
#19428=DIRECTION('ref_axis',(0.882947592858955,0.469471562785839,0.));
#19429=DIRECTION('center_axis',(0.,0.,1.));
#19430=DIRECTION('ref_axis',(-0.882947592858927,-0.469471562785891,0.));
#19431=DIRECTION('center_axis',(0.,0.,1.));
#19432=DIRECTION('ref_axis',(0.882947592858927,0.469471562785891,0.));
#19433=DIRECTION('center_axis',(0.,0.,-1.));
#19434=DIRECTION('ref_axis',(0.882947592858927,0.469471562785891,0.));
#19435=DIRECTION('center_axis',(0.,0.,-1.));
#19436=DIRECTION('ref_axis',(0.882947592858927,0.469471562785891,0.));
#19437=DIRECTION('center_axis',(-0.985581969673453,0.169198643772926,0.));
#19438=DIRECTION('ref_axis',(0.,0.,1.));
#19439=DIRECTION('',(0.,0.,1.));
#19440=DIRECTION('',(-0.169198643772926,-0.985581969673453,0.));
#19441=DIRECTION('',(0.,0.,-1.));
#19442=DIRECTION('center_axis',(0.,0.,-1.));
#19443=DIRECTION('ref_axis',(0.939692620785908,0.342020143325669,0.));
#19444=DIRECTION('center_axis',(0.,0.,1.));
#19445=DIRECTION('ref_axis',(0.939692620785908,0.342020143325669,0.));
#19446=DIRECTION('center_axis',(0.,0.,-1.));
#19447=DIRECTION('ref_axis',(0.939692620785908,0.342020143325669,0.));
#19448=DIRECTION('center_axis',(0.,0.,1.));
#19449=DIRECTION('ref_axis',(0.939692620785908,0.342020143325671,0.));
#19450=DIRECTION('center_axis',(0.,0.,1.));
#19451=DIRECTION('ref_axis',(-0.939692620785908,-0.342020143325669,0.));
#19452=DIRECTION('',(0.,0.,1.));
#19453=DIRECTION('center_axis',(-0.591433083115112,-0.80635408363631,0.));
#19454=DIRECTION('ref_axis',(0.,0.,1.));
#19455=DIRECTION('',(0.80635408363631,-0.591433083115112,0.));
#19456=DIRECTION('',(0.,0.,-1.));
#19457=DIRECTION('center_axis',(-0.646240799313603,-0.763133559282066,0.));
#19458=DIRECTION('ref_axis',(0.,0.,1.));
#19459=DIRECTION('',(0.763133559282066,-0.646240799313603,0.));
#19460=DIRECTION('',(0.,0.,-1.));
#19461=DIRECTION('center_axis',(-0.928866262851607,-0.370415261208404,0.));
#19462=DIRECTION('ref_axis',(0.,0.,1.));
#19463=DIRECTION('',(0.370415261208404,-0.928866262851607,0.));
#19464=DIRECTION('',(0.,0.,-1.));
#19465=DIRECTION('',(0.,0.,1.));
#19466=DIRECTION('center_axis',(0.,0.,1.));
#19467=DIRECTION('ref_axis',(0.990268068741571,-0.139173100960063,0.));
#19468=DIRECTION('center_axis',(0.,0.,1.));
#19469=DIRECTION('ref_axis',(-0.99026806874157,0.139173100960065,0.));
#19470=DIRECTION('',(0.,0.,-1.));
#19471=DIRECTION('center_axis',(0.,0.,1.));
#19472=DIRECTION('ref_axis',(-0.99026806874157,0.139173100960065,0.));
#19473=DIRECTION('center_axis',(0.,0.,1.));
#19474=DIRECTION('ref_axis',(-1.,0.,0.));
#19475=DIRECTION('center_axis',(0.,0.,-1.));
#19476=DIRECTION('ref_axis',(-1.,0.,0.));
#19477=DIRECTION('center_axis',(0.,0.,1.));
#19478=DIRECTION('ref_axis',(-1.,0.,0.));
#19479=DIRECTION('center_axis',(-0.697900095297593,0.71619512493706,0.));
#19480=DIRECTION('ref_axis',(0.,0.,1.));
#19481=DIRECTION('',(0.,0.,1.));
#19482=DIRECTION('',(-0.71619512493706,-0.697900095297593,0.));
#19483=DIRECTION('',(0.,0.,-1.));
#19484=DIRECTION('center_axis',(0.,0.,1.));
#19485=DIRECTION('ref_axis',(1.,0.,0.));
#19486=DIRECTION('center_axis',(0.,0.,-1.));
#19487=DIRECTION('ref_axis',(-1.,0.,0.));
#19488=DIRECTION('',(0.,0.,-1.));
#19489=DIRECTION('center_axis',(0.,0.,1.));
#19490=DIRECTION('ref_axis',(1.,0.,0.));
#19491=DIRECTION('center_axis',(0.,0.,1.));
#19492=DIRECTION('ref_axis',(-1.,0.,0.));
#19493=DIRECTION('center_axis',(0.,0.,1.));
#19494=DIRECTION('ref_axis',(-1.,0.,0.));
#19495=DIRECTION('center_axis',(-0.971378440778567,-0.237537207171004,0.));
#19496=DIRECTION('ref_axis',(0.,0.,1.));
#19497=DIRECTION('',(0.237537207171004,-0.971378440778567,0.));
#19498=DIRECTION('',(0.,0.,-1.));
#19499=DIRECTION('',(0.,0.,1.));
#19500=DIRECTION('center_axis',(0.,0.,1.));
#19501=DIRECTION('ref_axis',(-1.,0.,0.));
#19502=DIRECTION('center_axis',(0.,0.,-1.));
#19503=DIRECTION('ref_axis',(-1.,0.,0.));
#19504=DIRECTION('center_axis',(0.,0.,1.));
#19505=DIRECTION('ref_axis',(-1.,0.,0.));
#19506=DIRECTION('center_axis',(0.,0.,1.));
#19507=DIRECTION('ref_axis',(1.,0.,0.));
#19508=DIRECTION('center_axis',(0.,0.,1.));
#19509=DIRECTION('ref_axis',(1.,0.,0.));
#19510=DIRECTION('',(0.,0.,1.));
#19511=DIRECTION('center_axis',(-0.646240799313457,0.763133559282191,0.));
#19512=DIRECTION('ref_axis',(0.,0.,1.));
#19513=DIRECTION('',(-0.763133559282191,-0.646240799313457,0.));
#19514=DIRECTION('',(0.,0.,-1.));
#19515=DIRECTION('center_axis',(-0.985581969673418,-0.169198643773126,0.));
#19516=DIRECTION('ref_axis',(0.,0.,1.));
#19517=DIRECTION('',(0.169198643773126,-0.985581969673418,0.));
#19518=DIRECTION('',(0.,0.,-1.));
#19519=DIRECTION('',(0.,0.,1.));
#19520=DIRECTION('center_axis',(0.,0.,1.));
#19521=DIRECTION('ref_axis',(-1.,0.,0.));
#19522=DIRECTION('center_axis',(0.,0.,-1.));
#19523=DIRECTION('ref_axis',(-1.,0.,0.));
#19524=DIRECTION('center_axis',(0.,0.,1.));
#19525=DIRECTION('ref_axis',(-1.,0.,0.));
#19526=DIRECTION('center_axis',(0.,0.,1.));
#19527=DIRECTION('ref_axis',(1.,0.,0.));
#19528=DIRECTION('center_axis',(0.,0.,1.));
#19529=DIRECTION('ref_axis',(1.,0.,0.));
#19530=DIRECTION('',(0.,0.,1.));
#19531=DIRECTION('center_axis',(-0.591433083115099,0.806354083636319,0.));
#19532=DIRECTION('ref_axis',(0.,0.,1.));
#19533=DIRECTION('',(-0.806354083636319,-0.591433083115099,0.));
#19534=DIRECTION('',(0.,0.,-1.));
#19535=DIRECTION('center_axis',(-0.994983842282392,-0.100035761590388,0.));
#19536=DIRECTION('ref_axis',(0.,0.,1.));
#19537=DIRECTION('',(0.100035761590388,-0.994983842282392,0.));
#19538=DIRECTION('',(0.,0.,-1.));
#19539=DIRECTION('',(0.,0.,1.));
#19540=DIRECTION('center_axis',(0.,0.,1.));
#19541=DIRECTION('ref_axis',(-1.,0.,0.));
#19542=DIRECTION('center_axis',(0.,0.,-1.));
#19543=DIRECTION('ref_axis',(-1.,0.,0.));
#19544=DIRECTION('center_axis',(0.,0.,1.));
#19545=DIRECTION('ref_axis',(-1.,0.,0.));
#19546=DIRECTION('center_axis',(0.,0.,1.));
#19547=DIRECTION('ref_axis',(1.,0.,0.));
#19548=DIRECTION('center_axis',(0.,0.,1.));
#19549=DIRECTION('ref_axis',(1.,0.,0.));
#19550=DIRECTION('',(0.,0.,1.));
#19551=DIRECTION('center_axis',(-0.533743964386147,0.845646131949623,0.));
#19552=DIRECTION('ref_axis',(0.,0.,1.));
#19553=DIRECTION('',(-0.845646131949623,-0.533743964386147,0.));
#19554=DIRECTION('',(0.,0.,-1.));
#19555=DIRECTION('center_axis',(-0.999538253627158,-0.0303855152329365,
0.));
#19556=DIRECTION('ref_axis',(0.,0.,1.));
#19557=DIRECTION('',(0.0303855152329365,-0.999538253627158,0.));
#19558=DIRECTION('',(0.,0.,-1.));
#19559=DIRECTION('',(0.,0.,1.));
#19560=DIRECTION('center_axis',(0.,0.,1.));
#19561=DIRECTION('ref_axis',(-1.,0.,0.));
#19562=DIRECTION('center_axis',(0.,0.,-1.));
#19563=DIRECTION('ref_axis',(-1.,0.,0.));
#19564=DIRECTION('center_axis',(0.,0.,1.));
#19565=DIRECTION('ref_axis',(-1.,0.,0.));
#19566=DIRECTION('center_axis',(0.,0.,1.));
#19567=DIRECTION('ref_axis',(1.,0.,0.));
#19568=DIRECTION('center_axis',(0.,0.,1.));
#19569=DIRECTION('ref_axis',(1.,0.,0.));
#19570=DIRECTION('',(0.,0.,1.));
#19571=DIRECTION('center_axis',(-0.473454498714793,0.880818277311912,0.));
#19572=DIRECTION('ref_axis',(0.,0.,1.));
#19573=DIRECTION('',(-0.880818277311912,-0.473454498714793,0.));
#19574=DIRECTION('',(0.,0.,-1.));
#19575=DIRECTION('center_axis',(-0.999223015073487,0.0394127663004103,0.));
#19576=DIRECTION('ref_axis',(0.,0.,1.));
#19577=DIRECTION('',(-0.0394127663004103,-0.999223015073487,0.));
#19578=DIRECTION('',(0.,0.,-1.));
#19579=DIRECTION('',(0.,0.,1.));
#19580=DIRECTION('center_axis',(0.,0.,1.));
#19581=DIRECTION('ref_axis',(-1.,0.,0.));
#19582=DIRECTION('center_axis',(0.,0.,-1.));
#19583=DIRECTION('ref_axis',(-1.,0.,0.));
#19584=DIRECTION('center_axis',(0.,0.,1.));
#19585=DIRECTION('ref_axis',(-1.,0.,0.));
#19586=DIRECTION('center_axis',(0.,0.,1.));
#19587=DIRECTION('ref_axis',(1.,0.,0.));
#19588=DIRECTION('center_axis',(0.,0.,1.));
#19589=DIRECTION('ref_axis',(1.,0.,0.));
#19590=DIRECTION('',(0.,0.,1.));
#19591=DIRECTION('center_axis',(-0.410858410316824,0.911699164566872,0.));
#19592=DIRECTION('ref_axis',(0.,0.,1.));
#19593=DIRECTION('',(-0.911699164566872,-0.410858410316824,0.));
#19594=DIRECTION('',(0.,0.,-1.));
#19595=DIRECTION('center_axis',(-0.994039662431944,0.109019032797885,0.));
#19596=DIRECTION('ref_axis',(0.,0.,1.));
#19597=DIRECTION('',(-0.109019032797885,-0.994039662431944,0.));
#19598=DIRECTION('',(0.,0.,-1.));
#19599=DIRECTION('',(0.,0.,1.));
#19600=DIRECTION('center_axis',(0.,0.,1.));
#19601=DIRECTION('ref_axis',(-1.,0.,0.));
#19602=DIRECTION('center_axis',(0.,0.,-1.));
#19603=DIRECTION('ref_axis',(-1.,0.,0.));
#19604=DIRECTION('center_axis',(0.,0.,1.));
#19605=DIRECTION('ref_axis',(-1.,0.,0.));
#19606=DIRECTION('center_axis',(0.,0.,1.));
#19607=DIRECTION('ref_axis',(1.,0.,0.));
#19608=DIRECTION('center_axis',(0.,0.,1.));
#19609=DIRECTION('ref_axis',(1.,0.,0.));
#19610=DIRECTION('',(0.,0.,1.));
#19611=DIRECTION('center_axis',(-0.346260661043308,0.938138345135648,0.));
#19612=DIRECTION('ref_axis',(0.,0.,1.));
#19613=DIRECTION('',(-0.938138345135648,-0.346260661043308,0.));
#19614=DIRECTION('',(0.,0.,-1.));
#19615=DIRECTION('center_axis',(-0.984013448475546,0.178094169526304,0.));
#19616=DIRECTION('ref_axis',(0.,0.,1.));
#19617=DIRECTION('',(-0.178094169526304,-0.984013448475546,0.));
#19618=DIRECTION('',(0.,0.,-1.));
#19619=DIRECTION('',(0.,0.,1.));
#19620=DIRECTION('center_axis',(0.,0.,1.));
#19621=DIRECTION('ref_axis',(-1.,0.,0.));
#19622=DIRECTION('center_axis',(0.,0.,-1.));
#19623=DIRECTION('ref_axis',(-1.,0.,0.));
#19624=DIRECTION('center_axis',(0.,0.,1.));
#19625=DIRECTION('ref_axis',(-1.,0.,0.));
#19626=DIRECTION('center_axis',(0.,0.,1.));
#19627=DIRECTION('ref_axis',(1.,0.,0.));
#19628=DIRECTION('center_axis',(0.,0.,1.));
#19629=DIRECTION('ref_axis',(1.,0.,0.));
#19630=DIRECTION('',(0.,0.,1.));
#19631=DIRECTION('center_axis',(-0.279975964635197,0.960007009988256,0.));
#19632=DIRECTION('ref_axis',(0.,0.,1.));
#19633=DIRECTION('',(-0.960007009988256,-0.279975964635197,0.));
#19634=DIRECTION('',(0.,0.,-1.));
#19635=DIRECTION('center_axis',(-0.969193219910809,0.246301649362969,0.));
#19636=DIRECTION('ref_axis',(0.,0.,1.));
#19637=DIRECTION('',(-0.246301649362969,-0.969193219910809,0.));
#19638=DIRECTION('',(0.,0.,-1.));
#19639=DIRECTION('',(0.,0.,1.));
#19640=DIRECTION('center_axis',(0.,0.,1.));
#19641=DIRECTION('ref_axis',(-1.,0.,0.));
#19642=DIRECTION('center_axis',(0.,0.,-1.));
#19643=DIRECTION('ref_axis',(-1.,0.,0.));
#19644=DIRECTION('center_axis',(0.,0.,1.));
#19645=DIRECTION('ref_axis',(-1.,0.,0.));
#19646=DIRECTION('center_axis',(0.,0.,1.));
#19647=DIRECTION('ref_axis',(1.,0.,0.));
#19648=DIRECTION('center_axis',(0.,0.,1.));
#19649=DIRECTION('ref_axis',(1.,0.,0.));
#19650=DIRECTION('',(0.,0.,1.));
#19651=DIRECTION('center_axis',(-0.212327253470465,0.977198617187769,0.));
#19652=DIRECTION('ref_axis',(0.,0.,1.));
#19653=DIRECTION('',(-0.977198617187769,-0.212327253470465,0.));
#19654=DIRECTION('',(0.,0.,-1.));
#19655=DIRECTION('center_axis',(0.,0.,-1.));
#19656=DIRECTION('ref_axis',(0.669130606358858,-0.743144825477394,0.));
#19657=DIRECTION('center_axis',(0.,0.,1.));
#19658=DIRECTION('ref_axis',(0.669130606358858,-0.743144825477394,0.));
#19659=DIRECTION('center_axis',(0.,0.,-1.));
#19660=DIRECTION('ref_axis',(0.669130606358858,-0.743144825477394,0.));
#19661=DIRECTION('center_axis',(0.,0.,1.));
#19662=DIRECTION('ref_axis',(-1.,0.,0.));
#19663=DIRECTION('center_axis',(0.,0.,1.));
#19664=DIRECTION('ref_axis',(-1.,0.,0.));
#19665=DIRECTION('center_axis',(0.,0.,-1.));
#19666=DIRECTION('ref_axis',(-1.,0.,0.));
#19667=DIRECTION('center_axis',(0.,0.,1.));
#19668=DIRECTION('ref_axis',(-1.,0.,0.));
#19669=DIRECTION('center_axis',(0.,0.,1.));
#19670=DIRECTION('ref_axis',(-1.,0.,0.));
#19671=DIRECTION('center_axis',(0.,0.,-1.));
#19672=DIRECTION('ref_axis',(-1.,0.,0.));
#19673=DIRECTION('center_axis',(0.,0.,1.));
#19674=DIRECTION('ref_axis',(-1.,0.,0.));
#19675=DIRECTION('center_axis',(0.,0.,-1.));
#19676=DIRECTION('ref_axis',(-1.,0.,0.));
#19677=DIRECTION('center_axis',(0.,0.,1.));
#19678=DIRECTION('ref_axis',(-1.,0.,0.));
#19679=DIRECTION('center_axis',(0.,0.,1.));
#19680=DIRECTION('ref_axis',(1.,0.,0.));
#19681=DIRECTION('center_axis',(0.,0.,1.));
#19682=DIRECTION('ref_axis',(-0.961261695938319,-0.275637355816999,0.));
#19683=DIRECTION('center_axis',(0.,0.,1.));
#19684=DIRECTION('ref_axis',(-1.,0.,0.));
#19685=DIRECTION('center_axis',(0.,0.,1.));
#19686=DIRECTION('ref_axis',(-0.978147600733806,-0.20791169081776,0.));
#19687=DIRECTION('center_axis',(0.,0.,1.));
#19688=DIRECTION('ref_axis',(-1.,0.,0.));
#19689=DIRECTION('center_axis',(0.,0.,1.));
#19690=DIRECTION('ref_axis',(-0.99026806874157,-0.139173100960066,0.));
#19691=DIRECTION('center_axis',(0.,0.,1.));
#19692=DIRECTION('ref_axis',(-1.,0.,0.));
#19693=DIRECTION('center_axis',(0.,0.,1.));
#19694=DIRECTION('ref_axis',(-0.997564050259824,-0.0697564737441253,0.));
#19695=DIRECTION('center_axis',(0.,0.,1.));
#19696=DIRECTION('ref_axis',(-1.,0.,0.));
#19697=DIRECTION('center_axis',(0.,0.,1.));
#19698=DIRECTION('ref_axis',(-1.,1.22464679914735E-16,0.));
#19699=DIRECTION('center_axis',(0.,0.,1.));
#19700=DIRECTION('ref_axis',(-1.,0.,0.));
#19701=DIRECTION('center_axis',(0.,0.,1.));
#19702=DIRECTION('ref_axis',(-0.997564050259824,0.0697564737441255,0.));
#19703=DIRECTION('center_axis',(0.,0.,1.));
#19704=DIRECTION('ref_axis',(-1.,0.,0.));
#19705=DIRECTION('center_axis',(0.,0.,1.));
#19706=DIRECTION('ref_axis',(-0.978147600733806,0.207911690817759,0.));
#19707=DIRECTION('center_axis',(0.,0.,-1.));
#19708=DIRECTION('ref_axis',(0.961261695938319,-0.275637355816999,0.));
#19709=DIRECTION('center_axis',(0.,0.,-1.));
#19710=DIRECTION('ref_axis',(0.939692620785908,-0.342020143325669,0.));
#19711=DIRECTION('center_axis',(0.,0.,-1.));
#19712=DIRECTION('ref_axis',(0.913545457642601,-0.4067366430758,0.));
#19713=DIRECTION('center_axis',(0.,0.,-1.));
#19714=DIRECTION('ref_axis',(0.882947592858927,-0.469471562785891,0.));
#19715=DIRECTION('center_axis',(0.,0.,-1.));
#19716=DIRECTION('ref_axis',(0.848048096156426,-0.529919264233205,0.));
#19717=DIRECTION('center_axis',(0.,0.,-1.));
#19718=DIRECTION('ref_axis',(0.809016994374947,-0.587785252292473,0.));
#19719=DIRECTION('center_axis',(0.,0.,-1.));
#19720=DIRECTION('ref_axis',(0.766044443118978,-0.642787609686539,0.));
#19721=DIRECTION('center_axis',(0.,0.,-1.));
#19722=DIRECTION('ref_axis',(0.719339800338651,-0.694658370458997,0.));
#19723=DIRECTION('center_axis',(0.,0.,1.));
#19724=DIRECTION('ref_axis',(-1.,0.,0.));
#19725=DIRECTION('center_axis',(0.,0.,-1.));
#19726=DIRECTION('ref_axis',(0.615661475325658,-0.788010753606722,0.));
#19727=DIRECTION('center_axis',(0.,0.,1.));
#19728=DIRECTION('ref_axis',(-1.,0.,0.));
#19729=DIRECTION('center_axis',(0.,0.,-1.));
#19730=DIRECTION('ref_axis',(0.559192903470747,-0.829037572555042,0.));
#19731=DIRECTION('center_axis',(0.,0.,1.));
#19732=DIRECTION('ref_axis',(-1.,0.,0.));
#19733=DIRECTION('center_axis',(0.,0.,-1.));
#19734=DIRECTION('ref_axis',(0.5,-0.866025403784439,0.));
#19735=DIRECTION('center_axis',(0.,0.,1.));
#19736=DIRECTION('ref_axis',(-1.,0.,0.));
#19737=DIRECTION('center_axis',(0.,0.,-1.));
#19738=DIRECTION('ref_axis',(0.438371146789078,-0.898794046299167,0.));
#19739=DIRECTION('center_axis',(0.,0.,1.));
#19740=DIRECTION('ref_axis',(-1.,0.,0.));
#19741=DIRECTION('center_axis',(0.,0.,-1.));
#19742=DIRECTION('ref_axis',(0.374606593415912,-0.927183854566787,0.));
#19743=DIRECTION('center_axis',(0.,0.,1.));
#19744=DIRECTION('ref_axis',(-1.,0.,0.));
#19745=DIRECTION('center_axis',(0.,0.,-1.));
#19746=DIRECTION('ref_axis',(0.309016994374947,-0.951056516295154,0.));
#19747=DIRECTION('center_axis',(0.,0.,1.));
#19748=DIRECTION('ref_axis',(-1.,0.,0.));
#19749=DIRECTION('center_axis',(0.,0.,-1.));
#19750=DIRECTION('ref_axis',(0.241921895599668,-0.970295726275997,0.));
#19751=DIRECTION('center_axis',(0.,0.,1.));
#19752=DIRECTION('ref_axis',(-1.,0.,0.));
#19753=DIRECTION('center_axis',(0.,0.,-1.));
#19754=DIRECTION('ref_axis',(0.17364817766693,-0.984807753012208,0.));
#19755=DIRECTION('center_axis',(0.,0.,1.));
#19756=DIRECTION('ref_axis',(-1.,0.,0.));
#19757=DIRECTION('center_axis',(0.,0.,-1.));
#19758=DIRECTION('ref_axis',(0.104528463267654,-0.994521895368273,0.));
#19759=DIRECTION('center_axis',(0.,0.,1.));
#19760=DIRECTION('ref_axis',(-0.034899496702501,0.999390827019096,0.));
#19761=DIRECTION('center_axis',(0.,0.,1.));
#19762=DIRECTION('ref_axis',(1.,0.,0.));
#19763=DIRECTION('center_axis',(0.,0.,1.));
#19764=DIRECTION('ref_axis',(0.0348994967025011,0.999390827019096,0.));
#19765=DIRECTION('center_axis',(0.,0.,1.));
#19766=DIRECTION('ref_axis',(1.,0.,0.));
#19767=DIRECTION('center_axis',(0.,0.,-1.));
#19768=DIRECTION('ref_axis',(-0.104528463267653,-0.994521895368273,0.));
#19769=DIRECTION('center_axis',(0.,0.,1.));
#19770=DIRECTION('ref_axis',(1.,0.,0.));
#19771=DIRECTION('center_axis',(0.,0.,-1.));
#19772=DIRECTION('ref_axis',(-0.17364817766693,-0.984807753012208,0.));
#19773=DIRECTION('center_axis',(0.,0.,1.));
#19774=DIRECTION('ref_axis',(1.,0.,0.));
#19775=DIRECTION('center_axis',(0.,0.,-1.));
#19776=DIRECTION('ref_axis',(-0.241921895599668,-0.970295726275997,0.));
#19777=DIRECTION('center_axis',(0.,0.,1.));
#19778=DIRECTION('ref_axis',(1.,0.,0.));
#19779=DIRECTION('center_axis',(0.,0.,-1.));
#19780=DIRECTION('ref_axis',(-0.309016994374947,-0.951056516295154,0.));
#19781=DIRECTION('center_axis',(0.,0.,1.));
#19782=DIRECTION('ref_axis',(1.,0.,0.));
#19783=DIRECTION('center_axis',(0.,0.,-1.));
#19784=DIRECTION('ref_axis',(-0.374606593415912,-0.927183854566787,0.));
#19785=DIRECTION('center_axis',(0.,0.,1.));
#19786=DIRECTION('ref_axis',(1.,0.,0.));
#19787=DIRECTION('center_axis',(0.,0.,-1.));
#19788=DIRECTION('ref_axis',(-0.438371146789078,-0.898794046299167,0.));
#19789=DIRECTION('center_axis',(0.,0.,1.));
#19790=DIRECTION('ref_axis',(1.,0.,0.));
#19791=DIRECTION('center_axis',(0.,0.,-1.));
#19792=DIRECTION('ref_axis',(-0.5,-0.866025403784439,0.));
#19793=DIRECTION('center_axis',(0.,0.,1.));
#19794=DIRECTION('ref_axis',(1.,0.,0.));
#19795=DIRECTION('center_axis',(0.,0.,-1.));
#19796=DIRECTION('ref_axis',(-0.559192903470747,-0.829037572555042,0.));
#19797=DIRECTION('center_axis',(0.,0.,1.));
#19798=DIRECTION('ref_axis',(1.,0.,0.));
#19799=DIRECTION('center_axis',(0.,0.,1.));
#19800=DIRECTION('ref_axis',(0.615661475325658,0.788010753606722,0.));
#19801=DIRECTION('center_axis',(0.,0.,1.));
#19802=DIRECTION('ref_axis',(1.,0.,0.));
#19803=DIRECTION('center_axis',(0.,0.,-1.));
#19804=DIRECTION('ref_axis',(-0.669130606358858,-0.743144825477394,0.));
#19805=DIRECTION('center_axis',(0.,0.,1.));
#19806=DIRECTION('ref_axis',(1.,0.,0.));
#19807=DIRECTION('center_axis',(0.,0.,1.));
#19808=DIRECTION('ref_axis',(0.719339800338651,0.694658370458997,0.));
#19809=DIRECTION('center_axis',(0.,0.,1.));
#19810=DIRECTION('ref_axis',(1.,0.,0.));
#19811=DIRECTION('center_axis',(0.,0.,-1.));
#19812=DIRECTION('ref_axis',(-0.766044443118978,-0.642787609686539,0.));
#19813=DIRECTION('center_axis',(0.,0.,1.));
#19814=DIRECTION('ref_axis',(1.,0.,0.));
#19815=DIRECTION('center_axis',(0.,0.,-1.));
#19816=DIRECTION('ref_axis',(-0.809016994374947,-0.587785252292473,0.));
#19817=DIRECTION('center_axis',(0.,0.,1.));
#19818=DIRECTION('ref_axis',(1.,0.,0.));
#19819=DIRECTION('center_axis',(0.,0.,-1.));
#19820=DIRECTION('ref_axis',(-0.848048096156426,-0.529919264233205,0.));
#19821=DIRECTION('center_axis',(0.,0.,1.));
#19822=DIRECTION('ref_axis',(1.,0.,0.));
#19823=DIRECTION('center_axis',(0.,0.,-1.));
#19824=DIRECTION('ref_axis',(-0.882947592858927,-0.469471562785891,0.));
#19825=DIRECTION('center_axis',(0.,0.,1.));
#19826=DIRECTION('ref_axis',(1.,0.,0.));
#19827=DIRECTION('center_axis',(0.,0.,-1.));
#19828=DIRECTION('ref_axis',(-0.913545457642601,-0.4067366430758,0.));
#19829=DIRECTION('center_axis',(0.,0.,1.));
#19830=DIRECTION('ref_axis',(1.,0.,0.));
#19831=DIRECTION('center_axis',(0.,0.,-1.));
#19832=DIRECTION('ref_axis',(-0.939692620785908,-0.342020143325669,0.));
#19833=DIRECTION('center_axis',(0.,0.,1.));
#19834=DIRECTION('ref_axis',(1.,0.,0.));
#19835=DIRECTION('center_axis',(0.,0.,-1.));
#19836=DIRECTION('ref_axis',(-0.961261695938319,-0.275637355816999,0.));
#19837=DIRECTION('center_axis',(0.,0.,1.));
#19838=DIRECTION('ref_axis',(1.,0.,0.));
#19839=DIRECTION('center_axis',(0.,0.,1.));
#19840=DIRECTION('ref_axis',(0.978147600733806,0.207911690817759,0.));
#19841=DIRECTION('center_axis',(0.,0.,1.));
#19842=DIRECTION('ref_axis',(1.,0.,0.));
#19843=DIRECTION('center_axis',(0.,0.,-1.));
#19844=DIRECTION('ref_axis',(-0.99026806874157,-0.139173100960065,0.));
#19845=DIRECTION('center_axis',(0.,0.,1.));
#19846=DIRECTION('ref_axis',(1.,0.,0.));
#19847=DIRECTION('center_axis',(0.,0.,-1.));
#19848=DIRECTION('ref_axis',(-0.997564050259824,-0.0697564737441253,0.));
#19849=DIRECTION('center_axis',(0.,0.,1.));
#19850=DIRECTION('ref_axis',(1.,0.,0.));
#19851=DIRECTION('center_axis',(0.,0.,1.));
#19852=DIRECTION('ref_axis',(1.,0.,0.));
#19853=DIRECTION('center_axis',(0.,0.,1.));
#19854=DIRECTION('ref_axis',(1.,0.,0.));
#19855=DIRECTION('center_axis',(0.,0.,-1.));
#19856=DIRECTION('ref_axis',(-0.997564050259824,0.0697564737441256,0.));
#19857=DIRECTION('center_axis',(0.,0.,1.));
#19858=DIRECTION('ref_axis',(1.,0.,0.));
#19859=DIRECTION('center_axis',(0.,0.,-1.));
#19860=DIRECTION('ref_axis',(-0.99026806874157,0.139173100960066,0.));
#19861=DIRECTION('center_axis',(0.,0.,1.));
#19862=DIRECTION('ref_axis',(1.,0.,0.));
#19863=DIRECTION('center_axis',(0.,0.,-1.));
#19864=DIRECTION('ref_axis',(-0.978147600733805,0.20791169081776,0.));
#19865=DIRECTION('center_axis',(0.,0.,1.));
#19866=DIRECTION('ref_axis',(1.,0.,0.));
#19867=DIRECTION('center_axis',(0.,0.,-1.));
#19868=DIRECTION('ref_axis',(-0.961261695938319,0.275637355816999,0.));
#19869=DIRECTION('center_axis',(0.,0.,1.));
#19870=DIRECTION('ref_axis',(1.,0.,0.));
#19871=DIRECTION('center_axis',(0.,0.,-1.));
#19872=DIRECTION('ref_axis',(-0.939692620785908,0.342020143325669,0.));
#19873=DIRECTION('center_axis',(0.,0.,1.));
#19874=DIRECTION('ref_axis',(1.,0.,0.));
#19875=DIRECTION('center_axis',(0.,0.,-1.));
#19876=DIRECTION('ref_axis',(-0.913545457642601,0.4067366430758,0.));
#19877=DIRECTION('center_axis',(0.,0.,1.));
#19878=DIRECTION('ref_axis',(1.,0.,0.));
#19879=DIRECTION('center_axis',(0.,0.,1.));
#19880=DIRECTION('ref_axis',(0.882947592858927,-0.469471562785891,0.));
#19881=DIRECTION('center_axis',(0.,0.,1.));
#19882=DIRECTION('ref_axis',(1.,0.,0.));
#19883=DIRECTION('center_axis',(0.,0.,-1.));
#19884=DIRECTION('ref_axis',(-0.848048096156426,0.529919264233205,0.));
#19885=DIRECTION('center_axis',(0.,0.,1.));
#19886=DIRECTION('ref_axis',(1.,0.,0.));
#19887=DIRECTION('center_axis',(0.,0.,-1.));
#19888=DIRECTION('ref_axis',(-0.809016994374947,0.587785252292473,0.));
#19889=DIRECTION('center_axis',(0.,0.,1.));
#19890=DIRECTION('ref_axis',(1.,0.,0.));
#19891=DIRECTION('center_axis',(0.,0.,-1.));
#19892=DIRECTION('ref_axis',(-0.766044443118978,0.64278760968654,0.));
#19893=DIRECTION('center_axis',(0.,0.,1.));
#19894=DIRECTION('ref_axis',(1.,0.,0.));
#19895=DIRECTION('center_axis',(0.,0.,1.));
#19896=DIRECTION('ref_axis',(0.719339800338651,-0.694658370458998,0.));
#19897=DIRECTION('center_axis',(0.,0.,1.));
#19898=DIRECTION('ref_axis',(1.,0.,0.));
#19899=DIRECTION('center_axis',(0.,0.,-1.));
#19900=DIRECTION('ref_axis',(-0.669130606358858,0.743144825477395,0.));
#19901=DIRECTION('center_axis',(0.,0.,1.));
#19902=DIRECTION('ref_axis',(1.,0.,0.));
#19903=DIRECTION('center_axis',(0.,0.,-1.));
#19904=DIRECTION('ref_axis',(-0.615661475325659,0.788010753606722,0.));
#19905=DIRECTION('center_axis',(0.,0.,1.));
#19906=DIRECTION('ref_axis',(1.,0.,0.));
#19907=DIRECTION('center_axis',(0.,0.,-1.));
#19908=DIRECTION('ref_axis',(-0.559192903470747,0.829037572555042,0.));
#19909=DIRECTION('center_axis',(0.,0.,1.));
#19910=DIRECTION('ref_axis',(1.,0.,0.));
#19911=DIRECTION('center_axis',(0.,0.,-1.));
#19912=DIRECTION('ref_axis',(-0.5,0.866025403784439,0.));
#19913=DIRECTION('center_axis',(0.,0.,1.));
#19914=DIRECTION('ref_axis',(1.,0.,0.));
#19915=DIRECTION('center_axis',(0.,0.,-1.));
#19916=DIRECTION('ref_axis',(-0.438371146789077,0.898794046299167,0.));
#19917=DIRECTION('center_axis',(0.,0.,1.));
#19918=DIRECTION('ref_axis',(1.,0.,0.));
#19919=DIRECTION('center_axis',(0.,0.,1.));
#19920=DIRECTION('ref_axis',(0.374606593415912,-0.927183854566787,0.));
#19921=DIRECTION('center_axis',(0.,0.,1.));
#19922=DIRECTION('ref_axis',(1.,0.,0.));
#19923=DIRECTION('center_axis',(0.,0.,-1.));
#19924=DIRECTION('ref_axis',(-0.309016994374947,0.951056516295154,0.));
#19925=DIRECTION('center_axis',(0.,0.,1.));
#19926=DIRECTION('ref_axis',(1.,0.,0.));
#19927=DIRECTION('center_axis',(0.,0.,-1.));
#19928=DIRECTION('ref_axis',(-0.241921895599667,0.970295726275997,0.));
#19929=DIRECTION('center_axis',(0.,0.,1.));
#19930=DIRECTION('ref_axis',(1.,0.,0.));
#19931=DIRECTION('center_axis',(0.,0.,-1.));
#19932=DIRECTION('ref_axis',(-0.17364817766693,0.984807753012208,0.));
#19933=DIRECTION('center_axis',(0.,0.,1.));
#19934=DIRECTION('ref_axis',(1.,0.,0.));
#19935=DIRECTION('center_axis',(0.,0.,-1.));
#19936=DIRECTION('ref_axis',(-0.104528463267653,0.994521895368273,0.));
#19937=DIRECTION('center_axis',(0.,0.,1.));
#19938=DIRECTION('ref_axis',(1.,0.,0.));
#19939=DIRECTION('center_axis',(0.,0.,1.));
#19940=DIRECTION('ref_axis',(0.0348994967025013,-0.999390827019096,0.));
#19941=DIRECTION('center_axis',(0.,0.,1.));
#19942=DIRECTION('ref_axis',(1.,0.,0.));
#19943=DIRECTION('center_axis',(0.,0.,-1.));
#19944=DIRECTION('ref_axis',(0.0348994967025008,0.999390827019096,0.));
#19945=DIRECTION('center_axis',(0.,0.,1.));
#19946=DIRECTION('ref_axis',(-1.,0.,0.));
#19947=DIRECTION('center_axis',(0.,0.,-1.));
#19948=DIRECTION('ref_axis',(0.104528463267653,0.994521895368273,0.));
#19949=DIRECTION('center_axis',(0.,0.,1.));
#19950=DIRECTION('ref_axis',(-1.,0.,0.));
#19951=DIRECTION('center_axis',(0.,0.,-1.));
#19952=DIRECTION('ref_axis',(0.17364817766693,0.984807753012208,0.));
#19953=DIRECTION('center_axis',(0.,0.,1.));
#19954=DIRECTION('ref_axis',(-1.,0.,0.));
#19955=DIRECTION('center_axis',(0.,0.,-1.));
#19956=DIRECTION('ref_axis',(0.241921895599668,0.970295726275997,0.));
#19957=DIRECTION('center_axis',(0.,0.,1.));
#19958=DIRECTION('ref_axis',(-1.,0.,0.));
#19959=DIRECTION('center_axis',(0.,0.,1.));
#19960=DIRECTION('ref_axis',(-0.309016994374948,-0.951056516295154,0.));
#19961=DIRECTION('center_axis',(0.,0.,1.));
#19962=DIRECTION('ref_axis',(-1.,0.,0.));
#19963=DIRECTION('center_axis',(0.,0.,-1.));
#19964=DIRECTION('ref_axis',(0.374606593415912,0.927183854566787,0.));
#19965=DIRECTION('center_axis',(0.,0.,1.));
#19966=DIRECTION('ref_axis',(-1.,0.,0.));
#19967=DIRECTION('center_axis',(0.,0.,-1.));
#19968=DIRECTION('ref_axis',(0.438371146789078,0.898794046299167,0.));
#19969=DIRECTION('center_axis',(0.,0.,1.));
#19970=DIRECTION('ref_axis',(-1.,0.,0.));
#19971=DIRECTION('center_axis',(0.,0.,-1.));
#19972=DIRECTION('ref_axis',(0.5,0.866025403784438,0.));
#19973=DIRECTION('center_axis',(0.,0.,1.));
#19974=DIRECTION('ref_axis',(-1.,0.,0.));
#19975=DIRECTION('center_axis',(0.,0.,-1.));
#19976=DIRECTION('ref_axis',(0.559192903470747,0.829037572555042,0.));
#19977=DIRECTION('center_axis',(0.,0.,1.));
#19978=DIRECTION('ref_axis',(-1.,0.,0.));
#19979=DIRECTION('center_axis',(0.,0.,-1.));
#19980=DIRECTION('ref_axis',(0.615661475325658,0.788010753606722,0.));
#19981=DIRECTION('center_axis',(0.,0.,1.));
#19982=DIRECTION('ref_axis',(-1.,0.,0.));
#19983=DIRECTION('center_axis',(0.,0.,1.));
#19984=DIRECTION('ref_axis',(-0.669130606358858,-0.743144825477394,0.));
#19985=DIRECTION('center_axis',(0.,0.,1.));
#19986=DIRECTION('ref_axis',(-1.,0.,0.));
#19987=DIRECTION('center_axis',(0.,0.,-1.));
#19988=DIRECTION('ref_axis',(0.719339800338651,0.694658370458997,0.));
#19989=DIRECTION('center_axis',(0.,0.,1.));
#19990=DIRECTION('ref_axis',(-1.,0.,0.));
#19991=DIRECTION('center_axis',(0.,0.,-1.));
#19992=DIRECTION('ref_axis',(0.766044443118978,0.642787609686539,0.));
#19993=DIRECTION('center_axis',(0.,0.,1.));
#19994=DIRECTION('ref_axis',(-1.,0.,0.));
#19995=DIRECTION('center_axis',(0.,0.,-1.));
#19996=DIRECTION('ref_axis',(0.809016994374948,0.587785252292473,0.));
#19997=DIRECTION('center_axis',(0.,0.,1.));
#19998=DIRECTION('ref_axis',(-1.,0.,0.));
#19999=DIRECTION('center_axis',(0.,0.,-1.));
#20000=DIRECTION('ref_axis',(1.,0.,0.));
#20001=DIRECTION('center_axis',(0.,0.,1.));
#20002=DIRECTION('ref_axis',(0.96126169593832,0.275637355816994,0.));
#20003=DIRECTION('',(0.,0.,-1.));
#20004=DIRECTION('center_axis',(0.,0.,1.));
#20005=DIRECTION('ref_axis',(-0.961261695938319,-0.275637355816999,0.));
#20006=DIRECTION('',(0.,0.,1.));
#20007=DIRECTION('center_axis',(-0.971378440778616,0.237537207170802,0.));
#20008=DIRECTION('ref_axis',(0.,0.,1.));
#20009=DIRECTION('',(0.,0.,1.));
#20010=DIRECTION('',(-0.237537207170802,-0.971378440778616,0.));
#20011=DIRECTION('center_axis',(-0.969193219910856,-0.246301649362784,0.));
#20012=DIRECTION('ref_axis',(0.,0.,1.));
#20013=DIRECTION('',(0.,0.,1.));
#20014=DIRECTION('',(0.246301649362784,-0.969193219910856,0.));
#20015=DIRECTION('',(0.,0.,-1.));
#20016=DIRECTION('center_axis',(0.,0.,-1.));
#20017=DIRECTION('ref_axis',(0.719339800338651,0.694658370458997,0.));
#20018=DIRECTION('center_axis',(0.,0.,1.));
#20019=DIRECTION('ref_axis',(0.719339800338651,0.694658370458997,0.));
#20020=DIRECTION('center_axis',(0.,0.,1.));
#20021=DIRECTION('ref_axis',(0.719339800338677,0.69465837045897,0.));
#20022=DIRECTION('center_axis',(0.,0.,1.));
#20023=DIRECTION('ref_axis',(-0.719339800338651,-0.694658370458997,0.));
#20024=DIRECTION('',(0.,0.,1.));
#20025=DIRECTION('center_axis',(-0.279975964635093,-0.960007009988286,0.));
#20026=DIRECTION('ref_axis',(0.,0.,-1.));
#20027=DIRECTION('',(0.960007009988286,-0.279975964635093,0.));
#20028=DIRECTION('',(0.,0.,-1.));
#20029=DIRECTION('center_axis',(-0.984013448475508,-0.178094169526516,0.));
#20030=DIRECTION('ref_axis',(0.,0.,1.));
#20031=DIRECTION('',(0.,0.,1.));
#20032=DIRECTION('',(0.178094169526516,-0.984013448475508,0.));
#20033=DIRECTION('',(0.,0.,-1.));
#20034=DIRECTION('center_axis',(0.,0.,-1.));
#20035=DIRECTION('ref_axis',(0.766044443118978,0.642787609686539,0.));
#20036=DIRECTION('center_axis',(0.,0.,1.));
#20037=DIRECTION('ref_axis',(0.766044443118978,0.642787609686539,0.));
#20038=DIRECTION('center_axis',(0.,0.,1.));
#20039=DIRECTION('ref_axis',(0.766044443118982,0.642787609686535,0.));
#20040=DIRECTION('center_axis',(0.,0.,1.));
#20041=DIRECTION('ref_axis',(-0.766044443118978,-0.642787609686539,0.));
#20042=DIRECTION('',(0.,0.,1.));
#20043=DIRECTION('center_axis',(-0.346260661043498,-0.938138345135578,0.));
#20044=DIRECTION('ref_axis',(0.,0.,-1.));
#20045=DIRECTION('',(0.938138345135578,-0.346260661043498,0.));
#20046=DIRECTION('',(0.,0.,-1.));
#20047=DIRECTION('center_axis',(-0.994039662431923,-0.109019032798079,0.));
#20048=DIRECTION('ref_axis',(0.,0.,1.));
#20049=DIRECTION('',(0.,0.,1.));
#20050=DIRECTION('',(0.109019032798079,-0.994039662431923,0.));
#20051=DIRECTION('',(0.,0.,-1.));
#20052=DIRECTION('center_axis',(0.,0.,-1.));
#20053=DIRECTION('ref_axis',(0.809016994374947,0.587785252292473,0.));
#20054=DIRECTION('center_axis',(0.,0.,1.));
#20055=DIRECTION('ref_axis',(0.809016994374948,0.587785252292473,0.));
#20056=DIRECTION('center_axis',(0.,0.,1.));
#20057=DIRECTION('ref_axis',(0.809016994374978,0.587785252292431,0.));
#20058=DIRECTION('center_axis',(0.,0.,1.));
#20059=DIRECTION('ref_axis',(-0.809016994374948,-0.587785252292473,0.));
#20060=DIRECTION('',(0.,0.,1.));
#20061=DIRECTION('center_axis',(-0.999223015073487,-0.0394127663004103,
0.));
#20062=DIRECTION('ref_axis',(0.,0.,1.));
#20063=DIRECTION('',(0.,0.,1.));
#20064=DIRECTION('',(0.0394127663004103,-0.999223015073487,0.));
#20065=DIRECTION('center_axis',(0.,0.,1.));
#20066=DIRECTION('ref_axis',(1.,0.,0.));
#20067=DIRECTION('center_axis',(0.,0.,-1.));
#20068=DIRECTION('ref_axis',(-1.,0.,0.));
#20069=DIRECTION('',(0.,0.,-1.));
#20070=DIRECTION('center_axis',(0.,0.,1.));
#20071=DIRECTION('ref_axis',(1.,0.,0.));
#20072=DIRECTION('center_axis',(0.,0.,1.));
#20073=DIRECTION('ref_axis',(-1.,0.,0.));
#20074=DIRECTION('center_axis',(-0.410858410316832,-0.911699164566869,0.));
#20075=DIRECTION('ref_axis',(0.,0.,-1.));
#20076=DIRECTION('',(0.911699164566869,-0.410858410316832,0.));
#20077=DIRECTION('center_axis',(0.203491887231396,-0.979076632256641,0.));
#20078=DIRECTION('ref_axis',(0.,0.,-1.));
#20079=DIRECTION('',(0.979076632256641,0.203491887231396,0.));
#20080=DIRECTION('',(0.,0.,-1.));
#20081=DIRECTION('',(0.,0.,1.));
#20082=DIRECTION('center_axis',(0.,0.,1.));
#20083=DIRECTION('ref_axis',(-1.,0.,0.));
#20084=DIRECTION('center_axis',(0.,0.,-1.));
#20085=DIRECTION('ref_axis',(-1.,0.,0.));
#20086=DIRECTION('center_axis',(0.,0.,1.));
#20087=DIRECTION('ref_axis',(1.,0.,0.));
#20088=DIRECTION('center_axis',(0.,0.,1.));
#20089=DIRECTION('ref_axis',(1.,0.,0.));
#20090=DIRECTION('',(0.,0.,1.));
#20091=DIRECTION('center_axis',(-0.785222157581598,-0.61921414974377,0.));
#20092=DIRECTION('ref_axis',(0.,0.,1.));
#20093=DIRECTION('',(0.61921414974377,-0.785222157581598,0.));
#20094=DIRECTION('',(0.,0.,-1.));
#20095=DIRECTION('center_axis',(0.134699257830269,-0.990886527277455,0.));
#20096=DIRECTION('ref_axis',(0.,0.,-1.));
#20097=DIRECTION('',(0.990886527277455,0.134699257830269,0.));
#20098=DIRECTION('',(0.,0.,-1.));
#20099=DIRECTION('',(0.,0.,1.));
#20100=DIRECTION('center_axis',(0.,0.,1.));
#20101=DIRECTION('ref_axis',(-1.,0.,0.));
#20102=DIRECTION('center_axis',(0.,0.,-1.));
#20103=DIRECTION('ref_axis',(-1.,0.,0.));
#20104=DIRECTION('center_axis',(0.,0.,1.));
#20105=DIRECTION('ref_axis',(1.,0.,0.));
#20106=DIRECTION('center_axis',(0.,0.,1.));
#20107=DIRECTION('ref_axis',(1.,0.,0.));
#20108=DIRECTION('',(0.,0.,1.));
#20109=DIRECTION('center_axis',(-0.826503591449449,-0.562931446377943,0.));
#20110=DIRECTION('ref_axis',(0.,0.,1.));
#20111=DIRECTION('',(0.562931446377943,-0.826503591449449,0.));
#20112=DIRECTION('',(0.,0.,-1.));
#20113=DIRECTION('center_axis',(0.0652503871845092,-0.997868922740994,0.));
#20114=DIRECTION('ref_axis',(0.,0.,-1.));
#20115=DIRECTION('',(0.997868922740994,0.0652503871845092,0.));
#20116=DIRECTION('',(0.,0.,-1.));
#20117=DIRECTION('',(0.,0.,1.));
#20118=DIRECTION('center_axis',(0.,0.,1.));
#20119=DIRECTION('ref_axis',(-1.,0.,0.));
#20120=DIRECTION('center_axis',(0.,0.,-1.));
#20121=DIRECTION('ref_axis',(-1.,0.,0.));
#20122=DIRECTION('center_axis',(0.,0.,1.));
#20123=DIRECTION('ref_axis',(1.,0.,0.));
#20124=DIRECTION('center_axis',(0.,0.,1.));
#20125=DIRECTION('ref_axis',(1.,0.,0.));
#20126=DIRECTION('',(0.,0.,1.));
#20127=DIRECTION('center_axis',(-0.863758382899603,-0.503906197591043,0.));
#20128=DIRECTION('ref_axis',(0.,0.,1.));
#20129=DIRECTION('',(0.503906197591043,-0.863758382899603,0.));
#20130=DIRECTION('',(0.,0.,-1.));
#20131=DIRECTION('center_axis',(-0.0045163767884607,-0.999989801118344,
0.));
#20132=DIRECTION('ref_axis',(0.,0.,-1.));
#20133=DIRECTION('',(0.999989801118344,-0.0045163767884607,0.));
#20134=DIRECTION('',(0.,0.,-1.));
#20135=DIRECTION('',(0.,0.,1.));
#20136=DIRECTION('center_axis',(0.,0.,1.));
#20137=DIRECTION('ref_axis',(-1.,0.,0.));
#20138=DIRECTION('center_axis',(0.,0.,-1.));
#20139=DIRECTION('ref_axis',(-1.,0.,0.));
#20140=DIRECTION('center_axis',(0.,0.,1.));
#20141=DIRECTION('ref_axis',(1.,0.,0.));
#20142=DIRECTION('center_axis',(0.,0.,1.));
#20143=DIRECTION('ref_axis',(1.,0.,0.));
#20144=DIRECTION('',(0.,0.,1.));
#20145=DIRECTION('center_axis',(-0.896805030332968,-0.44242596846194,0.));
#20146=DIRECTION('ref_axis',(0.,0.,1.));
#20147=DIRECTION('',(0.44242596846194,-0.896805030332968,0.));
#20148=DIRECTION('',(0.,0.,-1.));
#20149=DIRECTION('center_axis',(-0.0742611374274884,-0.997238829703284,
0.));
#20150=DIRECTION('ref_axis',(0.,0.,-1.));
#20151=DIRECTION('',(0.997238829703284,-0.0742611374274884,0.));
#20152=DIRECTION('',(0.,0.,-1.));
#20153=DIRECTION('',(0.,0.,1.));
#20154=DIRECTION('center_axis',(0.,0.,1.));
#20155=DIRECTION('ref_axis',(-1.,0.,0.));
#20156=DIRECTION('center_axis',(0.,0.,-1.));
#20157=DIRECTION('ref_axis',(-1.,0.,0.));
#20158=DIRECTION('center_axis',(0.,0.,1.));
#20159=DIRECTION('ref_axis',(1.,0.,0.));
#20160=DIRECTION('center_axis',(0.,0.,1.));
#20161=DIRECTION('ref_axis',(1.,0.,0.));
#20162=DIRECTION('',(0.,0.,1.));
#20163=DIRECTION('center_axis',(-0.925482533805075,-0.378790284486995,0.));
#20164=DIRECTION('ref_axis',(0.,0.,1.));
#20165=DIRECTION('',(0.378790284486995,-0.925482533805075,0.));
#20166=DIRECTION('',(0.,0.,-1.));
#20167=DIRECTION('center_axis',(-0.143644105269881,-0.989629410952007,0.));
#20168=DIRECTION('ref_axis',(0.,0.,-1.));
#20169=DIRECTION('',(0.989629410952007,-0.143644105269881,0.));
#20170=DIRECTION('',(0.,0.,-1.));
#20171=DIRECTION('',(0.,0.,1.));
#20172=DIRECTION('center_axis',(0.,0.,1.));
#20173=DIRECTION('ref_axis',(-1.,0.,0.));
#20174=DIRECTION('center_axis',(0.,0.,-1.));
#20175=DIRECTION('ref_axis',(-1.,0.,0.));
#20176=DIRECTION('center_axis',(0.,0.,1.));
#20177=DIRECTION('ref_axis',(1.,0.,0.));
#20178=DIRECTION('center_axis',(0.,0.,1.));
#20179=DIRECTION('ref_axis',(1.,0.,0.));
#20180=DIRECTION('',(0.,0.,1.));
#20181=DIRECTION('center_axis',(-0.212327253470465,-0.977198617187769,0.));
#20182=DIRECTION('ref_axis',(0.,0.,-1.));
#20183=DIRECTION('',(0.,0.,1.));
#20184=DIRECTION('',(0.977198617187769,-0.212327253470465,0.));
#20185=DIRECTION('',(0.,0.,-1.));
#20186=DIRECTION('center_axis',(0.,0.,1.));
#20187=DIRECTION('ref_axis',(-1.,0.,0.));
#20188=DIRECTION('center_axis',(0.,0.,-1.));
#20189=DIRECTION('ref_axis',(-1.,0.,0.));
#20190=DIRECTION('center_axis',(0.,0.,1.));
#20191=DIRECTION('ref_axis',(-1.,0.,0.));
#20192=DIRECTION('center_axis',(0.,0.,-1.));
#20193=DIRECTION('ref_axis',(-1.,0.,0.));
#20194=DIRECTION('center_axis',(0.,0.,1.));
#20195=DIRECTION('ref_axis',(-1.,0.,0.));
#20196=DIRECTION('center_axis',(0.,0.,-1.));
#20197=DIRECTION('ref_axis',(-1.,0.,0.));
#20198=DIRECTION('center_axis',(0.,0.,1.));
#20199=DIRECTION('ref_axis',(1.,0.,0.));
#20200=DIRECTION('center_axis',(0.,0.,1.));
#20201=DIRECTION('ref_axis',(1.,0.,0.));
#20202=DIRECTION('center_axis',(0.,0.,1.));
#20203=DIRECTION('ref_axis',(1.,0.,0.));
#20204=DIRECTION('center_axis',(0.,0.,1.));
#20205=DIRECTION('ref_axis',(1.,0.,0.));
#20206=DIRECTION('center_axis',(0.,0.,1.));
#20207=DIRECTION('ref_axis',(1.,0.,0.));
#20208=DIRECTION('center_axis',(0.,0.,1.));
#20209=DIRECTION('ref_axis',(1.,0.,0.));
#20210=DIRECTION('center_axis',(-0.949651179401724,-0.313309172321709,0.));
#20211=DIRECTION('ref_axis',(0.,0.,1.));
#20212=DIRECTION('',(0.313309172321709,-0.949651179401724,0.));
#20213=DIRECTION('',(0.,0.,-1.));
#20214=DIRECTION('center_axis',(0.,0.,-1.));
#20215=DIRECTION('ref_axis',(0.374606593415912,0.927183854566787,0.));
#20216=DIRECTION('center_axis',(0.,0.,1.));
#20217=DIRECTION('ref_axis',(0.374606593415912,0.927183854566787,0.));
#20218=DIRECTION('center_axis',(0.,0.,-1.));
#20219=DIRECTION('ref_axis',(0.438371146789078,0.898794046299167,0.));
#20220=DIRECTION('center_axis',(0.,0.,1.));
#20221=DIRECTION('ref_axis',(0.438371146789078,0.898794046299167,0.));
#20222=DIRECTION('center_axis',(0.,0.,-1.));
#20223=DIRECTION('ref_axis',(0.5,0.866025403784438,0.));
#20224=DIRECTION('center_axis',(0.,0.,1.));
#20225=DIRECTION('ref_axis',(0.5,0.866025403784438,0.));
#20226=DIRECTION('center_axis',(0.,0.,-1.));
#20227=DIRECTION('ref_axis',(0.559192903470747,0.829037572555042,0.));
#20228=DIRECTION('center_axis',(0.,0.,1.));
#20229=DIRECTION('ref_axis',(0.559192903470747,0.829037572555042,0.));
#20230=DIRECTION('center_axis',(0.,0.,-1.));
#20231=DIRECTION('ref_axis',(0.615661475325658,0.788010753606722,0.));
#20232=DIRECTION('center_axis',(0.,0.,1.));
#20233=DIRECTION('ref_axis',(0.615661475325658,0.788010753606722,0.));
#20234=DIRECTION('center_axis',(0.,0.,1.));
#20235=DIRECTION('ref_axis',(0.66913060635886,0.743144825477393,0.));
#20236=DIRECTION('center_axis',(0.,0.,1.));
#20237=DIRECTION('ref_axis',(-0.669130606358858,-0.743144825477394,0.));
#20238=DIRECTION('center_axis',(0.,0.,1.));
#20239=DIRECTION('ref_axis',(0.615661475325709,0.788010753606683,0.));
#20240=DIRECTION('center_axis',(0.,0.,1.));
#20241=DIRECTION('ref_axis',(-0.615661475325658,-0.788010753606722,0.));
#20242=DIRECTION('center_axis',(0.,0.,1.));
#20243=DIRECTION('ref_axis',(0.559192903470803,0.829037572555004,0.));
#20244=DIRECTION('center_axis',(0.,0.,1.));
#20245=DIRECTION('ref_axis',(-0.559192903470747,-0.829037572555042,0.));
#20246=DIRECTION('center_axis',(0.,0.,1.));
#20247=DIRECTION('ref_axis',(0.5,0.866025403784439,0.));
#20248=DIRECTION('center_axis',(0.,0.,1.));
#20249=DIRECTION('ref_axis',(-0.5,-0.866025403784438,0.));
#20250=DIRECTION('center_axis',(0.,0.,1.));
#20251=DIRECTION('ref_axis',(0.438371146789079,0.898794046299166,0.));
#20252=DIRECTION('center_axis',(0.,0.,1.));
#20253=DIRECTION('ref_axis',(-0.438371146789078,-0.898794046299167,0.));
#20254=DIRECTION('center_axis',(0.,0.,1.));
#20255=DIRECTION('ref_axis',(0.374606593415967,0.927183854566765,0.));
#20256=DIRECTION('center_axis',(0.,0.,1.));
#20257=DIRECTION('ref_axis',(-0.374606593415912,-0.927183854566787,0.));
#20258=DIRECTION('center_axis',(-0.526083754912358,-0.850432762078998,0.));
#20259=DIRECTION('ref_axis',(0.,0.,1.));
#20260=DIRECTION('',(0.,0.,1.));
#20261=DIRECTION('',(0.850432762078998,-0.526083754912358,0.));
#20262=DIRECTION('',(0.,0.,-1.));
#20263=DIRECTION('center_axis',(0.,0.,-1.));
#20264=DIRECTION('ref_axis',(0.0348994967025008,0.999390827019096,0.));
#20265=DIRECTION('center_axis',(0.,0.,1.));
#20266=DIRECTION('ref_axis',(0.0348994967025008,0.999390827019096,0.));
#20267=DIRECTION('center_axis',(0.,0.,1.));
#20268=DIRECTION('ref_axis',(0.0348994967025657,0.999390827019093,0.));
#20269=DIRECTION('center_axis',(0.,0.,1.));
#20270=DIRECTION('ref_axis',(-0.0348994967025008,-0.999390827019096,0.));
#20271=DIRECTION('',(0.,0.,1.));
#20272=DIRECTION('center_axis',(0.465479050687347,-0.885058898249832,0.));
#20273=DIRECTION('ref_axis',(0.,0.,-1.));
#20274=DIRECTION('',(0.885058898249832,0.465479050687346,0.));
#20275=DIRECTION('',(0.,0.,-1.));
#20276=DIRECTION('center_axis',(0.,0.,1.));
#20277=DIRECTION('ref_axis',(-1.,0.,0.));
#20278=DIRECTION('center_axis',(0.,0.,-1.));
#20279=DIRECTION('ref_axis',(-1.,0.,0.));
#20280=DIRECTION('center_axis',(-0.584125431965383,-0.811663402976415,0.));
#20281=DIRECTION('ref_axis',(0.,0.,1.));
#20282=DIRECTION('',(0.,0.,1.));
#20283=DIRECTION('',(0.811663402976415,-0.584125431965383,0.));
#20284=DIRECTION('',(0.,0.,-1.));
#20285=DIRECTION('center_axis',(0.,0.,-1.));
#20286=DIRECTION('ref_axis',(0.104528463267653,0.994521895368273,0.));
#20287=DIRECTION('center_axis',(0.,0.,1.));
#20288=DIRECTION('ref_axis',(0.104528463267653,0.994521895368273,0.));
#20289=DIRECTION('center_axis',(0.,0.,1.));
#20290=DIRECTION('ref_axis',(0.104528463267748,0.994521895368263,0.));
#20291=DIRECTION('center_axis',(0.,0.,1.));
#20292=DIRECTION('ref_axis',(-0.104528463267653,-0.994521895368273,0.));
#20293=DIRECTION('',(0.,0.,1.));
#20294=DIRECTION('center_axis',(0.402606579317095,-0.91537311643427,0.));
#20295=DIRECTION('ref_axis',(0.,0.,-1.));
#20296=DIRECTION('',(0.91537311643427,0.402606579317095,0.));
#20297=DIRECTION('',(0.,0.,-1.));
#20298=DIRECTION('center_axis',(-0.639321308629955,-0.76893970136265,0.));
#20299=DIRECTION('ref_axis',(0.,0.,1.));
#20300=DIRECTION('',(0.,0.,1.));
#20301=DIRECTION('',(0.76893970136265,-0.639321308629955,0.));
#20302=DIRECTION('',(0.,0.,-1.));
#20303=DIRECTION('center_axis',(0.,0.,-1.));
#20304=DIRECTION('ref_axis',(0.17364817766693,0.984807753012208,0.));
#20305=DIRECTION('center_axis',(0.,0.,1.));
#20306=DIRECTION('ref_axis',(0.17364817766693,0.984807753012208,0.));
#20307=DIRECTION('center_axis',(0.,0.,1.));
#20308=DIRECTION('ref_axis',(0.173648177666931,0.984807753012208,0.));
#20309=DIRECTION('center_axis',(0.,0.,1.));
#20310=DIRECTION('ref_axis',(-0.17364817766693,-0.984807753012208,0.));
#20311=DIRECTION('',(0.,0.,1.));
#20312=DIRECTION('center_axis',(0.337772649161909,-0.941227728808574,0.));
#20313=DIRECTION('ref_axis',(0.,0.,-1.));
#20314=DIRECTION('',(0.941227728808574,0.337772649161909,0.));
#20315=DIRECTION('',(0.,0.,-1.));
#20316=DIRECTION('center_axis',(-0.691402476143223,-0.722469802817405,0.));
#20317=DIRECTION('ref_axis',(0.,0.,1.));
#20318=DIRECTION('',(0.,0.,1.));
#20319=DIRECTION('',(0.722469802817405,-0.691402476143223,0.));
#20320=DIRECTION('',(0.,0.,-1.));
#20321=DIRECTION('center_axis',(0.,0.,-1.));
#20322=DIRECTION('ref_axis',(0.241921895599668,0.970295726275996,0.));
#20323=DIRECTION('center_axis',(0.,0.,1.));
#20324=DIRECTION('ref_axis',(0.241921895599668,0.970295726275996,0.));
#20325=DIRECTION('center_axis',(0.,0.,1.));
#20326=DIRECTION('ref_axis',(0.241921895599671,0.970295726275996,0.));
#20327=DIRECTION('center_axis',(0.,0.,1.));
#20328=DIRECTION('ref_axis',(-0.241921895599668,-0.970295726275996,0.));
#20329=DIRECTION('',(0.,0.,1.));
#20330=DIRECTION('center_axis',(-0.740115200292399,-0.672480104015087,0.));
#20331=DIRECTION('ref_axis',(0.,0.,1.));
#20332=DIRECTION('',(0.,0.,1.));
#20333=DIRECTION('',(0.672480104015087,-0.740115200292399,0.));
#20334=DIRECTION('',(0.,0.,-1.));
#20335=DIRECTION('center_axis',(0.,0.,1.));
#20336=DIRECTION('ref_axis',(1.,0.,0.));
#20337=DIRECTION('center_axis',(0.,0.,-1.));
#20338=DIRECTION('ref_axis',(-1.,0.,0.));
#20339=DIRECTION('',(0.,0.,-1.));
#20340=DIRECTION('center_axis',(0.,0.,1.));
#20341=DIRECTION('ref_axis',(1.,0.,0.));
#20342=DIRECTION('center_axis',(0.,0.,1.));
#20343=DIRECTION('ref_axis',(-1.,0.,0.));
#20344=DIRECTION('center_axis',(0.271293124613069,-0.962496774299882,0.));
#20345=DIRECTION('ref_axis',(0.,0.,-1.));
#20346=DIRECTION('',(0.962496774299882,0.271293124613069,0.));
#20347=DIRECTION('center_axis',(0.785222157581596,-0.619214149743772,0.));
#20348=DIRECTION('ref_axis',(0.,0.,-1.));
#20349=DIRECTION('',(0.619214149743772,0.785222157581596,0.));
#20350=DIRECTION('',(0.,0.,-1.));
#20351=DIRECTION('',(0.,0.,1.));
#20352=DIRECTION('center_axis',(0.,0.,1.));
#20353=DIRECTION('ref_axis',(1.,0.,0.));
#20354=DIRECTION('center_axis',(0.,0.,-1.));
#20355=DIRECTION('ref_axis',(1.,0.,0.));
#20356=DIRECTION('center_axis',(0.,0.,1.));
#20357=DIRECTION('ref_axis',(1.,0.,0.));
#20358=DIRECTION('center_axis',(0.,0.,1.));
#20359=DIRECTION('ref_axis',(1.,0.,0.));
#20360=DIRECTION('',(0.,0.,1.));
#20361=DIRECTION('center_axis',(-0.203491887231601,-0.979076632256598,0.));
#20362=DIRECTION('ref_axis',(0.,0.,-1.));
#20363=DIRECTION('',(0.979076632256598,-0.203491887231601,0.));
#20364=DIRECTION('',(0.,0.,-1.));
#20365=DIRECTION('center_axis',(0.740115200292476,-0.672480104015002,0.));
#20366=DIRECTION('ref_axis',(0.,0.,-1.));
#20367=DIRECTION('',(0.672480104015002,0.740115200292476,0.));
#20368=DIRECTION('',(0.,0.,-1.));
#20369=DIRECTION('',(0.,0.,1.));
#20370=DIRECTION('center_axis',(0.,0.,1.));
#20371=DIRECTION('ref_axis',(1.,0.,0.));
#20372=DIRECTION('center_axis',(0.,0.,-1.));
#20373=DIRECTION('ref_axis',(1.,0.,0.));
#20374=DIRECTION('center_axis',(0.,0.,1.));
#20375=DIRECTION('ref_axis',(1.,0.,0.));
#20376=DIRECTION('center_axis',(0.,0.,1.));
#20377=DIRECTION('ref_axis',(1.,0.,0.));
#20378=DIRECTION('',(0.,0.,1.));
#20379=DIRECTION('center_axis',(-0.27129312461336,-0.9624967742998,0.));
#20380=DIRECTION('ref_axis',(0.,0.,-1.));
#20381=DIRECTION('',(0.9624967742998,-0.27129312461336,0.));
#20382=DIRECTION('',(0.,0.,-1.));
#20383=DIRECTION('center_axis',(0.691402476143227,-0.722469802817401,0.));
#20384=DIRECTION('ref_axis',(0.,0.,-1.));
#20385=DIRECTION('',(0.722469802817401,0.691402476143227,0.));
#20386=DIRECTION('',(0.,0.,-1.));
#20387=DIRECTION('',(0.,0.,1.));
#20388=DIRECTION('center_axis',(0.,0.,1.));
#20389=DIRECTION('ref_axis',(1.,0.,0.));
#20390=DIRECTION('center_axis',(0.,0.,-1.));
#20391=DIRECTION('ref_axis',(1.,0.,0.));
#20392=DIRECTION('center_axis',(0.,0.,1.));
#20393=DIRECTION('ref_axis',(1.,0.,0.));
#20394=DIRECTION('center_axis',(0.,0.,1.));
#20395=DIRECTION('ref_axis',(1.,0.,0.));
#20396=DIRECTION('',(0.,0.,1.));
#20397=DIRECTION('center_axis',(-0.337772649162104,-0.941227728808504,0.));
#20398=DIRECTION('ref_axis',(0.,0.,-1.));
#20399=DIRECTION('',(0.941227728808504,-0.337772649162104,0.));
#20400=DIRECTION('',(0.,0.,-1.));
#20401=DIRECTION('center_axis',(0.639321308629947,-0.768939701362657,0.));
#20402=DIRECTION('ref_axis',(0.,0.,-1.));
#20403=DIRECTION('',(0.768939701362657,0.639321308629947,0.));
#20404=DIRECTION('',(0.,0.,-1.));
#20405=DIRECTION('',(0.,0.,1.));
#20406=DIRECTION('center_axis',(0.,0.,1.));
#20407=DIRECTION('ref_axis',(1.,0.,0.));
#20408=DIRECTION('center_axis',(0.,0.,-1.));
#20409=DIRECTION('ref_axis',(1.,0.,0.));
#20410=DIRECTION('center_axis',(0.,0.,1.));
#20411=DIRECTION('ref_axis',(1.,0.,0.));
#20412=DIRECTION('center_axis',(0.,0.,1.));
#20413=DIRECTION('ref_axis',(1.,0.,0.));
#20414=DIRECTION('',(0.,0.,1.));
#20415=DIRECTION('center_axis',(-0.402606579317095,-0.91537311643427,0.));
#20416=DIRECTION('ref_axis',(0.,0.,-1.));
#20417=DIRECTION('',(0.91537311643427,-0.402606579317095,0.));
#20418=DIRECTION('',(0.,0.,-1.));
#20419=DIRECTION('center_axis',(0.584125431965637,-0.811663402976233,0.));
#20420=DIRECTION('ref_axis',(0.,0.,-1.));
#20421=DIRECTION('',(0.811663402976233,0.584125431965637,0.));
#20422=DIRECTION('',(0.,0.,-1.));
#20423=DIRECTION('',(0.,0.,1.));
#20424=DIRECTION('center_axis',(0.,0.,1.));
#20425=DIRECTION('ref_axis',(1.,0.,0.));
#20426=DIRECTION('center_axis',(0.,0.,-1.));
#20427=DIRECTION('ref_axis',(1.,0.,0.));
#20428=DIRECTION('center_axis',(0.,0.,1.));
#20429=DIRECTION('ref_axis',(1.,0.,0.));
#20430=DIRECTION('center_axis',(0.,0.,1.));
#20431=DIRECTION('ref_axis',(1.,0.,0.));
#20432=DIRECTION('',(0.,0.,1.));
#20433=DIRECTION('center_axis',(0.526083754912359,-0.850432762078998,0.));
#20434=DIRECTION('ref_axis',(0.,0.,-1.));
#20435=DIRECTION('',(0.,0.,1.));
#20436=DIRECTION('',(0.850432762078998,0.526083754912359,0.));
#20437=DIRECTION('',(0.,0.,-1.));
#20438=DIRECTION('center_axis',(0.,0.,1.));
#20439=DIRECTION('ref_axis',(1.,0.,0.));
#20440=DIRECTION('center_axis',(0.,0.,-1.));
#20441=DIRECTION('ref_axis',(1.,0.,0.));
#20442=DIRECTION('center_axis',(0.,0.,1.));
#20443=DIRECTION('ref_axis',(-1.,0.,0.));
#20444=DIRECTION('center_axis',(0.,0.,-1.));
#20445=DIRECTION('ref_axis',(-1.,0.,0.));
#20446=DIRECTION('center_axis',(0.,0.,1.));
#20447=DIRECTION('ref_axis',(-1.,0.,0.));
#20448=DIRECTION('center_axis',(0.,0.,-1.));
#20449=DIRECTION('ref_axis',(-1.,0.,0.));
#20450=DIRECTION('center_axis',(0.,0.,1.));
#20451=DIRECTION('ref_axis',(1.,0.,0.));
#20452=DIRECTION('center_axis',(0.,0.,1.));
#20453=DIRECTION('ref_axis',(1.,0.,0.));
#20454=DIRECTION('center_axis',(0.,0.,1.));
#20455=DIRECTION('ref_axis',(1.,0.,0.));
#20456=DIRECTION('center_axis',(0.,0.,1.));
#20457=DIRECTION('ref_axis',(1.,0.,0.));
#20458=DIRECTION('center_axis',(0.,0.,1.));
#20459=DIRECTION('ref_axis',(1.,0.,0.));
#20460=DIRECTION('center_axis',(0.,0.,1.));
#20461=DIRECTION('ref_axis',(1.,0.,0.));
#20462=DIRECTION('center_axis',(0.,0.,1.));
#20463=DIRECTION('ref_axis',(1.,0.,0.));
#20464=DIRECTION('center_axis',(0.,0.,1.));
#20465=DIRECTION('ref_axis',(1.,0.,0.));
#20466=DIRECTION('center_axis',(-0.465479050687165,-0.885058898249928,0.));
#20467=DIRECTION('ref_axis',(0.,0.,-1.));
#20468=DIRECTION('',(0.885058898249927,-0.465479050687165,0.));
#20469=DIRECTION('',(0.,0.,-1.));
#20470=DIRECTION('center_axis',(0.,0.,-1.));
#20471=DIRECTION('ref_axis',(-0.309016994374947,0.951056516295154,0.));
#20472=DIRECTION('center_axis',(0.,0.,1.));
#20473=DIRECTION('ref_axis',(-0.309016994374947,0.951056516295154,0.));
#20474=DIRECTION('center_axis',(0.,0.,-1.));
#20475=DIRECTION('ref_axis',(-0.241921895599667,0.970295726275997,0.));
#20476=DIRECTION('center_axis',(0.,0.,1.));
#20477=DIRECTION('ref_axis',(-0.241921895599667,0.970295726275997,0.));
#20478=DIRECTION('center_axis',(0.,0.,-1.));
#20479=DIRECTION('ref_axis',(-0.17364817766693,0.984807753012208,0.));
#20480=DIRECTION('center_axis',(0.,0.,1.));
#20481=DIRECTION('ref_axis',(-0.17364817766693,0.984807753012208,0.));
#20482=DIRECTION('center_axis',(0.,0.,-1.));
#20483=DIRECTION('ref_axis',(-0.104528463267653,0.994521895368273,0.));
#20484=DIRECTION('center_axis',(0.,0.,1.));
#20485=DIRECTION('ref_axis',(-0.104528463267653,0.994521895368273,0.));
#20486=DIRECTION('center_axis',(0.,0.,1.));
#20487=DIRECTION('ref_axis',(-0.0348994967025032,0.999390827019096,0.));
#20488=DIRECTION('center_axis',(0.,0.,1.));
#20489=DIRECTION('ref_axis',(0.0348994967025013,-0.999390827019096,0.));
#20490=DIRECTION('center_axis',(0.,0.,1.));
#20491=DIRECTION('ref_axis',(-0.104528463267655,0.994521895368273,0.));
#20492=DIRECTION('center_axis',(0.,0.,1.));
#20493=DIRECTION('ref_axis',(0.104528463267653,-0.994521895368273,0.));
#20494=DIRECTION('center_axis',(0.,0.,1.));
#20495=DIRECTION('ref_axis',(-0.173648177666993,0.984807753012197,0.));
#20496=DIRECTION('center_axis',(0.,0.,1.));
#20497=DIRECTION('ref_axis',(0.17364817766693,-0.984807753012208,0.));
#20498=DIRECTION('center_axis',(0.,0.,1.));
#20499=DIRECTION('ref_axis',(-0.241921895599764,0.970295726275972,0.));
#20500=DIRECTION('center_axis',(0.,0.,1.));
#20501=DIRECTION('ref_axis',(0.241921895599667,-0.970295726275997,0.));
#20502=DIRECTION('center_axis',(0.,0.,1.));
#20503=DIRECTION('ref_axis',(-0.309016994374908,0.951056516295166,0.));
#20504=DIRECTION('center_axis',(0.,0.,1.));
#20505=DIRECTION('ref_axis',(0.309016994374947,-0.951056516295154,0.));
#20506=DIRECTION('center_axis',(0.212327253470672,-0.977198617187725,0.));
#20507=DIRECTION('ref_axis',(0.,0.,-1.));
#20508=DIRECTION('',(0.,0.,1.));
#20509=DIRECTION('',(0.977198617187725,0.212327253470672,0.));
#20510=DIRECTION('',(0.,0.,-1.));
#20511=DIRECTION('center_axis',(0.,0.,-1.));
#20512=DIRECTION('ref_axis',(-0.669130606358858,0.743144825477395,0.));
#20513=DIRECTION('center_axis',(0.,0.,1.));
#20514=DIRECTION('ref_axis',(-0.669130606358858,0.743144825477395,0.));
#20515=DIRECTION('center_axis',(0.,0.,1.));
#20516=DIRECTION('ref_axis',(-0.669130606358858,0.743144825477394,0.));
#20517=DIRECTION('center_axis',(0.,0.,1.));
#20518=DIRECTION('ref_axis',(0.669130606358858,-0.743144825477395,0.));
#20519=DIRECTION('',(0.,0.,1.));
#20520=DIRECTION('center_axis',(0.949651179401661,-0.313309172321899,0.));
#20521=DIRECTION('ref_axis',(0.,0.,-1.));
#20522=DIRECTION('',(0.313309172321899,0.949651179401661,0.));
#20523=DIRECTION('',(0.,0.,-1.));
#20524=DIRECTION('center_axis',(0.143644105269891,-0.989629410952005,0.));
#20525=DIRECTION('ref_axis',(0.,0.,-1.));
#20526=DIRECTION('',(0.,0.,1.));
#20527=DIRECTION('',(0.989629410952005,0.143644105269891,0.));
#20528=DIRECTION('',(0.,0.,-1.));
#20529=DIRECTION('center_axis',(0.,0.,-1.));
#20530=DIRECTION('ref_axis',(-0.615661475325659,0.788010753606722,0.));
#20531=DIRECTION('center_axis',(0.,0.,1.));
#20532=DIRECTION('ref_axis',(-0.615661475325659,0.788010753606722,0.));
#20533=DIRECTION('center_axis',(0.,0.,1.));
#20534=DIRECTION('ref_axis',(-0.615661475325708,0.788010753606683,0.));
#20535=DIRECTION('center_axis',(0.,0.,1.));
#20536=DIRECTION('ref_axis',(0.615661475325659,-0.788010753606722,0.));
#20537=DIRECTION('',(0.,0.,1.));
#20538=DIRECTION('center_axis',(0.925482533805075,-0.378790284486995,0.));
#20539=DIRECTION('ref_axis',(0.,0.,-1.));
#20540=DIRECTION('',(0.378790284486995,0.925482533805075,0.));
#20541=DIRECTION('',(0.,0.,-1.));
#20542=DIRECTION('center_axis',(0.0742611374277114,-0.997238829703268,0.));
#20543=DIRECTION('ref_axis',(0.,0.,-1.));
#20544=DIRECTION('',(0.,0.,1.));
#20545=DIRECTION('',(0.997238829703268,0.0742611374277114,0.));
#20546=DIRECTION('',(0.,0.,-1.));
#20547=DIRECTION('center_axis',(0.,0.,-1.));
#20548=DIRECTION('ref_axis',(-0.559192903470747,0.829037572555042,0.));
#20549=DIRECTION('center_axis',(0.,0.,1.));
#20550=DIRECTION('ref_axis',(-0.559192903470747,0.829037572555042,0.));
#20551=DIRECTION('center_axis',(0.,0.,1.));
#20552=DIRECTION('ref_axis',(-0.559192903470747,0.829037572555042,0.));
#20553=DIRECTION('center_axis',(0.,0.,1.));
#20554=DIRECTION('ref_axis',(0.559192903470747,-0.829037572555042,0.));
#20555=DIRECTION('',(0.,0.,1.));
#20556=DIRECTION('center_axis',(0.896805030332968,-0.44242596846194,0.));
#20557=DIRECTION('ref_axis',(0.,0.,-1.));
#20558=DIRECTION('',(0.442425968461939,0.896805030332968,0.));
#20559=DIRECTION('',(0.,0.,-1.));
#20560=DIRECTION('center_axis',(0.0045163767882446,-0.999989801118345,0.));
#20561=DIRECTION('ref_axis',(0.,0.,-1.));
#20562=DIRECTION('',(0.,0.,1.));
#20563=DIRECTION('',(0.999989801118345,0.0045163767882446,0.));
#20564=DIRECTION('',(0.,0.,-1.));
#20565=DIRECTION('center_axis',(0.,0.,-1.));
#20566=DIRECTION('ref_axis',(-0.5,0.866025403784438,0.));
#20567=DIRECTION('center_axis',(0.,0.,1.));
#20568=DIRECTION('ref_axis',(-0.5,0.866025403784439,0.));
#20569=DIRECTION('center_axis',(0.,0.,1.));
#20570=DIRECTION('ref_axis',(-0.500000000000006,0.866025403784435,0.));
#20571=DIRECTION('center_axis',(0.,0.,1.));
#20572=DIRECTION('ref_axis',(0.5,-0.866025403784439,0.));
#20573=DIRECTION('',(0.,0.,1.));
#20574=DIRECTION('center_axis',(0.863758382899708,-0.503906197590862,0.));
#20575=DIRECTION('ref_axis',(0.,0.,-1.));
#20576=DIRECTION('',(0.503906197590862,0.863758382899708,0.));
#20577=DIRECTION('',(0.,0.,-1.));
#20578=DIRECTION('center_axis',(-0.0652503871847299,-0.997868922740979,
0.));
#20579=DIRECTION('ref_axis',(0.,0.,-1.));
#20580=DIRECTION('',(0.,0.,1.));
#20581=DIRECTION('',(0.997868922740979,-0.0652503871847299,0.));
#20582=DIRECTION('',(0.,0.,-1.));
#20583=DIRECTION('center_axis',(0.,0.,-1.));
#20584=DIRECTION('ref_axis',(-0.438371146789077,0.898794046299167,0.));
#20585=DIRECTION('center_axis',(0.,0.,1.));
#20586=DIRECTION('ref_axis',(-0.438371146789077,0.898794046299167,0.));
#20587=DIRECTION('center_axis',(0.,0.,1.));
#20588=DIRECTION('ref_axis',(-0.438371146789136,0.898794046299139,0.));
#20589=DIRECTION('center_axis',(0.,0.,1.));
#20590=DIRECTION('ref_axis',(0.438371146789077,-0.898794046299167,0.));
#20591=DIRECTION('',(0.,0.,1.));
#20592=DIRECTION('center_axis',(-0.134699257830059,-0.990886527277484,0.));
#20593=DIRECTION('ref_axis',(0.,0.,-1.));
#20594=DIRECTION('',(0.,0.,1.));
#20595=DIRECTION('',(0.990886527277484,-0.134699257830059,0.));
#20596=DIRECTION('',(0.,0.,-1.));
#20597=DIRECTION('center_axis',(0.,0.,1.));
#20598=DIRECTION('ref_axis',(1.,0.,0.));
#20599=DIRECTION('center_axis',(0.,0.,-1.));
#20600=DIRECTION('ref_axis',(1.,0.,0.));
#20601=DIRECTION('',(0.,0.,-1.));
#20602=DIRECTION('center_axis',(0.,0.,1.));
#20603=DIRECTION('ref_axis',(1.,0.,0.));
#20604=DIRECTION('center_axis',(0.,0.,1.));
#20605=DIRECTION('ref_axis',(1.,0.,0.));
#20606=DIRECTION('center_axis',(0.826503591449449,-0.562931446377943,0.));
#20607=DIRECTION('ref_axis',(0.,0.,-1.));
#20608=DIRECTION('',(0.562931446377943,0.826503591449449,0.));
#20609=DIRECTION('center_axis',(0.999538253627158,0.0303855152329264,0.));
#20610=DIRECTION('ref_axis',(0.,0.,-1.));
#20611=DIRECTION('',(-0.0303855152329264,0.999538253627158,0.));
#20612=DIRECTION('',(0.,0.,-1.));
#20613=DIRECTION('',(0.,0.,1.));
#20614=DIRECTION('center_axis',(0.,0.,1.));
#20615=DIRECTION('ref_axis',(1.,0.,0.));
#20616=DIRECTION('center_axis',(0.,0.,-1.));
#20617=DIRECTION('ref_axis',(1.,0.,0.));
#20618=DIRECTION('center_axis',(0.,0.,1.));
#20619=DIRECTION('ref_axis',(1.,0.,0.));
#20620=DIRECTION('center_axis',(0.,0.,1.));
#20621=DIRECTION('ref_axis',(1.,0.,0.));
#20622=DIRECTION('',(0.,0.,1.));
#20623=DIRECTION('center_axis',(0.473454498714615,-0.880818277312008,0.));
#20624=DIRECTION('ref_axis',(0.,0.,-1.));
#20625=DIRECTION('',(0.880818277312008,0.473454498714615,0.));
#20626=DIRECTION('',(0.,0.,-1.));
#20627=DIRECTION('center_axis',(0.999223015073487,-0.0394127663004103,0.));
#20628=DIRECTION('ref_axis',(0.,0.,-1.));
#20629=DIRECTION('',(0.0394127663004103,0.999223015073487,0.));
#20630=DIRECTION('',(0.,0.,-1.));
#20631=DIRECTION('',(0.,0.,1.));
#20632=DIRECTION('center_axis',(0.,0.,1.));
#20633=DIRECTION('ref_axis',(1.,0.,0.));
#20634=DIRECTION('center_axis',(0.,0.,-1.));
#20635=DIRECTION('ref_axis',(1.,0.,0.));
#20636=DIRECTION('center_axis',(0.,0.,1.));
#20637=DIRECTION('ref_axis',(1.,0.,0.));
#20638=DIRECTION('center_axis',(0.,0.,1.));
#20639=DIRECTION('ref_axis',(1.,0.,0.));
#20640=DIRECTION('',(0.,0.,1.));
#20641=DIRECTION('center_axis',(0.410858410317009,-0.911699164566789,0.));
#20642=DIRECTION('ref_axis',(0.,0.,-1.));
#20643=DIRECTION('',(0.911699164566789,0.410858410317009,0.));
#20644=DIRECTION('',(0.,0.,-1.));
#20645=DIRECTION('center_axis',(0.994039662431923,-0.10901903279808,0.));
#20646=DIRECTION('ref_axis',(0.,0.,-1.));
#20647=DIRECTION('',(0.10901903279808,0.994039662431923,0.));
#20648=DIRECTION('',(0.,0.,-1.));
#20649=DIRECTION('',(0.,0.,1.));
#20650=DIRECTION('center_axis',(0.,0.,1.));
#20651=DIRECTION('ref_axis',(1.,0.,0.));
#20652=DIRECTION('center_axis',(0.,0.,-1.));
#20653=DIRECTION('ref_axis',(1.,0.,0.));
#20654=DIRECTION('center_axis',(0.,0.,1.));
#20655=DIRECTION('ref_axis',(1.,0.,0.));
#20656=DIRECTION('center_axis',(0.,0.,1.));
#20657=DIRECTION('ref_axis',(1.,0.,0.));
#20658=DIRECTION('',(0.,0.,1.));
#20659=DIRECTION('center_axis',(0.346260661043305,-0.938138345135649,0.));
#20660=DIRECTION('ref_axis',(0.,0.,-1.));
#20661=DIRECTION('',(0.938138345135649,0.346260661043305,0.));
#20662=DIRECTION('',(0.,0.,-1.));
#20663=DIRECTION('center_axis',(0.984013448475546,-0.178094169526304,0.));
#20664=DIRECTION('ref_axis',(0.,0.,-1.));
#20665=DIRECTION('',(0.178094169526304,0.984013448475546,0.));
#20666=DIRECTION('',(0.,0.,-1.));
#20667=DIRECTION('',(0.,0.,1.));
#20668=DIRECTION('center_axis',(0.,0.,1.));
#20669=DIRECTION('ref_axis',(1.,0.,0.));
#20670=DIRECTION('center_axis',(0.,0.,-1.));
#20671=DIRECTION('ref_axis',(1.,0.,0.));
#20672=DIRECTION('center_axis',(0.,0.,1.));
#20673=DIRECTION('ref_axis',(1.,0.,0.));
#20674=DIRECTION('center_axis',(0.,0.,1.));
#20675=DIRECTION('ref_axis',(1.,0.,0.));
#20676=DIRECTION('',(0.,0.,1.));
#20677=DIRECTION('center_axis',(0.969193219910809,-0.246301649362969,0.));
#20678=DIRECTION('ref_axis',(0.,0.,-1.));
#20679=DIRECTION('',(0.,0.,1.));
#20680=DIRECTION('',(0.246301649362969,0.969193219910809,0.));
#20681=DIRECTION('',(0.,0.,-1.));
#20682=DIRECTION('center_axis',(0.,0.,1.));
#20683=DIRECTION('ref_axis',(1.,0.,0.));
#20684=DIRECTION('center_axis',(0.,0.,-1.));
#20685=DIRECTION('ref_axis',(1.,0.,0.));
#20686=DIRECTION('center_axis',(0.,0.,1.));
#20687=DIRECTION('ref_axis',(1.,0.,0.));
#20688=DIRECTION('center_axis',(0.,0.,-1.));
#20689=DIRECTION('ref_axis',(1.,0.,0.));
#20690=DIRECTION('center_axis',(0.,0.,1.));
#20691=DIRECTION('ref_axis',(1.,0.,0.));
#20692=DIRECTION('center_axis',(0.,0.,-1.));
#20693=DIRECTION('ref_axis',(1.,0.,0.));
#20694=DIRECTION('center_axis',(0.,0.,1.));
#20695=DIRECTION('ref_axis',(1.,0.,0.));
#20696=DIRECTION('center_axis',(0.,0.,-1.));
#20697=DIRECTION('ref_axis',(1.,0.,0.));
#20698=DIRECTION('center_axis',(0.,0.,1.));
#20699=DIRECTION('ref_axis',(1.,0.,0.));
#20700=DIRECTION('center_axis',(0.,0.,-1.));
#20701=DIRECTION('ref_axis',(1.,0.,0.));
#20702=DIRECTION('center_axis',(0.,0.,1.));
#20703=DIRECTION('ref_axis',(1.,0.,0.));
#20704=DIRECTION('center_axis',(0.,0.,1.));
#20705=DIRECTION('ref_axis',(1.,0.,0.));
#20706=DIRECTION('center_axis',(0.,0.,1.));
#20707=DIRECTION('ref_axis',(1.,0.,0.));
#20708=DIRECTION('center_axis',(0.,0.,1.));
#20709=DIRECTION('ref_axis',(1.,0.,0.));
#20710=DIRECTION('center_axis',(0.,0.,1.));
#20711=DIRECTION('ref_axis',(1.,0.,0.));
#20712=DIRECTION('center_axis',(0.,0.,1.));
#20713=DIRECTION('ref_axis',(1.,0.,0.));
#20714=DIRECTION('center_axis',(0.,0.,1.));
#20715=DIRECTION('ref_axis',(1.,0.,0.));
#20716=DIRECTION('center_axis',(0.,0.,1.));
#20717=DIRECTION('ref_axis',(1.,0.,0.));
#20718=DIRECTION('center_axis',(0.,0.,1.));
#20719=DIRECTION('ref_axis',(1.,0.,0.));
#20720=DIRECTION('center_axis',(0.,0.,1.));
#20721=DIRECTION('ref_axis',(1.,0.,0.));
#20722=DIRECTION('center_axis',(0.279975964635192,-0.960007009988257,0.));
#20723=DIRECTION('ref_axis',(0.,0.,-1.));
#20724=DIRECTION('',(0.960007009988257,0.279975964635192,0.));
#20725=DIRECTION('',(0.,0.,-1.));
#20726=DIRECTION('center_axis',(0.,0.,-1.));
#20727=DIRECTION('ref_axis',(-0.848048096156426,0.529919264233205,0.));
#20728=DIRECTION('center_axis',(0.,0.,1.));
#20729=DIRECTION('ref_axis',(-0.848048096156426,0.529919264233205,0.));
#20730=DIRECTION('center_axis',(0.,0.,-1.));
#20731=DIRECTION('ref_axis',(-0.809016994374947,0.587785252292473,0.));
#20732=DIRECTION('center_axis',(0.,0.,1.));
#20733=DIRECTION('ref_axis',(-0.809016994374947,0.587785252292473,0.));
#20734=DIRECTION('center_axis',(0.,0.,-1.));
#20735=DIRECTION('ref_axis',(-0.766044443118978,0.64278760968654,0.));
#20736=DIRECTION('center_axis',(0.,0.,1.));
#20737=DIRECTION('ref_axis',(-0.766044443118978,0.64278760968654,0.));
#20738=DIRECTION('center_axis',(0.,0.,1.));
#20739=DIRECTION('ref_axis',(-0.719339800338695,0.694658370458952,0.));
#20740=DIRECTION('center_axis',(0.,0.,1.));
#20741=DIRECTION('ref_axis',(0.719339800338651,-0.694658370458998,0.));
#20742=DIRECTION('center_axis',(0.,0.,1.));
#20743=DIRECTION('ref_axis',(-0.766044443118978,0.64278760968654,0.));
#20744=DIRECTION('center_axis',(0.,0.,1.));
#20745=DIRECTION('ref_axis',(0.766044443118978,-0.64278760968654,0.));
#20746=DIRECTION('center_axis',(0.,0.,1.));
#20747=DIRECTION('ref_axis',(-0.809016994374946,0.587785252292475,0.));
#20748=DIRECTION('center_axis',(0.,0.,1.));
#20749=DIRECTION('ref_axis',(0.809016994374947,-0.587785252292473,0.));
#20750=DIRECTION('center_axis',(0.,0.,1.));
#20751=DIRECTION('ref_axis',(-0.848048096156458,0.529919264233154,0.));
#20752=DIRECTION('center_axis',(0.,0.,1.));
#20753=DIRECTION('ref_axis',(0.848048096156426,-0.529919264233205,0.));
#20754=DIRECTION('center_axis',(0.831554643148335,-0.555442954279236,0.));
#20755=DIRECTION('ref_axis',(0.,0.,-1.));
#20756=DIRECTION('',(0.,0.,1.));
#20757=DIRECTION('',(0.555442954279236,0.831554643148335,0.));
#20758=DIRECTION('',(0.,0.,-1.));
#20759=DIRECTION('center_axis',(0.,0.,-1.));
#20760=DIRECTION('ref_axis',(-0.997564050259824,0.0697564737441256,0.));
#20761=DIRECTION('center_axis',(0.,0.,1.));
#20762=DIRECTION('ref_axis',(-0.997564050259824,0.0697564737441256,0.));
#20763=DIRECTION('center_axis',(0.,0.,1.));
#20764=DIRECTION('ref_axis',(-0.997564050259824,0.0697564737441253,0.));
#20765=DIRECTION('center_axis',(0.,0.,1.));
#20766=DIRECTION('ref_axis',(0.997564050259824,-0.0697564737441256,0.));
#20767=DIRECTION('',(0.,0.,1.));
#20768=DIRECTION('center_axis',(0.900764728877051,0.434307383325513,0.));
#20769=DIRECTION('ref_axis',(0.,0.,-1.));
#20770=DIRECTION('',(-0.434307383325513,0.900764728877051,0.));
#20771=DIRECTION('',(0.,0.,-1.));
#20772=DIRECTION('center_axis',(0.,0.,1.));
#20773=DIRECTION('ref_axis',(1.,0.,0.));
#20774=DIRECTION('center_axis',(0.,0.,-1.));
#20775=DIRECTION('ref_axis',(1.,0.,0.));
#20776=DIRECTION('center_axis',(0.790783275975002,-0.612096242790497,0.));
#20777=DIRECTION('ref_axis',(0.,0.,-1.));
#20778=DIRECTION('',(0.,0.,1.));
#20779=DIRECTION('',(0.612096242790497,0.790783275975002,0.));
#20780=DIRECTION('',(0.,0.,-1.));
#20781=DIRECTION('center_axis',(0.,0.,-1.));
#20782=DIRECTION('ref_axis',(-0.99026806874157,0.139173100960066,0.));
#20783=DIRECTION('center_axis',(0.,0.,1.));
#20784=DIRECTION('ref_axis',(-0.99026806874157,0.139173100960066,0.));
#20785=DIRECTION('center_axis',(0.,0.,1.));
#20786=DIRECTION('ref_axis',(-0.990268068741562,0.139173100960128,0.));
#20787=DIRECTION('center_axis',(0.,0.,1.));
#20788=DIRECTION('ref_axis',(0.99026806874157,-0.139173100960066,0.));
#20789=DIRECTION('',(0.,0.,1.));
#20790=DIRECTION('center_axis',(0.928866262851607,0.370415261208404,0.));
#20791=DIRECTION('ref_axis',(0.,0.,-1.));
#20792=DIRECTION('',(-0.370415261208404,0.928866262851607,0.));
#20793=DIRECTION('',(0.,0.,-1.));
#20794=DIRECTION('center_axis',(0.746159292170273,-0.665767459934741,0.));
#20795=DIRECTION('ref_axis',(0.,0.,-1.));
#20796=DIRECTION('',(0.,0.,1.));
#20797=DIRECTION('',(0.665767459934741,0.746159292170273,0.));
#20798=DIRECTION('',(0.,0.,-1.));
#20799=DIRECTION('center_axis',(0.,0.,-1.));
#20800=DIRECTION('ref_axis',(-0.978147600733806,0.20791169081776,0.));
#20801=DIRECTION('center_axis',(0.,0.,1.));
#20802=DIRECTION('ref_axis',(-0.978147600733806,0.20791169081776,0.));
#20803=DIRECTION('center_axis',(0.,0.,1.));
#20804=DIRECTION('ref_axis',(-0.978147600733805,0.207911690817762,0.));
#20805=DIRECTION('center_axis',(0.,0.,1.));
#20806=DIRECTION('ref_axis',(0.978147600733806,-0.20791169081776,0.));
#20807=DIRECTION('',(0.,0.,1.));
#20808=DIRECTION('center_axis',(0.952442453762932,0.304718513172479,0.));
#20809=DIRECTION('ref_axis',(0.,0.,-1.));
#20810=DIRECTION('',(-0.304718513172479,0.952442453762931,0.));
#20811=DIRECTION('',(0.,0.,-1.));
#20812=DIRECTION('center_axis',(0.697900095297528,-0.716195124937124,0.));
#20813=DIRECTION('ref_axis',(0.,0.,-1.));
#20814=DIRECTION('',(0.,0.,1.));
#20815=DIRECTION('',(0.716195124937124,0.697900095297528,0.));
#20816=DIRECTION('',(0.,0.,-1.));
#20817=DIRECTION('center_axis',(0.,0.,-1.));
#20818=DIRECTION('ref_axis',(-0.961261695938319,0.275637355816999,0.));
#20819=DIRECTION('center_axis',(0.,0.,1.));
#20820=DIRECTION('ref_axis',(-0.961261695938319,0.275637355816999,0.));
#20821=DIRECTION('center_axis',(0.,0.,1.));
#20822=DIRECTION('ref_axis',(-0.961261695938347,0.2756373558169,0.));
#20823=DIRECTION('center_axis',(0.,0.,1.));
#20824=DIRECTION('ref_axis',(0.961261695938319,-0.275637355816999,0.));
#20825=DIRECTION('',(0.,0.,1.));
#20826=DIRECTION('center_axis',(0.971378440778617,0.237537207170797,0.));
#20827=DIRECTION('ref_axis',(0.,0.,-1.));
#20828=DIRECTION('',(-0.237537207170797,0.971378440778617,0.));
#20829=DIRECTION('',(0.,0.,-1.));
#20830=DIRECTION('center_axis',(0.646240799313603,-0.763133559282066,0.));
#20831=DIRECTION('ref_axis',(0.,0.,-1.));
#20832=DIRECTION('',(0.,0.,1.));
#20833=DIRECTION('',(0.763133559282066,0.646240799313603,0.));
#20834=DIRECTION('',(0.,0.,-1.));
#20835=DIRECTION('center_axis',(0.,0.,-1.));
#20836=DIRECTION('ref_axis',(-0.939692620785908,0.342020143325669,0.));
#20837=DIRECTION('center_axis',(0.,0.,1.));
#20838=DIRECTION('ref_axis',(-0.939692620785908,0.342020143325669,0.));
#20839=DIRECTION('center_axis',(0.,0.,1.));
#20840=DIRECTION('ref_axis',(-0.939692620785885,0.342020143325732,0.));
#20841=DIRECTION('center_axis',(0.,0.,1.));
#20842=DIRECTION('ref_axis',(0.939692620785908,-0.342020143325669,0.));
#20843=DIRECTION('',(0.,0.,1.));
#20844=DIRECTION('center_axis',(0.985581969673418,0.169198643773125,0.));
#20845=DIRECTION('ref_axis',(0.,0.,-1.));
#20846=DIRECTION('',(-0.169198643773125,0.985581969673418,0.));
#20847=DIRECTION('',(0.,0.,-1.));
#20848=DIRECTION('center_axis',(0.591433083115112,-0.80635408363631,0.));
#20849=DIRECTION('ref_axis',(0.,0.,-1.));
#20850=DIRECTION('',(0.,0.,1.));
#20851=DIRECTION('',(0.80635408363631,0.591433083115112,0.));
#20852=DIRECTION('',(0.,0.,-1.));
#20853=DIRECTION('center_axis',(0.,0.,-1.));
#20854=DIRECTION('ref_axis',(-0.913545457642601,0.4067366430758,0.));
#20855=DIRECTION('center_axis',(0.,0.,1.));
#20856=DIRECTION('ref_axis',(-0.913545457642601,0.4067366430758,0.));
#20857=DIRECTION('center_axis',(0.,0.,1.));
#20858=DIRECTION('ref_axis',(-0.913545457642558,0.406736643075896,0.));
#20859=DIRECTION('center_axis',(0.,0.,1.));
#20860=DIRECTION('ref_axis',(0.913545457642601,-0.4067366430758,0.));
#20861=DIRECTION('',(0.,0.,1.));
#20862=DIRECTION('center_axis',(0.533743964386317,-0.845646131949516,0.));
#20863=DIRECTION('ref_axis',(0.,0.,-1.));
#20864=DIRECTION('',(0.,0.,1.));
#20865=DIRECTION('',(0.845646131949516,0.533743964386317,0.));
#20866=DIRECTION('',(0.,0.,-1.));
#20867=DIRECTION('center_axis',(0.,0.,1.));
#20868=DIRECTION('ref_axis',(1.,0.,0.));
#20869=DIRECTION('center_axis',(0.,0.,-1.));
#20870=DIRECTION('ref_axis',(1.,0.,0.));
#20871=DIRECTION('',(0.,0.,-1.));
#20872=DIRECTION('center_axis',(0.,0.,1.));
#20873=DIRECTION('ref_axis',(1.,0.,0.));
#20874=DIRECTION('center_axis',(0.,0.,1.));
#20875=DIRECTION('ref_axis',(1.,0.,0.));
#20876=DIRECTION('center_axis',(0.994983842282363,0.100035761590676,0.));
#20877=DIRECTION('ref_axis',(0.,0.,-1.));
#20878=DIRECTION('',(-0.100035761590676,0.994983842282363,0.));
#20879=DIRECTION('center_axis',(0.746159292170123,0.66576745993491,0.));
#20880=DIRECTION('ref_axis',(0.,0.,-1.));
#20881=DIRECTION('',(-0.66576745993491,0.746159292170123,0.));
#20882=DIRECTION('',(0.,0.,-1.));
#20883=DIRECTION('',(0.,0.,1.));
#20884=DIRECTION('center_axis',(0.,0.,1.));
#20885=DIRECTION('ref_axis',(1.,0.,0.));
#20886=DIRECTION('center_axis',(0.,0.,-1.));
#20887=DIRECTION('ref_axis',(1.,0.,0.));
#20888=DIRECTION('center_axis',(0.,0.,1.));
#20889=DIRECTION('ref_axis',(1.,0.,0.));
#20890=DIRECTION('center_axis',(0.,0.,1.));
#20891=DIRECTION('ref_axis',(1.,0.,0.));
#20892=DIRECTION('',(0.,0.,1.));
#20893=DIRECTION('center_axis',(0.92886626285169,-0.370415261208196,0.));
#20894=DIRECTION('ref_axis',(0.,0.,-1.));
#20895=DIRECTION('',(0.370415261208196,0.928866262851689,0.));
#20896=DIRECTION('',(0.,0.,-1.));
#20897=DIRECTION('center_axis',(0.790783275974884,0.61209624279065,0.));
#20898=DIRECTION('ref_axis',(0.,0.,-1.));
#20899=DIRECTION('',(-0.61209624279065,0.790783275974884,0.));
#20900=DIRECTION('',(0.,0.,-1.));
#20901=DIRECTION('',(0.,0.,1.));
#20902=DIRECTION('center_axis',(0.,0.,1.));
#20903=DIRECTION('ref_axis',(1.,0.,0.));
#20904=DIRECTION('center_axis',(0.,0.,-1.));
#20905=DIRECTION('ref_axis',(1.,0.,0.));
#20906=DIRECTION('center_axis',(0.,0.,1.));
#20907=DIRECTION('ref_axis',(1.,0.,0.));
#20908=DIRECTION('center_axis',(0.,0.,1.));
#20909=DIRECTION('ref_axis',(1.,0.,0.));
#20910=DIRECTION('',(0.,0.,1.));
#20911=DIRECTION('center_axis',(0.900764728877053,-0.434307383325507,0.));
#20912=DIRECTION('ref_axis',(0.,0.,-1.));
#20913=DIRECTION('',(0.434307383325507,0.900764728877053,0.));
#20914=DIRECTION('',(0.,0.,-1.));
#20915=DIRECTION('center_axis',(0.831554643148452,0.555442954279061,0.));
#20916=DIRECTION('ref_axis',(0.,0.,-1.));
#20917=DIRECTION('',(-0.555442954279061,0.831554643148452,0.));
#20918=DIRECTION('',(0.,0.,-1.));
#20919=DIRECTION('',(0.,0.,1.));
#20920=DIRECTION('center_axis',(0.,0.,1.));
#20921=DIRECTION('ref_axis',(1.,0.,0.));
#20922=DIRECTION('center_axis',(0.,0.,-1.));
#20923=DIRECTION('ref_axis',(1.,0.,0.));
#20924=DIRECTION('center_axis',(0.,0.,1.));
#20925=DIRECTION('ref_axis',(1.,0.,0.));
#20926=DIRECTION('center_axis',(0.,0.,1.));
#20927=DIRECTION('ref_axis',(1.,0.,0.));
#20928=DIRECTION('',(0.,0.,1.));
#20929=DIRECTION('center_axis',(0.868274759687958,0.496083603527489,0.));
#20930=DIRECTION('ref_axis',(0.,0.,-1.));
#20931=DIRECTION('',(0.,0.,1.));
#20932=DIRECTION('',(-0.496083603527489,0.868274759687958,0.));
#20933=DIRECTION('',(0.,0.,-1.));
#20934=DIRECTION('center_axis',(0.,0.,1.));
#20935=DIRECTION('ref_axis',(1.,0.,0.));
#20936=DIRECTION('center_axis',(0.,0.,-1.));
#20937=DIRECTION('ref_axis',(1.,0.,0.));
#20938=DIRECTION('center_axis',(0.,0.,1.));
#20939=DIRECTION('ref_axis',(1.,0.,0.));
#20940=DIRECTION('center_axis',(0.,0.,-1.));
#20941=DIRECTION('ref_axis',(1.,0.,0.));
#20942=DIRECTION('center_axis',(0.,0.,1.));
#20943=DIRECTION('ref_axis',(1.,0.,0.));
#20944=DIRECTION('center_axis',(0.,0.,-1.));
#20945=DIRECTION('ref_axis',(1.,0.,0.));
#20946=DIRECTION('center_axis',(0.,0.,1.));
#20947=DIRECTION('ref_axis',(1.,0.,0.));
#20948=DIRECTION('center_axis',(0.,0.,-1.));
#20949=DIRECTION('ref_axis',(1.,0.,0.));
#20950=DIRECTION('center_axis',(0.,0.,1.));
#20951=DIRECTION('ref_axis',(1.,0.,0.));
#20952=DIRECTION('center_axis',(0.,0.,-1.));
#20953=DIRECTION('ref_axis',(1.,0.,0.));
#20954=DIRECTION('center_axis',(0.,0.,1.));
#20955=DIRECTION('ref_axis',(1.,0.,0.));
#20956=DIRECTION('center_axis',(0.,0.,1.));
#20957=DIRECTION('ref_axis',(1.,0.,0.));
#20958=DIRECTION('center_axis',(0.,0.,1.));
#20959=DIRECTION('ref_axis',(1.,0.,0.));
#20960=DIRECTION('center_axis',(0.,0.,1.));
#20961=DIRECTION('ref_axis',(1.,0.,0.));
#20962=DIRECTION('center_axis',(0.,0.,1.));
#20963=DIRECTION('ref_axis',(1.,0.,0.));
#20964=DIRECTION('center_axis',(0.,0.,1.));
#20965=DIRECTION('ref_axis',(1.,0.,0.));
#20966=DIRECTION('center_axis',(0.,0.,1.));
#20967=DIRECTION('ref_axis',(1.,0.,0.));
#20968=DIRECTION('center_axis',(0.,0.,1.));
#20969=DIRECTION('ref_axis',(1.,0.,0.));
#20970=DIRECTION('center_axis',(0.,0.,1.));
#20971=DIRECTION('ref_axis',(1.,0.,0.));
#20972=DIRECTION('center_axis',(0.,0.,1.));
#20973=DIRECTION('ref_axis',(1.,0.,0.));
#20974=DIRECTION('center_axis',(0.,0.,1.));
#20975=DIRECTION('ref_axis',(1.,0.,0.));
#20976=DIRECTION('center_axis',(0.,0.,1.));
#20977=DIRECTION('ref_axis',(1.,0.,0.));
#20978=DIRECTION('center_axis',(0.868274759687958,-0.496083603527489,0.));
#20979=DIRECTION('ref_axis',(0.,0.,-1.));
#20980=DIRECTION('',(0.496083603527489,0.868274759687958,0.));
#20981=DIRECTION('',(0.,0.,-1.));
#20982=DIRECTION('center_axis',(0.,0.,-1.));
#20983=DIRECTION('ref_axis',(-0.99026806874157,-0.139173100960065,0.));
#20984=DIRECTION('center_axis',(0.,0.,1.));
#20985=DIRECTION('ref_axis',(-0.99026806874157,-0.139173100960065,0.));
#20986=DIRECTION('center_axis',(0.,0.,-1.));
#20987=DIRECTION('ref_axis',(-0.997564050259824,-0.0697564737441253,0.));
#20988=DIRECTION('center_axis',(0.,0.,1.));
#20989=DIRECTION('ref_axis',(-0.997564050259824,-0.0697564737441253,0.));
#20990=DIRECTION('center_axis',(0.,0.,1.));
#20991=DIRECTION('ref_axis',(-1.,-1.22464679914735E-16,0.));
#20992=DIRECTION('center_axis',(0.,0.,1.));
#20993=DIRECTION('ref_axis',(1.,0.,0.));
#20994=DIRECTION('center_axis',(0.,0.,1.));
#20995=DIRECTION('ref_axis',(-0.99756405025982,-0.0697564737441876,0.));
#20996=DIRECTION('center_axis',(0.,0.,1.));
#20997=DIRECTION('ref_axis',(0.997564050259824,0.0697564737441253,0.));
#20998=DIRECTION('center_axis',(0.,0.,1.));
#20999=DIRECTION('ref_axis',(-0.99026806874158,-0.139173100959998,0.));
#21000=DIRECTION('center_axis',(0.,0.,1.));
#21001=DIRECTION('ref_axis',(0.99026806874157,0.139173100960065,0.));
#21002=DIRECTION('center_axis',(0.984013448475508,0.178094169526516,0.));
#21003=DIRECTION('ref_axis',(0.,0.,-1.));
#21004=DIRECTION('',(0.,0.,1.));
#21005=DIRECTION('',(-0.178094169526516,0.984013448475508,0.));
#21006=DIRECTION('',(0.,0.,-1.));
#21007=DIRECTION('center_axis',(0.,0.,-1.));
#21008=DIRECTION('ref_axis',(-0.766044443118978,-0.642787609686539,0.));
#21009=DIRECTION('center_axis',(0.,0.,1.));
#21010=DIRECTION('ref_axis',(-0.766044443118978,-0.642787609686539,0.));
#21011=DIRECTION('center_axis',(0.,0.,1.));
#21012=DIRECTION('ref_axis',(-0.766044443118982,-0.642787609686535,0.));
#21013=DIRECTION('center_axis',(0.,0.,1.));
#21014=DIRECTION('ref_axis',(0.766044443118978,0.642787609686539,0.));
#21015=DIRECTION('',(0.,0.,1.));
#21016=DIRECTION('center_axis',(0.346260661043498,0.938138345135578,0.));
#21017=DIRECTION('ref_axis',(0.,0.,1.));
#21018=DIRECTION('',(-0.938138345135578,0.346260661043498,0.));
#21019=DIRECTION('',(0.,0.,-1.));
#21020=DIRECTION('center_axis',(0.994039662431945,0.109019032797875,0.));
#21021=DIRECTION('ref_axis',(0.,0.,-1.));
#21022=DIRECTION('',(0.,0.,1.));
#21023=DIRECTION('',(-0.109019032797875,0.994039662431945,0.));
#21024=DIRECTION('',(0.,0.,-1.));
#21025=DIRECTION('center_axis',(0.,0.,-1.));
#21026=DIRECTION('ref_axis',(-0.809016994374948,-0.587785252292473,0.));
#21027=DIRECTION('center_axis',(0.,0.,1.));
#21028=DIRECTION('ref_axis',(-0.809016994374948,-0.587785252292473,0.));
#21029=DIRECTION('center_axis',(0.,0.,1.));
#21030=DIRECTION('ref_axis',(-0.809016994374945,-0.587785252292477,0.));
#21031=DIRECTION('center_axis',(0.,0.,1.));
#21032=DIRECTION('ref_axis',(0.809016994374948,0.587785252292473,0.));
#21033=DIRECTION('',(0.,0.,1.));
#21034=DIRECTION('center_axis',(0.41085841031682,0.911699164566874,0.));
#21035=DIRECTION('ref_axis',(0.,0.,1.));
#21036=DIRECTION('',(-0.911699164566874,0.41085841031682,0.));
#21037=DIRECTION('',(0.,0.,-1.));
#21038=DIRECTION('center_axis',(0.999223015073487,0.0394127663004103,0.));
#21039=DIRECTION('ref_axis',(0.,0.,-1.));
#21040=DIRECTION('',(0.,0.,1.));
#21041=DIRECTION('',(-0.0394127663004103,0.999223015073487,0.));
#21042=DIRECTION('',(0.,0.,-1.));
#21043=DIRECTION('center_axis',(0.,0.,-1.));
#21044=DIRECTION('ref_axis',(-0.848048096156426,-0.529919264233205,0.));
#21045=DIRECTION('center_axis',(0.,0.,1.));
#21046=DIRECTION('ref_axis',(-0.848048096156426,-0.529919264233205,0.));
#21047=DIRECTION('center_axis',(0.,0.,1.));
#21048=DIRECTION('ref_axis',(-0.848048096156423,-0.529919264233209,0.));
#21049=DIRECTION('center_axis',(0.,0.,1.));
#21050=DIRECTION('ref_axis',(0.848048096156426,0.529919264233205,0.));
#21051=DIRECTION('',(0.,0.,1.));
#21052=DIRECTION('center_axis',(0.473454498714793,0.880818277311912,0.));
#21053=DIRECTION('ref_axis',(0.,0.,1.));
#21054=DIRECTION('',(-0.880818277311912,0.473454498714793,0.));
#21055=DIRECTION('',(0.,0.,-1.));
#21056=DIRECTION('center_axis',(0.999538253627158,-0.0303855152329264,0.));
#21057=DIRECTION('ref_axis',(0.,0.,-1.));
#21058=DIRECTION('',(0.,0.,1.));
#21059=DIRECTION('',(0.0303855152329264,0.999538253627158,0.));
#21060=DIRECTION('',(0.,0.,-1.));
#21061=DIRECTION('center_axis',(0.,0.,-1.));
#21062=DIRECTION('ref_axis',(-0.882947592858927,-0.469471562785891,0.));
#21063=DIRECTION('center_axis',(0.,0.,1.));
#21064=DIRECTION('ref_axis',(-0.882947592858927,-0.469471562785891,0.));
#21065=DIRECTION('center_axis',(0.,0.,1.));
#21066=DIRECTION('ref_axis',(-0.882947592858927,-0.469471562785891,0.));
#21067=DIRECTION('center_axis',(0.,0.,1.));
#21068=DIRECTION('ref_axis',(0.882947592858927,0.469471562785891,0.));
#21069=DIRECTION('',(0.,0.,1.));
#21070=DIRECTION('center_axis',(0.533743964386317,0.845646131949516,0.));
#21071=DIRECTION('ref_axis',(0.,0.,-1.));
#21072=DIRECTION('',(-0.845646131949516,0.533743964386317,0.));
#21073=DIRECTION('',(0.,0.,-1.));
#21074=DIRECTION('center_axis',(0.994983842282394,-0.100035761590367,0.));
#21075=DIRECTION('ref_axis',(0.,0.,-1.));
#21076=DIRECTION('',(0.,0.,1.));
#21077=DIRECTION('',(0.100035761590367,0.994983842282394,0.));
#21078=DIRECTION('',(0.,0.,-1.));
#21079=DIRECTION('center_axis',(0.,0.,-1.));
#21080=DIRECTION('ref_axis',(-0.913545457642601,-0.4067366430758,0.));
#21081=DIRECTION('center_axis',(0.,0.,1.));
#21082=DIRECTION('ref_axis',(-0.913545457642601,-0.4067366430758,0.));
#21083=DIRECTION('center_axis',(0.,0.,1.));
#21084=DIRECTION('ref_axis',(-0.913545457642598,-0.406736643075806,0.));
#21085=DIRECTION('center_axis',(0.,0.,1.));
#21086=DIRECTION('ref_axis',(0.913545457642601,0.4067366430758,0.));
#21087=DIRECTION('',(0.,0.,1.));
#21088=DIRECTION('center_axis',(0.591433083115112,0.80635408363631,0.));
#21089=DIRECTION('ref_axis',(0.,0.,-1.));
#21090=DIRECTION('',(-0.80635408363631,0.591433083115112,0.));
#21091=DIRECTION('',(0.,0.,-1.));
#21092=DIRECTION('center_axis',(0.985581969673453,-0.169198643772926,0.));
#21093=DIRECTION('ref_axis',(0.,0.,-1.));
#21094=DIRECTION('',(0.,0.,1.));
#21095=DIRECTION('',(0.169198643772926,0.985581969673453,0.));
#21096=DIRECTION('',(0.,0.,-1.));
#21097=DIRECTION('center_axis',(0.,0.,-1.));
#21098=DIRECTION('ref_axis',(-0.939692620785908,-0.342020143325669,0.));
#21099=DIRECTION('center_axis',(0.,0.,1.));
#21100=DIRECTION('ref_axis',(-0.939692620785908,-0.342020143325669,0.));
#21101=DIRECTION('center_axis',(0.,0.,1.));
#21102=DIRECTION('ref_axis',(-0.939692620785908,-0.342020143325671,0.));
#21103=DIRECTION('center_axis',(0.,0.,1.));
#21104=DIRECTION('ref_axis',(0.939692620785908,0.342020143325669,0.));
#21105=DIRECTION('',(0.,0.,1.));
#21106=DIRECTION('center_axis',(0.646240799313611,0.76313355928206,0.));
#21107=DIRECTION('ref_axis',(0.,0.,-1.));
#21108=DIRECTION('',(-0.76313355928206,0.646240799313611,0.));
#21109=DIRECTION('',(0.,0.,-1.));
#21110=DIRECTION('center_axis',(0.971378440778567,-0.237537207171004,0.));
#21111=DIRECTION('ref_axis',(0.,0.,-1.));
#21112=DIRECTION('',(0.,0.,1.));
#21113=DIRECTION('',(0.237537207171004,0.971378440778567,0.));
#21114=DIRECTION('',(0.,0.,-1.));
#21115=DIRECTION('center_axis',(0.,0.,-1.));
#21116=DIRECTION('ref_axis',(-0.961261695938319,-0.275637355816999,0.));
#21117=DIRECTION('center_axis',(0.,0.,1.));
#21118=DIRECTION('ref_axis',(-0.961261695938319,-0.275637355816999,0.));
#21119=DIRECTION('center_axis',(0.,0.,1.));
#21120=DIRECTION('ref_axis',(-0.96126169593832,-0.275637355816994,0.));
#21121=DIRECTION('center_axis',(0.,0.,1.));
#21122=DIRECTION('ref_axis',(0.961261695938319,0.275637355816999,0.));
#21123=DIRECTION('',(0.,0.,1.));
#21124=DIRECTION('center_axis',(0.952442453762929,-0.304718513172487,0.));
#21125=DIRECTION('ref_axis',(0.,0.,-1.));
#21126=DIRECTION('',(0.,0.,1.));
#21127=DIRECTION('',(0.304718513172487,0.952442453762929,0.));
#21128=DIRECTION('',(0.,0.,-1.));
#21129=DIRECTION('center_axis',(0.,0.,1.));
#21130=DIRECTION('ref_axis',(1.,0.,0.));
#21131=DIRECTION('center_axis',(0.,0.,-1.));
#21132=DIRECTION('ref_axis',(1.,0.,0.));
#21133=DIRECTION('',(0.,0.,-1.));
#21134=DIRECTION('center_axis',(0.,0.,1.));
#21135=DIRECTION('ref_axis',(1.,0.,0.));
#21136=DIRECTION('center_axis',(0.,0.,1.));
#21137=DIRECTION('ref_axis',(1.,0.,0.));
#21138=DIRECTION('center_axis',(0.697900095297593,0.71619512493706,0.));
#21139=DIRECTION('ref_axis',(0.,0.,-1.));
#21140=DIRECTION('',(-0.71619512493706,0.697900095297593,0.));
#21141=DIRECTION('center_axis',(0.143644105269892,0.989629410952005,0.));
#21142=DIRECTION('ref_axis',(0.,0.,1.));
#21143=DIRECTION('',(-0.989629410952005,0.143644105269892,0.));
#21144=DIRECTION('',(0.,0.,-1.));
#21145=DIRECTION('',(0.,0.,1.));
#21146=DIRECTION('center_axis',(0.,0.,1.));
#21147=DIRECTION('ref_axis',(1.,0.,0.));
#21148=DIRECTION('center_axis',(0.,0.,-1.));
#21149=DIRECTION('ref_axis',(1.,0.,0.));
#21150=DIRECTION('center_axis',(0.,0.,1.));
#21151=DIRECTION('ref_axis',(1.,0.,0.));
#21152=DIRECTION('center_axis',(0.,0.,1.));
#21153=DIRECTION('ref_axis',(1.,0.,0.));
#21154=DIRECTION('',(0.,0.,1.));
#21155=DIRECTION('center_axis',(0.949651179401728,0.313309172321697,0.));
#21156=DIRECTION('ref_axis',(0.,0.,-1.));
#21157=DIRECTION('',(-0.313309172321697,0.949651179401728,0.));
#21158=DIRECTION('',(0.,0.,-1.));
#21159=DIRECTION('center_axis',(0.212327253470465,0.977198617187769,0.));
#21160=DIRECTION('ref_axis',(0.,0.,1.));
#21161=DIRECTION('',(-0.977198617187769,0.212327253470465,0.));
#21162=DIRECTION('',(0.,0.,-1.));
#21163=DIRECTION('',(0.,0.,1.));
#21164=DIRECTION('center_axis',(0.,0.,1.));
#21165=DIRECTION('ref_axis',(1.,0.,0.));
#21166=DIRECTION('center_axis',(0.,0.,-1.));
#21167=DIRECTION('ref_axis',(1.,0.,0.));
#21168=DIRECTION('center_axis',(0.,0.,1.));
#21169=DIRECTION('ref_axis',(1.,0.,0.));
#21170=DIRECTION('center_axis',(0.,0.,1.));
#21171=DIRECTION('ref_axis',(1.,0.,0.));
#21172=DIRECTION('',(0.,0.,1.));
#21173=DIRECTION('center_axis',(0.279975964635197,0.960007009988256,0.));
#21174=DIRECTION('ref_axis',(0.,0.,1.));
#21175=DIRECTION('',(0.,0.,1.));
#21176=DIRECTION('',(-0.960007009988256,0.279975964635197,0.));
#21177=DIRECTION('',(0.,0.,-1.));
#21178=DIRECTION('center_axis',(0.,0.,1.));
#21179=DIRECTION('ref_axis',(1.,0.,0.));
#21180=DIRECTION('center_axis',(0.,0.,-1.));
#21181=DIRECTION('ref_axis',(1.,0.,0.));
#21182=DIRECTION('center_axis',(0.,0.,1.));
#21183=DIRECTION('ref_axis',(1.,0.,0.));
#21184=DIRECTION('center_axis',(0.,0.,-1.));
#21185=DIRECTION('ref_axis',(1.,0.,0.));
#21186=DIRECTION('center_axis',(0.,0.,1.));
#21187=DIRECTION('ref_axis',(1.,0.,0.));
#21188=DIRECTION('center_axis',(0.,0.,-1.));
#21189=DIRECTION('ref_axis',(1.,0.,0.));
#21190=DIRECTION('center_axis',(0.,0.,1.));
#21191=DIRECTION('ref_axis',(1.,0.,0.));
#21192=DIRECTION('center_axis',(0.,0.,-1.));
#21193=DIRECTION('ref_axis',(1.,0.,0.));
#21194=DIRECTION('center_axis',(0.,0.,1.));
#21195=DIRECTION('ref_axis',(1.,0.,0.));
#21196=DIRECTION('center_axis',(0.,0.,-1.));
#21197=DIRECTION('ref_axis',(1.,0.,0.));
#21198=DIRECTION('center_axis',(0.,0.,1.));
#21199=DIRECTION('ref_axis',(1.,0.,0.));
#21200=DIRECTION('center_axis',(0.,0.,-1.));
#21201=DIRECTION('ref_axis',(1.,0.,0.));
#21202=DIRECTION('center_axis',(0.,0.,1.));
#21203=DIRECTION('ref_axis',(1.,0.,0.));
#21204=DIRECTION('center_axis',(0.,0.,-1.));
#21205=DIRECTION('ref_axis',(1.,0.,0.));
#21206=DIRECTION('center_axis',(0.,0.,1.));
#21207=DIRECTION('ref_axis',(1.,0.,0.));
#21208=DIRECTION('center_axis',(0.,0.,1.));
#21209=DIRECTION('ref_axis',(1.,0.,0.));
#21210=DIRECTION('center_axis',(0.,0.,1.));
#21211=DIRECTION('ref_axis',(1.,0.,0.));
#21212=DIRECTION('center_axis',(0.,0.,1.));
#21213=DIRECTION('ref_axis',(1.,0.,0.));
#21214=DIRECTION('center_axis',(0.,0.,1.));
#21215=DIRECTION('ref_axis',(1.,0.,0.));
#21216=DIRECTION('center_axis',(0.,0.,1.));
#21217=DIRECTION('ref_axis',(1.,0.,0.));
#21218=DIRECTION('center_axis',(0.,0.,1.));
#21219=DIRECTION('ref_axis',(1.,0.,0.));
#21220=DIRECTION('center_axis',(0.,0.,1.));
#21221=DIRECTION('ref_axis',(1.,0.,0.));
#21222=DIRECTION('center_axis',(0.,0.,1.));
#21223=DIRECTION('ref_axis',(1.,0.,0.));
#21224=DIRECTION('center_axis',(0.,0.,1.));
#21225=DIRECTION('ref_axis',(1.,0.,0.));
#21226=DIRECTION('center_axis',(0.,0.,1.));
#21227=DIRECTION('ref_axis',(1.,0.,0.));
#21228=DIRECTION('center_axis',(0.,0.,1.));
#21229=DIRECTION('ref_axis',(1.,0.,0.));
#21230=DIRECTION('center_axis',(0.,0.,1.));
#21231=DIRECTION('ref_axis',(1.,0.,0.));
#21232=DIRECTION('center_axis',(0.,0.,1.));
#21233=DIRECTION('ref_axis',(1.,0.,0.));
#21234=DIRECTION('center_axis',(0.969193219910809,0.246301649362969,0.));
#21235=DIRECTION('ref_axis',(0.,0.,-1.));
#21236=DIRECTION('',(-0.246301649362969,0.969193219910809,0.));
#21237=DIRECTION('',(0.,0.,-1.));
#21238=DIRECTION('center_axis',(0.,0.,-1.));
#21239=DIRECTION('ref_axis',(-0.669130606358858,-0.743144825477394,0.));
#21240=DIRECTION('center_axis',(0.,0.,1.));
#21241=DIRECTION('ref_axis',(-0.669130606358858,-0.743144825477394,0.));
#21242=DIRECTION('center_axis',(0.,0.,1.));
#21243=DIRECTION('ref_axis',(-0.719339800338695,-0.694658370458952,0.));
#21244=DIRECTION('center_axis',(0.,0.,1.));
#21245=DIRECTION('ref_axis',(0.719339800338651,0.694658370458997,0.));
#21246=DIRECTION('center_axis',(0.,0.,1.));
#21247=DIRECTION('ref_axis',(-0.669130606358858,-0.743144825477394,0.));
#21248=DIRECTION('center_axis',(0.,0.,1.));
#21249=DIRECTION('ref_axis',(0.669130606358858,0.743144825477394,0.));
#21250=DIRECTION('center_axis',(0.584125431965383,0.811663402976415,0.));
#21251=DIRECTION('ref_axis',(0.,0.,-1.));
#21252=DIRECTION('',(0.,0.,1.));
#21253=DIRECTION('',(-0.811663402976415,0.584125431965383,0.));
#21254=DIRECTION('',(0.,0.,-1.));
#21255=DIRECTION('center_axis',(0.,0.,-1.));
#21256=DIRECTION('ref_axis',(-0.104528463267653,-0.994521895368273,0.));
#21257=DIRECTION('center_axis',(0.,0.,1.));
#21258=DIRECTION('ref_axis',(-0.104528463267653,-0.994521895368273,0.));
#21259=DIRECTION('center_axis',(0.,0.,1.));
#21260=DIRECTION('ref_axis',(-0.104528463267749,-0.994521895368263,0.));
#21261=DIRECTION('center_axis',(0.,0.,1.));
#21262=DIRECTION('ref_axis',(0.104528463267653,0.994521895368273,0.));
#21263=DIRECTION('',(0.,0.,1.));
#21264=DIRECTION('center_axis',(-0.402606579317095,0.91537311643427,0.));
#21265=DIRECTION('ref_axis',(0.,0.,1.));
#21266=DIRECTION('',(-0.91537311643427,-0.402606579317095,0.));
#21267=DIRECTION('',(0.,0.,-1.));
#21268=DIRECTION('center_axis',(0.639321308629955,0.76893970136265,0.));
#21269=DIRECTION('ref_axis',(0.,0.,-1.));
#21270=DIRECTION('',(0.,0.,1.));
#21271=DIRECTION('',(-0.76893970136265,0.639321308629955,0.));
#21272=DIRECTION('',(0.,0.,-1.));
#21273=DIRECTION('center_axis',(0.,0.,-1.));
#21274=DIRECTION('ref_axis',(-0.17364817766693,-0.984807753012208,0.));
#21275=DIRECTION('center_axis',(0.,0.,1.));
#21276=DIRECTION('ref_axis',(-0.17364817766693,-0.984807753012208,0.));
#21277=DIRECTION('center_axis',(0.,0.,1.));
#21278=DIRECTION('ref_axis',(-0.173648177666931,-0.984807753012208,0.));
#21279=DIRECTION('center_axis',(0.,0.,1.));
#21280=DIRECTION('ref_axis',(0.17364817766693,0.984807753012208,0.));
#21281=DIRECTION('',(0.,0.,1.));
#21282=DIRECTION('center_axis',(-0.337772649161909,0.941227728808574,0.));
#21283=DIRECTION('ref_axis',(0.,0.,1.));
#21284=DIRECTION('',(-0.941227728808574,-0.337772649161909,0.));
#21285=DIRECTION('',(0.,0.,-1.));
#21286=DIRECTION('center_axis',(0.691402476143371,0.722469802817263,0.));
#21287=DIRECTION('ref_axis',(0.,0.,-1.));
#21288=DIRECTION('',(0.,0.,1.));
#21289=DIRECTION('',(-0.722469802817263,0.691402476143371,0.));
#21290=DIRECTION('',(0.,0.,-1.));
#21291=DIRECTION('center_axis',(0.,0.,-1.));
#21292=DIRECTION('ref_axis',(-0.241921895599668,-0.970295726275996,0.));
#21293=DIRECTION('center_axis',(0.,0.,1.));
#21294=DIRECTION('ref_axis',(-0.241921895599668,-0.970295726275996,0.));
#21295=DIRECTION('center_axis',(0.,0.,1.));
#21296=DIRECTION('ref_axis',(-0.241921895599672,-0.970295726275995,0.));
#21297=DIRECTION('center_axis',(0.,0.,1.));
#21298=DIRECTION('ref_axis',(0.241921895599668,0.970295726275996,0.));
#21299=DIRECTION('',(0.,0.,1.));
#21300=DIRECTION('center_axis',(-0.27129312461327,0.962496774299825,0.));
#21301=DIRECTION('ref_axis',(0.,0.,1.));
#21302=DIRECTION('',(-0.962496774299825,-0.27129312461327,0.));
#21303=DIRECTION('',(0.,0.,-1.));
#21304=DIRECTION('center_axis',(0.740115200292261,0.672480104015239,0.));
#21305=DIRECTION('ref_axis',(0.,0.,-1.));
#21306=DIRECTION('',(0.,0.,1.));
#21307=DIRECTION('',(-0.672480104015239,0.740115200292261,0.));
#21308=DIRECTION('',(0.,0.,-1.));
#21309=DIRECTION('center_axis',(0.,0.,-1.));
#21310=DIRECTION('ref_axis',(-0.309016994374948,-0.951056516295154,0.));
#21311=DIRECTION('center_axis',(0.,0.,1.));
#21312=DIRECTION('ref_axis',(-0.309016994374947,-0.951056516295154,0.));
#21313=DIRECTION('center_axis',(0.,0.,1.));
#21314=DIRECTION('ref_axis',(-0.309016994374943,-0.951056516295155,0.));
#21315=DIRECTION('center_axis',(0.,0.,1.));
#21316=DIRECTION('ref_axis',(0.309016994374947,0.951056516295154,0.));
#21317=DIRECTION('',(0.,0.,1.));
#21318=DIRECTION('center_axis',(-0.203491887231385,0.979076632256643,0.));
#21319=DIRECTION('ref_axis',(0.,0.,1.));
#21320=DIRECTION('',(-0.979076632256643,-0.203491887231385,0.));
#21321=DIRECTION('',(0.,0.,-1.));
#21322=DIRECTION('center_axis',(0.785222157581596,0.619214149743772,0.));
#21323=DIRECTION('ref_axis',(0.,0.,-1.));
#21324=DIRECTION('',(0.,0.,1.));
#21325=DIRECTION('',(-0.619214149743772,0.785222157581596,0.));
#21326=DIRECTION('',(0.,0.,-1.));
#21327=DIRECTION('center_axis',(0.,0.,-1.));
#21328=DIRECTION('ref_axis',(-0.374606593415912,-0.927183854566787,0.));
#21329=DIRECTION('center_axis',(0.,0.,1.));
#21330=DIRECTION('ref_axis',(-0.374606593415912,-0.927183854566787,0.));
#21331=DIRECTION('center_axis',(0.,0.,1.));
#21332=DIRECTION('ref_axis',(-0.374606593415899,-0.927183854566793,0.));
#21333=DIRECTION('center_axis',(0.,0.,1.));
#21334=DIRECTION('ref_axis',(0.374606593415912,0.927183854566787,0.));
#21335=DIRECTION('',(0.,0.,1.));
#21336=DIRECTION('center_axis',(-0.134699257830059,0.990886527277484,0.));
#21337=DIRECTION('ref_axis',(0.,0.,1.));
#21338=DIRECTION('',(-0.990886527277484,-0.134699257830059,0.));
#21339=DIRECTION('',(0.,0.,-1.));
#21340=DIRECTION('center_axis',(0.826503591449444,0.56293144637795,0.));
#21341=DIRECTION('ref_axis',(0.,0.,-1.));
#21342=DIRECTION('',(0.,0.,1.));
#21343=DIRECTION('',(-0.56293144637795,0.826503591449444,0.));
#21344=DIRECTION('',(0.,0.,-1.));
#21345=DIRECTION('center_axis',(0.,0.,-1.));
#21346=DIRECTION('ref_axis',(-0.438371146789078,-0.898794046299167,0.));
#21347=DIRECTION('center_axis',(0.,0.,1.));
#21348=DIRECTION('ref_axis',(-0.438371146789077,-0.898794046299167,0.));
#21349=DIRECTION('center_axis',(0.,0.,1.));
#21350=DIRECTION('ref_axis',(-0.438371146789136,-0.898794046299139,0.));
#21351=DIRECTION('center_axis',(0.,0.,1.));
#21352=DIRECTION('ref_axis',(0.438371146789077,0.898794046299167,0.));
#21353=DIRECTION('',(0.,0.,1.));
#21354=DIRECTION('center_axis',(-0.0652503871847199,0.99786892274098,0.));
#21355=DIRECTION('ref_axis',(0.,0.,1.));
#21356=DIRECTION('',(-0.99786892274098,-0.0652503871847199,0.));
#21357=DIRECTION('',(0.,0.,-1.));
#21358=DIRECTION('center_axis',(0.863758382899708,0.503906197590862,0.));
#21359=DIRECTION('ref_axis',(0.,0.,-1.));
#21360=DIRECTION('',(0.,0.,1.));
#21361=DIRECTION('',(-0.503906197590862,0.863758382899708,0.));
#21362=DIRECTION('',(0.,0.,-1.));
#21363=DIRECTION('center_axis',(0.,0.,-1.));
#21364=DIRECTION('ref_axis',(-0.5,-0.866025403784438,0.));
#21365=DIRECTION('center_axis',(0.,0.,1.));
#21366=DIRECTION('ref_axis',(-0.5,-0.866025403784439,0.));
#21367=DIRECTION('center_axis',(0.,0.,1.));
#21368=DIRECTION('ref_axis',(-0.500000000000006,-0.866025403784435,0.));
#21369=DIRECTION('center_axis',(0.,0.,1.));
#21370=DIRECTION('ref_axis',(0.5,0.866025403784439,0.));
#21371=DIRECTION('',(0.,0.,1.));
#21372=DIRECTION('center_axis',(0.0045163767882446,0.999989801118345,0.));
#21373=DIRECTION('ref_axis',(0.,0.,1.));
#21374=DIRECTION('',(-0.999989801118345,0.0045163767882446,0.));
#21375=DIRECTION('',(0.,0.,-1.));
#21376=DIRECTION('center_axis',(0.89680503033297,0.442425968461935,0.));
#21377=DIRECTION('ref_axis',(0.,0.,-1.));
#21378=DIRECTION('',(0.,0.,1.));
#21379=DIRECTION('',(-0.442425968461935,0.89680503033297,0.));
#21380=DIRECTION('',(0.,0.,-1.));
#21381=DIRECTION('center_axis',(0.,0.,-1.));
#21382=DIRECTION('ref_axis',(-0.559192903470747,-0.829037572555042,0.));
#21383=DIRECTION('center_axis',(0.,0.,1.));
#21384=DIRECTION('ref_axis',(-0.559192903470747,-0.829037572555042,0.));
#21385=DIRECTION('center_axis',(0.,0.,1.));
#21386=DIRECTION('ref_axis',(-0.559192903470747,-0.829037572555042,0.));
#21387=DIRECTION('center_axis',(0.,0.,1.));
#21388=DIRECTION('ref_axis',(0.559192903470747,0.829037572555042,0.));
#21389=DIRECTION('',(0.,0.,1.));
#21390=DIRECTION('center_axis',(0.925482533805075,0.378790284486995,0.));
#21391=DIRECTION('ref_axis',(0.,0.,-1.));
#21392=DIRECTION('',(0.,0.,1.));
#21393=DIRECTION('',(-0.378790284486995,0.925482533805075,0.));
#21394=DIRECTION('',(0.,0.,-1.));
#21395=DIRECTION('center_axis',(0.,0.,1.));
#21396=DIRECTION('ref_axis',(1.,0.,0.));
#21397=DIRECTION('center_axis',(0.,0.,-1.));
#21398=DIRECTION('ref_axis',(1.,0.,0.));
#21399=DIRECTION('',(0.,0.,-1.));
#21400=DIRECTION('center_axis',(0.,0.,1.));
#21401=DIRECTION('ref_axis',(1.,0.,0.));
#21402=DIRECTION('center_axis',(0.,0.,1.));
#21403=DIRECTION('ref_axis',(1.,0.,0.));
#21404=DIRECTION('center_axis',(0.0742611374276901,0.997238829703269,0.));
#21405=DIRECTION('ref_axis',(0.,0.,1.));
#21406=DIRECTION('',(-0.997238829703269,0.0742611374276901,0.));
#21407=DIRECTION('center_axis',(-0.526083754912358,0.850432762078998,0.));
#21408=DIRECTION('ref_axis',(0.,0.,1.));
#21409=DIRECTION('',(-0.850432762078998,-0.526083754912358,0.));
#21410=DIRECTION('',(0.,0.,-1.));
#21411=DIRECTION('',(0.,0.,1.));
#21412=DIRECTION('center_axis',(0.,0.,1.));
#21413=DIRECTION('ref_axis',(1.,0.,0.));
#21414=DIRECTION('center_axis',(0.,0.,-1.));
#21415=DIRECTION('ref_axis',(1.,0.,0.));
#21416=DIRECTION('center_axis',(0.,0.,1.));
#21417=DIRECTION('ref_axis',(1.,0.,0.));
#21418=DIRECTION('center_axis',(0.,0.,1.));
#21419=DIRECTION('ref_axis',(1.,0.,0.));
#21420=DIRECTION('',(0.,0.,1.));
#21421=DIRECTION('center_axis',(-0.465479050687347,0.885058898249832,0.));
#21422=DIRECTION('ref_axis',(0.,0.,1.));
#21423=DIRECTION('',(0.,0.,1.));
#21424=DIRECTION('',(-0.885058898249832,-0.465479050687346,0.));
#21425=DIRECTION('',(0.,0.,-1.));
#21426=DIRECTION('center_axis',(0.,0.,1.));
#21427=DIRECTION('ref_axis',(1.,0.,0.));
#21428=DIRECTION('center_axis',(0.,0.,-1.));
#21429=DIRECTION('ref_axis',(1.,0.,0.));
#21430=DIRECTION('center_axis',(0.,0.,1.));
#21431=DIRECTION('ref_axis',(1.,0.,0.));
#21432=DIRECTION('center_axis',(0.,0.,-1.));
#21433=DIRECTION('ref_axis',(1.,0.,0.));
#21434=DIRECTION('center_axis',(0.,0.,1.));
#21435=DIRECTION('ref_axis',(1.,0.,0.));
#21436=DIRECTION('center_axis',(0.,0.,-1.));
#21437=DIRECTION('ref_axis',(1.,0.,0.));
#21438=DIRECTION('center_axis',(0.,0.,1.));
#21439=DIRECTION('ref_axis',(1.,0.,0.));
#21440=DIRECTION('center_axis',(0.,0.,-1.));
#21441=DIRECTION('ref_axis',(1.,0.,0.));
#21442=DIRECTION('center_axis',(0.,0.,1.));
#21443=DIRECTION('ref_axis',(1.,0.,0.));
#21444=DIRECTION('center_axis',(0.,0.,-1.));
#21445=DIRECTION('ref_axis',(1.,0.,0.));
#21446=DIRECTION('center_axis',(0.,0.,1.));
#21447=DIRECTION('ref_axis',(1.,0.,0.));
#21448=DIRECTION('center_axis',(0.,0.,-1.));
#21449=DIRECTION('ref_axis',(1.,0.,0.));
#21450=DIRECTION('center_axis',(0.,0.,1.));
#21451=DIRECTION('ref_axis',(1.,0.,0.));
#21452=DIRECTION('center_axis',(0.,0.,-1.));
#21453=DIRECTION('ref_axis',(1.,0.,0.));
#21454=DIRECTION('center_axis',(0.,0.,1.));
#21455=DIRECTION('ref_axis',(1.,0.,0.));
#21456=DIRECTION('center_axis',(0.,0.,-1.));
#21457=DIRECTION('ref_axis',(1.,0.,0.));
#21458=DIRECTION('center_axis',(0.,0.,1.));
#21459=DIRECTION('ref_axis',(1.,0.,0.));
#21460=DIRECTION('center_axis',(0.,0.,1.));
#21461=DIRECTION('ref_axis',(1.,0.,0.));
#21462=DIRECTION('center_axis',(0.,0.,1.));
#21463=DIRECTION('ref_axis',(1.,0.,0.));
#21464=DIRECTION('center_axis',(0.,0.,1.));
#21465=DIRECTION('ref_axis',(1.,0.,0.));
#21466=DIRECTION('center_axis',(0.,0.,1.));
#21467=DIRECTION('ref_axis',(1.,0.,0.));
#21468=DIRECTION('center_axis',(0.,0.,1.));
#21469=DIRECTION('ref_axis',(1.,0.,0.));
#21470=DIRECTION('center_axis',(0.,0.,1.));
#21471=DIRECTION('ref_axis',(1.,0.,0.));
#21472=DIRECTION('center_axis',(0.,0.,1.));
#21473=DIRECTION('ref_axis',(1.,0.,0.));
#21474=DIRECTION('center_axis',(0.,0.,1.));
#21475=DIRECTION('ref_axis',(1.,0.,0.));
#21476=DIRECTION('center_axis',(0.,0.,1.));
#21477=DIRECTION('ref_axis',(1.,0.,0.));
#21478=DIRECTION('center_axis',(0.,0.,1.));
#21479=DIRECTION('ref_axis',(1.,0.,0.));
#21480=DIRECTION('center_axis',(0.,0.,1.));
#21481=DIRECTION('ref_axis',(1.,0.,0.));
#21482=DIRECTION('center_axis',(0.,0.,1.));
#21483=DIRECTION('ref_axis',(1.,0.,0.));
#21484=DIRECTION('center_axis',(0.,0.,1.));
#21485=DIRECTION('ref_axis',(1.,0.,0.));
#21486=DIRECTION('center_axis',(0.,0.,1.));
#21487=DIRECTION('ref_axis',(1.,0.,0.));
#21488=DIRECTION('center_axis',(0.,0.,1.));
#21489=DIRECTION('ref_axis',(1.,0.,0.));
#21490=DIRECTION('center_axis',(0.526083754912358,0.850432762078998,0.));
#21491=DIRECTION('ref_axis',(0.,0.,-1.));
#21492=DIRECTION('',(-0.850432762078998,0.526083754912358,0.));
#21493=DIRECTION('',(0.,0.,-1.));
#21494=DIRECTION('center_axis',(0.,0.,1.));
#21495=DIRECTION('ref_axis',(-0.0348994967025649,-0.999390827019094,0.));
#21496=DIRECTION('center_axis',(0.,0.,1.));
#21497=DIRECTION('ref_axis',(0.0348994967025011,0.999390827019096,0.));
#21498=DIRECTION('center_axis',(-0.949651179401728,0.313309172321697,0.));
#21499=DIRECTION('ref_axis',(0.,0.,1.));
#21500=DIRECTION('',(-0.313309172321697,-0.949651179401728,0.));
#21501=DIRECTION('',(0.,0.,-1.));
#21502=DIRECTION('',(0.,0.,1.));
#21503=DIRECTION('center_axis',(0.,0.,1.));
#21504=DIRECTION('ref_axis',(-1.,0.,0.));
#21505=DIRECTION('center_axis',(0.,0.,-1.));
#21506=DIRECTION('ref_axis',(-1.,0.,0.));
#21507=DIRECTION('center_axis',(0.,0.,1.));
#21508=DIRECTION('ref_axis',(1.,0.,0.));
#21509=DIRECTION('center_axis',(0.,0.,1.));
#21510=DIRECTION('ref_axis',(1.,0.,0.));
#21511=DIRECTION('',(0.,0.,1.));
#21512=DIRECTION('center_axis',(-0.143644105269892,0.989629410952005,0.));
#21513=DIRECTION('ref_axis',(0.,0.,1.));
#21514=DIRECTION('',(-0.989629410952005,-0.143644105269892,0.));
#21515=DIRECTION('',(0.,0.,-1.));
#21516=DIRECTION('center_axis',(-0.925482533805075,0.378790284486995,0.));
#21517=DIRECTION('ref_axis',(0.,0.,1.));
#21518=DIRECTION('',(-0.378790284486995,-0.925482533805075,0.));
#21519=DIRECTION('',(0.,0.,-1.));
#21520=DIRECTION('',(0.,0.,1.));
#21521=DIRECTION('center_axis',(0.,0.,1.));
#21522=DIRECTION('ref_axis',(-1.,0.,0.));
#21523=DIRECTION('center_axis',(0.,0.,-1.));
#21524=DIRECTION('ref_axis',(-1.,0.,0.));
#21525=DIRECTION('center_axis',(0.,0.,1.));
#21526=DIRECTION('ref_axis',(1.,0.,0.));
#21527=DIRECTION('center_axis',(0.,0.,1.));
#21528=DIRECTION('ref_axis',(1.,0.,0.));
#21529=DIRECTION('',(0.,0.,1.));
#21530=DIRECTION('center_axis',(-0.0742611374276901,0.997238829703269,0.));
#21531=DIRECTION('ref_axis',(0.,0.,1.));
#21532=DIRECTION('',(-0.997238829703269,-0.0742611374276901,0.));
#21533=DIRECTION('',(0.,0.,-1.));
#21534=DIRECTION('center_axis',(-0.89680503033297,0.442425968461935,0.));
#21535=DIRECTION('ref_axis',(0.,0.,1.));
#21536=DIRECTION('',(-0.442425968461935,-0.89680503033297,0.));
#21537=DIRECTION('',(0.,0.,-1.));
#21538=DIRECTION('',(0.,0.,1.));
#21539=DIRECTION('center_axis',(0.,0.,1.));
#21540=DIRECTION('ref_axis',(-1.,0.,0.));
#21541=DIRECTION('center_axis',(0.,0.,-1.));
#21542=DIRECTION('ref_axis',(-1.,0.,0.));
#21543=DIRECTION('center_axis',(0.,0.,1.));
#21544=DIRECTION('ref_axis',(1.,0.,0.));
#21545=DIRECTION('center_axis',(0.,0.,1.));
#21546=DIRECTION('ref_axis',(1.,0.,0.));
#21547=DIRECTION('',(0.,0.,1.));
#21548=DIRECTION('center_axis',(-0.0045163767882446,0.999989801118345,0.));
#21549=DIRECTION('ref_axis',(0.,0.,1.));
#21550=DIRECTION('',(-0.999989801118345,-0.0045163767882446,0.));
#21551=DIRECTION('',(0.,0.,-1.));
#21552=DIRECTION('center_axis',(-0.863758382899608,0.503906197591034,0.));
#21553=DIRECTION('ref_axis',(0.,0.,1.));
#21554=DIRECTION('',(-0.503906197591034,-0.863758382899608,0.));
#21555=DIRECTION('',(0.,0.,-1.));
#21556=DIRECTION('',(0.,0.,1.));
#21557=DIRECTION('center_axis',(0.,0.,1.));
#21558=DIRECTION('ref_axis',(-1.,0.,0.));
#21559=DIRECTION('center_axis',(0.,0.,-1.));
#21560=DIRECTION('ref_axis',(-1.,0.,0.));
#21561=DIRECTION('center_axis',(0.,0.,1.));
#21562=DIRECTION('ref_axis',(1.,0.,0.));
#21563=DIRECTION('center_axis',(0.,0.,1.));
#21564=DIRECTION('ref_axis',(1.,0.,0.));
#21565=DIRECTION('',(0.,0.,1.));
#21566=DIRECTION('center_axis',(0.065250387184499,0.997868922740995,0.));
#21567=DIRECTION('ref_axis',(0.,0.,1.));
#21568=DIRECTION('',(-0.997868922740995,0.065250387184499,0.));
#21569=DIRECTION('',(0.,0.,-1.));
#21570=DIRECTION('center_axis',(-0.826503591449438,0.562931446377958,0.));
#21571=DIRECTION('ref_axis',(0.,0.,1.));
#21572=DIRECTION('',(-0.562931446377958,-0.826503591449438,0.));
#21573=DIRECTION('',(0.,0.,-1.));
#21574=DIRECTION('',(0.,0.,1.));
#21575=DIRECTION('center_axis',(0.,0.,1.));
#21576=DIRECTION('ref_axis',(-1.,0.,0.));
#21577=DIRECTION('center_axis',(0.,0.,-1.));
#21578=DIRECTION('ref_axis',(-1.,0.,0.));
#21579=DIRECTION('center_axis',(0.,0.,1.));
#21580=DIRECTION('ref_axis',(1.,0.,0.));
#21581=DIRECTION('center_axis',(0.,0.,1.));
#21582=DIRECTION('ref_axis',(1.,0.,0.));
#21583=DIRECTION('',(0.,0.,1.));
#21584=DIRECTION('center_axis',(0.134699257830059,0.990886527277484,0.));
#21585=DIRECTION('ref_axis',(0.,0.,1.));
#21586=DIRECTION('',(-0.990886527277484,0.134699257830059,0.));
#21587=DIRECTION('',(0.,0.,-1.));
#21588=DIRECTION('center_axis',(-0.785222157581596,0.619214149743772,0.));
#21589=DIRECTION('ref_axis',(0.,0.,1.));
#21590=DIRECTION('',(-0.619214149743772,-0.785222157581596,0.));
#21591=DIRECTION('',(0.,0.,-1.));
#21592=DIRECTION('',(0.,0.,1.));
#21593=DIRECTION('center_axis',(0.,0.,1.));
#21594=DIRECTION('ref_axis',(-1.,0.,0.));
#21595=DIRECTION('center_axis',(0.,0.,-1.));
#21596=DIRECTION('ref_axis',(-1.,0.,0.));
#21597=DIRECTION('center_axis',(0.,0.,1.));
#21598=DIRECTION('ref_axis',(1.,0.,0.));
#21599=DIRECTION('center_axis',(0.,0.,1.));
#21600=DIRECTION('ref_axis',(1.,0.,0.));
#21601=DIRECTION('',(0.,0.,1.));
#21602=DIRECTION('center_axis',(0.203491887231601,0.979076632256598,0.));
#21603=DIRECTION('ref_axis',(0.,0.,1.));
#21604=DIRECTION('',(-0.979076632256598,0.203491887231601,0.));
#21605=DIRECTION('',(0.,0.,-1.));
#21606=DIRECTION('center_axis',(-0.740115200292264,0.672480104015236,0.));
#21607=DIRECTION('ref_axis',(0.,0.,1.));
#21608=DIRECTION('',(-0.672480104015236,-0.740115200292264,0.));
#21609=DIRECTION('',(0.,0.,-1.));
#21610=DIRECTION('',(0.,0.,1.));
#21611=DIRECTION('center_axis',(0.,0.,1.));
#21612=DIRECTION('ref_axis',(-1.,0.,0.));
#21613=DIRECTION('center_axis',(0.,0.,-1.));
#21614=DIRECTION('ref_axis',(-1.,0.,0.));
#21615=DIRECTION('center_axis',(0.,0.,1.));
#21616=DIRECTION('ref_axis',(1.,0.,0.));
#21617=DIRECTION('center_axis',(0.,0.,1.));
#21618=DIRECTION('ref_axis',(1.,0.,0.));
#21619=DIRECTION('',(0.,0.,1.));
#21620=DIRECTION('center_axis',(0.271293124613069,0.962496774299882,0.));
#21621=DIRECTION('ref_axis',(0.,0.,1.));
#21622=DIRECTION('',(-0.962496774299882,0.271293124613069,0.));
#21623=DIRECTION('',(0.,0.,-1.));
#21624=DIRECTION('center_axis',(-0.691402476143223,0.722469802817405,0.));
#21625=DIRECTION('ref_axis',(0.,0.,1.));
#21626=DIRECTION('',(-0.722469802817405,-0.691402476143223,0.));
#21627=DIRECTION('',(0.,0.,-1.));
#21628=DIRECTION('',(0.,0.,1.));
#21629=DIRECTION('center_axis',(0.,0.,1.));
#21630=DIRECTION('ref_axis',(-1.,0.,0.));
#21631=DIRECTION('center_axis',(0.,0.,-1.));
#21632=DIRECTION('ref_axis',(-1.,0.,0.));
#21633=DIRECTION('center_axis',(0.,0.,1.));
#21634=DIRECTION('ref_axis',(1.,0.,0.));
#21635=DIRECTION('center_axis',(0.,0.,1.));
#21636=DIRECTION('ref_axis',(1.,0.,0.));
#21637=DIRECTION('',(0.,0.,1.));
#21638=DIRECTION('center_axis',(0.337772649161909,0.941227728808574,0.));
#21639=DIRECTION('ref_axis',(0.,0.,1.));
#21640=DIRECTION('',(-0.941227728808574,0.337772649161909,0.));
#21641=DIRECTION('',(0.,0.,-1.));
#21642=DIRECTION('center_axis',(-0.639321308629956,0.768939701362649,0.));
#21643=DIRECTION('ref_axis',(0.,0.,1.));
#21644=DIRECTION('',(-0.768939701362649,-0.639321308629956,0.));
#21645=DIRECTION('',(0.,0.,-1.));
#21646=DIRECTION('',(0.,0.,1.));
#21647=DIRECTION('center_axis',(0.,0.,1.));
#21648=DIRECTION('ref_axis',(-1.,0.,0.));
#21649=DIRECTION('center_axis',(0.,0.,-1.));
#21650=DIRECTION('ref_axis',(-1.,0.,0.));
#21651=DIRECTION('center_axis',(0.,0.,1.));
#21652=DIRECTION('ref_axis',(1.,0.,0.));
#21653=DIRECTION('center_axis',(0.,0.,1.));
#21654=DIRECTION('ref_axis',(1.,0.,0.));
#21655=DIRECTION('',(0.,0.,1.));
#21656=DIRECTION('center_axis',(-0.584125431965383,0.811663402976415,0.));
#21657=DIRECTION('ref_axis',(0.,0.,1.));
#21658=DIRECTION('',(-0.811663402976415,-0.584125431965383,0.));
#21659=DIRECTION('',(0.,0.,1.));
#21660=DIRECTION('center_axis',(0.,0.,1.));
#21661=DIRECTION('ref_axis',(0.104528463267749,-0.994521895368263,0.));
#21662=DIRECTION('center_axis',(0.,0.,1.));
#21663=DIRECTION('ref_axis',(0.104528463267654,-0.994521895368273,0.));
#21664=DIRECTION('',(0.,0.,-1.));
#21665=DIRECTION('center_axis',(0.,0.,1.));
#21666=DIRECTION('ref_axis',(-0.104528463267654,0.994521895368273,0.));
#21667=DIRECTION('center_axis',(0.,0.,-1.));
#21668=DIRECTION('ref_axis',(0.104528463267654,-0.994521895368273,0.));
#21669=DIRECTION('center_axis',(0.402606579317095,0.91537311643427,0.));
#21670=DIRECTION('ref_axis',(0.,0.,1.));
#21671=DIRECTION('',(-0.91537311643427,0.402606579317095,0.));
#21672=DIRECTION('center_axis',(0.,0.,-1.));
#21673=DIRECTION('ref_axis',(0.615661475325658,-0.788010753606722,0.));
#21674=DIRECTION('center_axis',(0.,0.,1.));
#21675=DIRECTION('ref_axis',(0.615661475325658,-0.788010753606722,0.));
#21676=DIRECTION('center_axis',(0.,0.,-1.));
#21677=DIRECTION('ref_axis',(0.559192903470747,-0.829037572555042,0.));
#21678=DIRECTION('center_axis',(0.,0.,1.));
#21679=DIRECTION('ref_axis',(0.559192903470747,-0.829037572555042,0.));
#21680=DIRECTION('center_axis',(0.,0.,-1.));
#21681=DIRECTION('ref_axis',(0.5,-0.866025403784439,0.));
#21682=DIRECTION('center_axis',(0.,0.,1.));
#21683=DIRECTION('ref_axis',(0.5,-0.866025403784439,0.));
#21684=DIRECTION('center_axis',(0.,0.,-1.));
#21685=DIRECTION('ref_axis',(0.438371146789078,-0.898794046299167,0.));
#21686=DIRECTION('center_axis',(0.,0.,1.));
#21687=DIRECTION('ref_axis',(0.438371146789078,-0.898794046299167,0.));
#21688=DIRECTION('center_axis',(0.,0.,-1.));
#21689=DIRECTION('ref_axis',(0.374606593415912,-0.927183854566787,0.));
#21690=DIRECTION('center_axis',(0.,0.,1.));
#21691=DIRECTION('ref_axis',(0.374606593415912,-0.927183854566787,0.));
#21692=DIRECTION('center_axis',(0.,0.,-1.));
#21693=DIRECTION('ref_axis',(0.309016994374947,-0.951056516295154,0.));
#21694=DIRECTION('center_axis',(0.,0.,1.));
#21695=DIRECTION('ref_axis',(0.309016994374947,-0.951056516295154,0.));
#21696=DIRECTION('center_axis',(0.,0.,-1.));
#21697=DIRECTION('ref_axis',(0.241921895599668,-0.970295726275996,0.));
#21698=DIRECTION('center_axis',(0.,0.,1.));
#21699=DIRECTION('ref_axis',(0.241921895599668,-0.970295726275996,0.));
#21700=DIRECTION('center_axis',(0.,0.,-1.));
#21701=DIRECTION('ref_axis',(0.17364817766693,-0.984807753012208,0.));
#21702=DIRECTION('center_axis',(0.,0.,1.));
#21703=DIRECTION('ref_axis',(0.17364817766693,-0.984807753012208,0.));
#21704=DIRECTION('center_axis',(0.,0.,1.));
#21705=DIRECTION('ref_axis',(0.173648177666931,-0.984807753012208,0.));
#21706=DIRECTION('center_axis',(0.,0.,1.));
#21707=DIRECTION('ref_axis',(-0.17364817766693,0.984807753012208,0.));
#21708=DIRECTION('center_axis',(0.,0.,1.));
#21709=DIRECTION('ref_axis',(0.241921895599671,-0.970295726275996,0.));
#21710=DIRECTION('center_axis',(0.,0.,1.));
#21711=DIRECTION('ref_axis',(-0.241921895599668,0.970295726275996,0.));
#21712=DIRECTION('center_axis',(0.,0.,1.));
#21713=DIRECTION('ref_axis',(0.309016994374995,-0.951056516295138,0.));
#21714=DIRECTION('center_axis',(0.,0.,1.));
#21715=DIRECTION('ref_axis',(-0.309016994374947,0.951056516295154,0.));
#21716=DIRECTION('center_axis',(0.,0.,1.));
#21717=DIRECTION('ref_axis',(0.374606593415899,-0.927183854566793,0.));
#21718=DIRECTION('center_axis',(0.,0.,1.));
#21719=DIRECTION('ref_axis',(-0.374606593415912,0.927183854566787,0.));
#21720=DIRECTION('center_axis',(0.,0.,1.));
#21721=DIRECTION('ref_axis',(0.438371146789079,-0.898794046299166,0.));
#21722=DIRECTION('center_axis',(0.,0.,1.));
#21723=DIRECTION('ref_axis',(-0.438371146789078,0.898794046299167,0.));
#21724=DIRECTION('center_axis',(0.,0.,1.));
#21725=DIRECTION('ref_axis',(0.500000000000058,-0.866025403784405,0.));
#21726=DIRECTION('center_axis',(0.,0.,1.));
#21727=DIRECTION('ref_axis',(-0.5,0.866025403784439,0.));
#21728=DIRECTION('center_axis',(0.,0.,1.));
#21729=DIRECTION('ref_axis',(0.559192903470747,-0.829037572555042,0.));
#21730=DIRECTION('center_axis',(0.,0.,1.));
#21731=DIRECTION('ref_axis',(-0.559192903470747,0.829037572555042,0.));
#21732=DIRECTION('center_axis',(0.,0.,1.));
#21733=DIRECTION('ref_axis',(0.615661475325708,-0.788010753606683,0.));
#21734=DIRECTION('center_axis',(0.,0.,1.));
#21735=DIRECTION('ref_axis',(-0.615661475325658,0.788010753606722,0.));
#21736=DIRECTION('center_axis',(0.,0.,-1.));
#21737=DIRECTION('ref_axis',(1.,0.,0.));
#21738=DIRECTION('center_axis',(0.,0.,1.));
#21739=DIRECTION('ref_axis',(1.,0.,0.));
#21740=DIRECTION('',(-0.707106781186546,-8.65956056235491E-17,-0.707106781186549));
#21741=DIRECTION('center_axis',(0.,0.,1.));
#21742=DIRECTION('ref_axis',(1.,0.,0.));
#21743=DIRECTION('center_axis',(0.,0.,-1.));
#21744=DIRECTION('ref_axis',(1.,0.,0.));
#21745=DIRECTION('',(0.,0.,-1.));
#21746=DIRECTION('center_axis',(-0.952442453762929,-0.304718513172487,0.));
#21747=DIRECTION('ref_axis',(0.,0.,1.));
#21748=DIRECTION('',(0.,0.,1.));
#21749=DIRECTION('',(0.304718513172487,-0.952442453762929,0.));
#21750=DIRECTION('center_axis',(0.,0.,-1.));
#21751=DIRECTION('ref_axis',(0.961261695938319,-0.275637355816999,0.));
#21752=DIRECTION('center_axis',(0.,0.,1.));
#21753=DIRECTION('ref_axis',(0.961261695938319,-0.275637355816999,0.));
#21754=DIRECTION('center_axis',(0.,0.,-1.));
#21755=DIRECTION('ref_axis',(0.939692620785908,-0.342020143325669,0.));
#21756=DIRECTION('center_axis',(0.,0.,1.));
#21757=DIRECTION('ref_axis',(0.939692620785908,-0.342020143325669,0.));
#21758=DIRECTION('center_axis',(0.,0.,-1.));
#21759=DIRECTION('ref_axis',(0.913545457642601,-0.4067366430758,0.));
#21760=DIRECTION('center_axis',(0.,0.,1.));
#21761=DIRECTION('ref_axis',(0.913545457642601,-0.4067366430758,0.));
#21762=DIRECTION('center_axis',(0.,0.,-1.));
#21763=DIRECTION('ref_axis',(0.882947592858927,-0.469471562785891,0.));
#21764=DIRECTION('center_axis',(0.,0.,1.));
#21765=DIRECTION('ref_axis',(0.882947592858927,-0.469471562785891,0.));
#21766=DIRECTION('center_axis',(0.,0.,-1.));
#21767=DIRECTION('ref_axis',(0.848048096156426,-0.529919264233205,0.));
#21768=DIRECTION('center_axis',(0.,0.,1.));
#21769=DIRECTION('ref_axis',(0.848048096156426,-0.529919264233205,0.));
#21770=DIRECTION('center_axis',(0.,0.,-1.));
#21771=DIRECTION('ref_axis',(0.809016994374947,-0.587785252292473,0.));
#21772=DIRECTION('center_axis',(0.,0.,1.));
#21773=DIRECTION('ref_axis',(0.809016994374947,-0.587785252292473,0.));
#21774=DIRECTION('center_axis',(0.,0.,-1.));
#21775=DIRECTION('ref_axis',(0.766044443118978,-0.642787609686539,0.));
#21776=DIRECTION('center_axis',(0.,0.,1.));
#21777=DIRECTION('ref_axis',(0.766044443118978,-0.642787609686539,0.));
#21778=DIRECTION('center_axis',(0.,0.,-1.));
#21779=DIRECTION('ref_axis',(0.719339800338651,-0.694658370458997,0.));
#21780=DIRECTION('center_axis',(0.,0.,1.));
#21781=DIRECTION('ref_axis',(0.719339800338651,-0.694658370458997,0.));
#21782=DIRECTION('center_axis',(0.,0.,1.));
#21783=DIRECTION('ref_axis',(0.669130606358858,-0.743144825477395,0.));
#21784=DIRECTION('center_axis',(0.,0.,1.));
#21785=DIRECTION('ref_axis',(-0.669130606358858,0.743144825477394,0.));
#21786=DIRECTION('center_axis',(0.,0.,1.));
#21787=DIRECTION('ref_axis',(0.719339800338695,-0.694658370458952,0.));
#21788=DIRECTION('center_axis',(0.,0.,1.));
#21789=DIRECTION('ref_axis',(-0.719339800338651,0.694658370458997,0.));
#21790=DIRECTION('center_axis',(0.,0.,1.));
#21791=DIRECTION('ref_axis',(0.76604444311897,-0.642787609686549,0.));
#21792=DIRECTION('center_axis',(0.,0.,1.));
#21793=DIRECTION('ref_axis',(-0.766044443118978,0.642787609686539,0.));
#21794=DIRECTION('center_axis',(0.,0.,1.));
#21795=DIRECTION('ref_axis',(0.809016994374945,-0.587785252292477,0.));
#21796=DIRECTION('center_axis',(0.,0.,1.));
#21797=DIRECTION('ref_axis',(-0.809016994374947,0.587785252292473,0.));
#21798=DIRECTION('center_axis',(0.,0.,1.));
#21799=DIRECTION('ref_axis',(0.848048096156423,-0.52991926423321,0.));
#21800=DIRECTION('center_axis',(0.,0.,1.));
#21801=DIRECTION('ref_axis',(-0.848048096156426,0.529919264233205,0.));
#21802=DIRECTION('center_axis',(0.,0.,1.));
#21803=DIRECTION('ref_axis',(0.882947592858954,-0.469471562785839,0.));
#21804=DIRECTION('center_axis',(0.,0.,1.));
#21805=DIRECTION('ref_axis',(-0.882947592858927,0.469471562785891,0.));
#21806=DIRECTION('center_axis',(0.,0.,1.));
#21807=DIRECTION('ref_axis',(0.913545457642601,-0.406736643075801,0.));
#21808=DIRECTION('center_axis',(0.,0.,1.));
#21809=DIRECTION('ref_axis',(-0.913545457642601,0.4067366430758,0.));
#21810=DIRECTION('center_axis',(0.,0.,1.));
#21811=DIRECTION('ref_axis',(0.939692620785906,-0.342020143325675,0.));
#21812=DIRECTION('center_axis',(0.,0.,1.));
#21813=DIRECTION('ref_axis',(-0.939692620785908,0.342020143325669,0.));
#21814=DIRECTION('center_axis',(0.,0.,1.));
#21815=DIRECTION('ref_axis',(0.96126169593832,-0.275637355816994,0.));
#21816=DIRECTION('center_axis',(0.,0.,1.));
#21817=DIRECTION('ref_axis',(-0.961261695938319,0.275637355816999,0.));
#21818=DIRECTION('center_axis',(-0.746159292170122,0.665767459934911,0.));
#21819=DIRECTION('ref_axis',(0.,0.,1.));
#21820=DIRECTION('',(0.,0.,1.));
#21821=DIRECTION('',(-0.665767459934911,-0.746159292170122,0.));
#21822=DIRECTION('',(0.,0.,-1.));
#21823=DIRECTION('center_axis',(0.,0.,1.));
#21824=DIRECTION('ref_axis',(0.978147600733817,-0.207911690817704,0.));
#21825=DIRECTION('center_axis',(0.,0.,1.));
#21826=DIRECTION('ref_axis',(-0.978147600733806,0.207911690817759,0.));
#21827=DIRECTION('center_axis',(-0.697900095297744,-0.716195124936913,0.));
#21828=DIRECTION('ref_axis',(0.,0.,1.));
#21829=DIRECTION('',(0.716195124936913,-0.697900095297744,0.));
#21830=DIRECTION('',(0.,0.,-1.));
#21831=DIRECTION('center_axis',(0.,0.,1.));
#21832=DIRECTION('ref_axis',(-1.,0.,0.));
#21833=DIRECTION('center_axis',(0.,0.,-1.));
#21834=DIRECTION('ref_axis',(-1.,0.,0.));
#21835=DIRECTION('center_axis',(-0.952442453762929,0.304718513172488,0.));
#21836=DIRECTION('ref_axis',(0.,0.,1.));
#21837=DIRECTION('',(0.,0.,1.));
#21838=DIRECTION('',(-0.304718513172488,-0.952442453762928,0.));
#21839=DIRECTION('',(0.,0.,-1.));
#21840=DIRECTION('center_axis',(0.,0.,1.));
#21841=DIRECTION('ref_axis',(0.978147600733804,0.207911690817768,0.));
#21842=DIRECTION('center_axis',(0.,0.,1.));
#21843=DIRECTION('ref_axis',(-0.978147600733806,-0.20791169081776,0.));
#21844=DIRECTION('',(0.,0.,1.));
#21845=DIRECTION('center_axis',(-0.900764728877144,-0.43430738332532,0.));
#21846=DIRECTION('ref_axis',(0.,0.,1.));
#21847=DIRECTION('',(0.,0.,1.));
#21848=DIRECTION('',(0.43430738332532,-0.900764728877144,0.));
#21849=DIRECTION('',(0.,0.,-1.));
#21850=DIRECTION('center_axis',(0.,0.,1.));
#21851=DIRECTION('ref_axis',(-1.,0.,0.));
#21852=DIRECTION('center_axis',(0.,0.,-1.));
#21853=DIRECTION('ref_axis',(-1.,0.,0.));
#21854=DIRECTION('center_axis',(-0.790783275974884,0.61209624279065,0.));
#21855=DIRECTION('ref_axis',(0.,0.,1.));
#21856=DIRECTION('',(0.,0.,1.));
#21857=DIRECTION('',(-0.61209624279065,-0.790783275974884,0.));
#21858=DIRECTION('center_axis',(0.,0.,1.));
#21859=DIRECTION('ref_axis',(0.997564050259824,-0.0697564737441227,0.));
#21860=DIRECTION('',(0.,0.,-1.));
#21861=DIRECTION('center_axis',(0.,0.,1.));
#21862=DIRECTION('ref_axis',(-0.997564050259824,0.0697564737441255,0.));
#21863=DIRECTION('center_axis',(-0.746159292170273,-0.665767459934741,0.));
#21864=DIRECTION('ref_axis',(0.,0.,1.));
#21865=DIRECTION('',(0.665767459934741,-0.746159292170273,0.));
#21866=DIRECTION('',(0.,0.,-1.));
#21867=DIRECTION('center_axis',(0.,0.,1.));
#21868=DIRECTION('ref_axis',(-1.,0.,0.));
#21869=DIRECTION('center_axis',(0.,0.,-1.));
#21870=DIRECTION('ref_axis',(-1.,0.,0.));
#21871=DIRECTION('center_axis',(-0.92886626285169,0.370415261208196,0.));
#21872=DIRECTION('ref_axis',(0.,0.,1.));
#21873=DIRECTION('',(0.,0.,1.));
#21874=DIRECTION('',(-0.370415261208196,-0.928866262851689,0.));
#21875=DIRECTION('',(0.,0.,-1.));
#21876=DIRECTION('center_axis',(0.,0.,1.));
#21877=DIRECTION('ref_axis',(0.99026806874158,0.139173100959998,0.));
#21878=DIRECTION('center_axis',(0.,0.,1.));
#21879=DIRECTION('ref_axis',(-0.99026806874157,-0.139173100960066,0.));
#21880=DIRECTION('',(0.,0.,1.));
#21881=DIRECTION('center_axis',(-0.868274759687958,-0.496083603527489,0.));
#21882=DIRECTION('ref_axis',(0.,0.,1.));
#21883=DIRECTION('',(0.,0.,1.));
#21884=DIRECTION('',(0.496083603527489,-0.868274759687958,0.));
#21885=DIRECTION('',(0.,0.,-1.));
#21886=DIRECTION('center_axis',(0.,0.,1.));
#21887=DIRECTION('ref_axis',(-1.,0.,0.));
#21888=DIRECTION('center_axis',(0.,0.,-1.));
#21889=DIRECTION('ref_axis',(-1.,0.,0.));
#21890=DIRECTION('center_axis',(-0.831554643148455,0.555442954279056,0.));
#21891=DIRECTION('ref_axis',(0.,0.,1.));
#21892=DIRECTION('',(0.,0.,1.));
#21893=DIRECTION('',(-0.555442954279056,-0.831554643148455,0.));
#21894=DIRECTION('center_axis',(0.,0.,1.));
#21895=DIRECTION('ref_axis',(1.,0.,0.));
#21896=DIRECTION('',(0.,0.,-1.));
#21897=DIRECTION('center_axis',(0.,0.,1.));
#21898=DIRECTION('ref_axis',(-1.,1.22464679914735E-16,0.));
#21899=DIRECTION('center_axis',(-0.790783275974884,-0.61209624279065,0.));
#21900=DIRECTION('ref_axis',(0.,0.,1.));
#21901=DIRECTION('',(0.61209624279065,-0.790783275974884,0.));
#21902=DIRECTION('',(0.,0.,-1.));
#21903=DIRECTION('center_axis',(0.,0.,1.));
#21904=DIRECTION('ref_axis',(-1.,0.,0.));
#21905=DIRECTION('center_axis',(0.,0.,-1.));
#21906=DIRECTION('ref_axis',(-1.,0.,0.));
#21907=DIRECTION('center_axis',(-0.900764728877053,0.434307383325507,0.));
#21908=DIRECTION('ref_axis',(0.,0.,1.));
#21909=DIRECTION('',(0.,0.,1.));
#21910=DIRECTION('',(-0.434307383325507,-0.900764728877053,0.));
#21911=DIRECTION('',(0.,0.,-1.));
#21912=DIRECTION('center_axis',(0.,0.,1.));
#21913=DIRECTION('ref_axis',(0.99756405025982,0.0697564737441876,0.));
#21914=DIRECTION('center_axis',(0.,0.,1.));
#21915=DIRECTION('ref_axis',(-0.997564050259824,-0.0697564737441253,0.));
#21916=DIRECTION('',(0.,0.,1.));
#21917=DIRECTION('center_axis',(-0.831554643148452,-0.555442954279061,0.));
#21918=DIRECTION('ref_axis',(0.,0.,1.));
#21919=DIRECTION('',(0.555442954279061,-0.831554643148452,0.));
#21920=DIRECTION('',(0.,0.,-1.));
#21921=DIRECTION('center_axis',(0.,0.,1.));
#21922=DIRECTION('ref_axis',(-1.,0.,0.));
#21923=DIRECTION('center_axis',(0.,0.,-1.));
#21924=DIRECTION('ref_axis',(-1.,0.,0.));
#21925=DIRECTION('center_axis',(-0.868274759687958,0.496083603527489,0.));
#21926=DIRECTION('ref_axis',(0.,0.,1.));
#21927=DIRECTION('',(0.,0.,1.));
#21928=DIRECTION('',(-0.496083603527489,-0.868274759687958,0.));
#21929=DIRECTION('center_axis',(0.,-9.18840917267949E-15,-1.));
#21930=DIRECTION('ref_axis',(1.,3.08644517216793E-17,0.));
#21931=DIRECTION('center_axis',(0.,0.,1.));
#21932=DIRECTION('ref_axis',(1.,6.12323399573677E-17,0.));
#21933=DIRECTION('',(0.923879532511287,3.43162438417493E-15,0.38268343236509));
#21934=DIRECTION('center_axis',(0.,0.,-1.));
#21935=DIRECTION('ref_axis',(1.,0.,0.));
#21936=DIRECTION('center_axis',(0.,0.,1.));
#21937=DIRECTION('ref_axis',(1.,0.,0.));
#21938=DIRECTION('center_axis',(0.,0.,1.));
#21939=DIRECTION('ref_axis',(1.,0.,0.));
#21940=DIRECTION('center_axis',(0.,0.,-1.));
#21941=DIRECTION('ref_axis',(1.,0.,0.));
#21942=DIRECTION('',(-0.707106781186547,-8.65956056235493E-17,-0.707106781186547));
#21943=DIRECTION('center_axis',(0.,0.,1.));
#21944=DIRECTION('ref_axis',(1.,0.,0.));
#21945=DIRECTION('center_axis',(0.,0.,1.));
#21946=DIRECTION('ref_axis',(1.,0.,0.));
#21947=DIRECTION('center_axis',(0.,0.,1.));
#21948=DIRECTION('ref_axis',(1.,0.,0.));
#21949=DIRECTION('center_axis',(0.,0.,1.));
#21950=DIRECTION('ref_axis',(1.,0.,0.));
#21951=DIRECTION('center_axis',(0.,0.,1.));
#21952=DIRECTION('ref_axis',(1.,0.,0.));
#21953=DIRECTION('center_axis',(0.,0.,1.));
#21954=DIRECTION('ref_axis',(1.,0.,0.));
#21955=DIRECTION('center_axis',(0.,0.,1.));
#21956=DIRECTION('ref_axis',(1.,0.,0.));
#21957=DIRECTION('center_axis',(0.,0.,1.));
#21958=DIRECTION('ref_axis',(1.,0.,0.));
#21959=DIRECTION('center_axis',(0.,0.,1.));
#21960=DIRECTION('ref_axis',(1.,0.,0.));
#21961=DIRECTION('center_axis',(0.,0.,1.));
#21962=DIRECTION('ref_axis',(1.,0.,0.));
#21963=DIRECTION('center_axis',(0.,0.,1.));
#21964=DIRECTION('ref_axis',(1.,0.,0.));
#21965=DIRECTION('center_axis',(0.,0.,1.));
#21966=DIRECTION('ref_axis',(1.,0.,0.));
#21967=DIRECTION('center_axis',(0.,0.,1.));
#21968=DIRECTION('ref_axis',(1.,0.,0.));
#21969=DIRECTION('center_axis',(0.,0.,1.));
#21970=DIRECTION('ref_axis',(1.,0.,0.));
#21971=DIRECTION('center_axis',(0.,0.,1.));
#21972=DIRECTION('ref_axis',(1.,0.,0.));
#21973=DIRECTION('center_axis',(0.,0.,1.));
#21974=DIRECTION('ref_axis',(1.,0.,0.));
#21975=DIRECTION('center_axis',(0.,0.,1.));
#21976=DIRECTION('ref_axis',(1.,0.,0.));
#21977=DIRECTION('center_axis',(0.,0.,1.));
#21978=DIRECTION('ref_axis',(1.,0.,0.));
#21979=DIRECTION('center_axis',(0.,0.,1.));
#21980=DIRECTION('ref_axis',(1.,0.,0.));
#21981=DIRECTION('center_axis',(0.,0.,1.));
#21982=DIRECTION('ref_axis',(1.,0.,0.));
#21983=DIRECTION('center_axis',(0.,0.,1.));
#21984=DIRECTION('ref_axis',(1.,0.,0.));
#21985=DIRECTION('center_axis',(0.,0.,1.));
#21986=DIRECTION('ref_axis',(1.,0.,0.));
#21987=DIRECTION('center_axis',(0.,0.,1.));
#21988=DIRECTION('ref_axis',(1.,0.,0.));
#21989=DIRECTION('center_axis',(0.,0.,1.));
#21990=DIRECTION('ref_axis',(1.,0.,0.));
#21991=DIRECTION('center_axis',(0.,0.,1.));
#21992=DIRECTION('ref_axis',(1.,0.,0.));
#21993=DIRECTION('center_axis',(0.,0.,1.));
#21994=DIRECTION('ref_axis',(1.,0.,0.));
#21995=DIRECTION('center_axis',(0.,0.,1.));
#21996=DIRECTION('ref_axis',(1.,0.,0.));
#21997=DIRECTION('center_axis',(0.,0.,1.));
#21998=DIRECTION('ref_axis',(1.,0.,0.));
#21999=DIRECTION('center_axis',(0.,0.,1.));
#22000=DIRECTION('ref_axis',(1.,0.,0.));
#22001=DIRECTION('center_axis',(0.,0.,1.));
#22002=DIRECTION('ref_axis',(1.,0.,0.));
#22003=DIRECTION('center_axis',(0.,0.,1.));
#22004=DIRECTION('ref_axis',(1.,0.,0.));
#22005=DIRECTION('center_axis',(0.,0.,1.));
#22006=DIRECTION('ref_axis',(1.,0.,0.));
#22007=DIRECTION('center_axis',(0.,0.,1.));
#22008=DIRECTION('ref_axis',(1.,0.,0.));
#22009=DIRECTION('center_axis',(0.,0.,1.));
#22010=DIRECTION('ref_axis',(1.,0.,0.));
#22011=DIRECTION('center_axis',(0.,0.,1.));
#22012=DIRECTION('ref_axis',(1.,0.,0.));
#22013=DIRECTION('center_axis',(0.,0.,1.));
#22014=DIRECTION('ref_axis',(1.,0.,0.));
#22015=DIRECTION('center_axis',(0.,0.,1.));
#22016=DIRECTION('ref_axis',(1.,0.,0.));
#22017=DIRECTION('center_axis',(0.,0.,1.));
#22018=DIRECTION('ref_axis',(1.,0.,0.));
#22019=DIRECTION('center_axis',(0.,0.,1.));
#22020=DIRECTION('ref_axis',(1.,0.,0.));
#22021=DIRECTION('center_axis',(0.,0.,1.));
#22022=DIRECTION('ref_axis',(1.,0.,0.));
#22023=DIRECTION('center_axis',(0.,0.,1.));
#22024=DIRECTION('ref_axis',(1.,0.,0.));
#22025=DIRECTION('center_axis',(0.,0.,1.));
#22026=DIRECTION('ref_axis',(1.,0.,0.));
#22027=DIRECTION('center_axis',(0.,0.,1.));
#22028=DIRECTION('ref_axis',(1.,0.,0.));
#22029=DIRECTION('center_axis',(0.,0.,1.));
#22030=DIRECTION('ref_axis',(1.,0.,0.));
#22031=DIRECTION('center_axis',(0.,0.,1.));
#22032=DIRECTION('ref_axis',(1.,0.,0.));
#22033=DIRECTION('center_axis',(0.,0.,1.));
#22034=DIRECTION('ref_axis',(1.,0.,0.));
#22035=DIRECTION('center_axis',(0.,0.,1.));
#22036=DIRECTION('ref_axis',(1.,0.,0.));
#22037=DIRECTION('center_axis',(0.,0.,1.));
#22038=DIRECTION('ref_axis',(1.,0.,0.));
#22039=DIRECTION('center_axis',(0.,0.,1.));
#22040=DIRECTION('ref_axis',(1.,0.,0.));
#22041=DIRECTION('center_axis',(0.,0.,1.));
#22042=DIRECTION('ref_axis',(1.,0.,0.));
#22043=DIRECTION('center_axis',(0.,0.,1.));
#22044=DIRECTION('ref_axis',(1.,0.,0.));
#22045=DIRECTION('center_axis',(0.,0.,1.));
#22046=DIRECTION('ref_axis',(1.,0.,0.));
#22047=DIRECTION('center_axis',(0.,0.,1.));
#22048=DIRECTION('ref_axis',(1.,0.,0.));
#22049=DIRECTION('center_axis',(0.,0.,1.));
#22050=DIRECTION('ref_axis',(1.,0.,0.));
#22051=DIRECTION('center_axis',(0.,0.,1.));
#22052=DIRECTION('ref_axis',(1.,0.,0.));
#22053=DIRECTION('center_axis',(0.,0.,1.));
#22054=DIRECTION('ref_axis',(1.,0.,0.));
#22055=DIRECTION('center_axis',(0.,0.,1.));
#22056=DIRECTION('ref_axis',(1.,0.,0.));
#22057=DIRECTION('center_axis',(0.,0.,1.));
#22058=DIRECTION('ref_axis',(1.,0.,0.));
#22059=DIRECTION('center_axis',(0.,0.,1.));
#22060=DIRECTION('ref_axis',(1.,0.,0.));
#22061=DIRECTION('center_axis',(0.,0.,1.));
#22062=DIRECTION('ref_axis',(1.,0.,0.));
#22063=DIRECTION('center_axis',(0.,0.,1.));
#22064=DIRECTION('ref_axis',(1.,0.,0.));
#22065=DIRECTION('center_axis',(0.,0.,1.));
#22066=DIRECTION('ref_axis',(1.,0.,0.));
#22067=DIRECTION('center_axis',(0.,0.,1.));
#22068=DIRECTION('ref_axis',(1.,0.,0.));
#22069=DIRECTION('center_axis',(0.,0.,1.));
#22070=DIRECTION('ref_axis',(1.,0.,0.));
#22071=DIRECTION('center_axis',(0.,0.,1.));
#22072=DIRECTION('ref_axis',(1.,0.,0.));
#22073=DIRECTION('center_axis',(0.,0.,1.));
#22074=DIRECTION('ref_axis',(1.,0.,0.));
#22075=DIRECTION('center_axis',(0.,0.,1.));
#22076=DIRECTION('ref_axis',(1.,0.,0.));
#22077=DIRECTION('center_axis',(0.,0.,1.));
#22078=DIRECTION('ref_axis',(1.,0.,0.));
#22079=DIRECTION('center_axis',(0.,0.,1.));
#22080=DIRECTION('ref_axis',(1.,0.,0.));
#22081=DIRECTION('center_axis',(0.,0.,1.));
#22082=DIRECTION('ref_axis',(1.,0.,0.));
#22083=DIRECTION('center_axis',(0.,0.,1.));
#22084=DIRECTION('ref_axis',(1.,0.,0.));
#22085=DIRECTION('center_axis',(0.,0.,1.));
#22086=DIRECTION('ref_axis',(1.,0.,0.));
#22087=DIRECTION('center_axis',(0.,0.,1.));
#22088=DIRECTION('ref_axis',(1.,0.,0.));
#22089=DIRECTION('center_axis',(0.,0.,1.));
#22090=DIRECTION('ref_axis',(1.,0.,0.));
#22091=DIRECTION('center_axis',(0.,0.,1.));
#22092=DIRECTION('ref_axis',(1.,0.,0.));
#22093=DIRECTION('center_axis',(0.,0.,1.));
#22094=DIRECTION('ref_axis',(1.,0.,0.));
#22095=DIRECTION('center_axis',(0.,0.,1.));
#22096=DIRECTION('ref_axis',(1.,0.,0.));
#22097=DIRECTION('center_axis',(0.,0.,1.));
#22098=DIRECTION('ref_axis',(1.,0.,0.));
#22099=DIRECTION('center_axis',(0.,0.,1.));
#22100=DIRECTION('ref_axis',(1.,0.,0.));
#22101=DIRECTION('center_axis',(0.,0.,1.));
#22102=DIRECTION('ref_axis',(1.,0.,0.));
#22103=DIRECTION('center_axis',(0.,0.,1.));
#22104=DIRECTION('ref_axis',(1.,0.,0.));
#22105=DIRECTION('center_axis',(0.,0.,1.));
#22106=DIRECTION('ref_axis',(1.,0.,0.));
#22107=DIRECTION('center_axis',(0.,0.,1.));
#22108=DIRECTION('ref_axis',(1.,0.,0.));
#22109=DIRECTION('center_axis',(0.,0.,1.));
#22110=DIRECTION('ref_axis',(1.,0.,0.));
#22111=DIRECTION('center_axis',(0.,0.,1.));
#22112=DIRECTION('ref_axis',(1.,0.,0.));
#22113=DIRECTION('center_axis',(0.,0.,1.));
#22114=DIRECTION('ref_axis',(1.,0.,0.));
#22115=DIRECTION('center_axis',(0.,0.,1.));
#22116=DIRECTION('ref_axis',(1.,0.,0.));
#22117=DIRECTION('center_axis',(0.,0.,1.));
#22118=DIRECTION('ref_axis',(1.,0.,0.));
#22119=DIRECTION('center_axis',(0.,0.,1.));
#22120=DIRECTION('ref_axis',(1.,0.,0.));
#22121=DIRECTION('center_axis',(0.,0.,1.));
#22122=DIRECTION('ref_axis',(1.,0.,0.));
#22123=DIRECTION('center_axis',(0.,0.,1.));
#22124=DIRECTION('ref_axis',(1.,0.,0.));
#22125=DIRECTION('center_axis',(0.,0.,1.));
#22126=DIRECTION('ref_axis',(1.,0.,0.));
#22127=DIRECTION('center_axis',(0.,0.,1.));
#22128=DIRECTION('ref_axis',(1.,0.,0.));
#22129=DIRECTION('center_axis',(0.,0.,1.));
#22130=DIRECTION('ref_axis',(1.,0.,0.));
#22131=DIRECTION('center_axis',(0.,0.,1.));
#22132=DIRECTION('ref_axis',(1.,0.,0.));
#22133=DIRECTION('center_axis',(0.,0.,1.));
#22134=DIRECTION('ref_axis',(1.,0.,0.));
#22135=DIRECTION('center_axis',(0.,0.,1.));
#22136=DIRECTION('ref_axis',(1.,0.,0.));
#22137=DIRECTION('center_axis',(0.,0.,1.));
#22138=DIRECTION('ref_axis',(1.,0.,0.));
#22139=DIRECTION('center_axis',(0.,0.,1.));
#22140=DIRECTION('ref_axis',(1.,0.,0.));
#22141=DIRECTION('center_axis',(0.,0.,1.));
#22142=DIRECTION('ref_axis',(1.,0.,0.));
#22143=DIRECTION('center_axis',(0.,0.,1.));
#22144=DIRECTION('ref_axis',(1.,0.,0.));
#22145=DIRECTION('center_axis',(0.,0.,1.));
#22146=DIRECTION('ref_axis',(1.,0.,0.));
#22147=DIRECTION('center_axis',(0.,0.,1.));
#22148=DIRECTION('ref_axis',(1.,0.,0.));
#22149=DIRECTION('',(0.707106781186548,8.65956056235493E-17,-0.707106781186548));
#22150=DIRECTION('center_axis',(0.,0.,-1.));
#22151=DIRECTION('ref_axis',(1.,0.,0.));
#22152=DIRECTION('center_axis',(0.,0.,1.));
#22153=DIRECTION('ref_axis',(1.,0.,0.));
#22154=DIRECTION('center_axis',(0.,0.,1.));
#22155=DIRECTION('ref_axis',(1.,0.,0.));
#22156=DIRECTION('center_axis',(0.,0.,1.));
#22157=DIRECTION('ref_axis',(1.,0.,0.));
#22158=DIRECTION('center_axis',(0.,0.,1.));
#22159=DIRECTION('ref_axis',(1.,0.,0.));
#22160=DIRECTION('center_axis',(0.,0.,-1.));
#22161=DIRECTION('ref_axis',(1.,0.,0.));
#22162=DIRECTION('center_axis',(0.,0.,1.));
#22163=DIRECTION('ref_axis',(1.,0.,0.));
#22164=DIRECTION('center_axis',(0.,0.,1.));
#22165=DIRECTION('ref_axis',(1.,0.,0.));
#22166=DIRECTION('center_axis',(0.,0.,-1.));
#22167=DIRECTION('ref_axis',(1.,0.,0.));
#22168=DIRECTION('',(0.,0.,-1.));
#22169=DIRECTION('center_axis',(0.,0.,1.));
#22170=DIRECTION('ref_axis',(1.,0.,0.));
#22171=DIRECTION('center_axis',(0.,0.,1.));
#22172=DIRECTION('ref_axis',(1.,0.,0.));
#22173=DIRECTION('',(0.707106781186548,8.65956056235493E-17,-0.707106781186548));
#22174=DIRECTION('center_axis',(0.,0.,-1.));
#22175=DIRECTION('ref_axis',(1.,0.,0.));
#22176=DIRECTION('center_axis',(0.,0.,-1.));
#22177=DIRECTION('ref_axis',(1.,0.,0.));
#22178=DIRECTION('',(0.,0.,-1.));
#22179=DIRECTION('center_axis',(0.,0.,1.));
#22180=DIRECTION('ref_axis',(1.,0.,0.));
#22181=DIRECTION('center_axis',(0.,0.,1.));
#22182=DIRECTION('ref_axis',(1.,0.,0.));
#22183=DIRECTION('',(0.707106781186548,8.65956056235493E-17,-0.707106781186548));
#22184=DIRECTION('center_axis',(0.,0.,-1.));
#22185=DIRECTION('ref_axis',(1.,0.,0.));
#22186=DIRECTION('center_axis',(0.,0.,-1.));
#22187=DIRECTION('ref_axis',(1.,0.,0.));
#22188=DIRECTION('',(0.,0.,-1.));
#22189=DIRECTION('center_axis',(0.,0.,1.));
#22190=DIRECTION('ref_axis',(1.,0.,0.));
#22191=DIRECTION('center_axis',(0.,0.,1.));
#22192=DIRECTION('ref_axis',(1.,0.,0.));
#22193=DIRECTION('',(0.707106781186548,8.65956056235493E-17,-0.707106781186548));
#22194=DIRECTION('center_axis',(0.,0.,-1.));
#22195=DIRECTION('ref_axis',(1.,0.,0.));
#22196=DIRECTION('center_axis',(0.,0.,-1.));
#22197=DIRECTION('ref_axis',(1.,0.,0.));
#22198=DIRECTION('',(0.,0.,-1.));
#22199=DIRECTION('center_axis',(0.,0.,1.));
#22200=DIRECTION('ref_axis',(1.,0.,0.));
#22201=DIRECTION('center_axis',(0.,0.,1.));
#22202=DIRECTION('ref_axis',(1.,0.,0.));
#22203=DIRECTION('',(0.707106781186548,8.65956056235493E-17,-0.707106781186548));
#22204=DIRECTION('center_axis',(0.,0.,-1.));
#22205=DIRECTION('ref_axis',(1.,0.,0.));
#22206=DIRECTION('center_axis',(0.,0.,-1.));
#22207=DIRECTION('ref_axis',(1.,0.,0.));
#22208=DIRECTION('',(0.,0.,-1.));
#22209=DIRECTION('center_axis',(0.,0.,1.));
#22210=DIRECTION('ref_axis',(1.,0.,0.));
#22211=DIRECTION('center_axis',(0.,0.,1.));
#22212=DIRECTION('ref_axis',(1.,0.,0.));
#22213=DIRECTION('',(0.707106781186545,8.6595605623549E-17,-0.70710678118655));
#22214=DIRECTION('center_axis',(0.,0.,-1.));
#22215=DIRECTION('ref_axis',(1.,0.,0.));
#22216=DIRECTION('center_axis',(0.,0.,1.));
#22217=DIRECTION('ref_axis',(1.,0.,0.));
#22218=DIRECTION('',(0.,0.,-1.));
#22219=DIRECTION('center_axis',(0.,0.,1.));
#22220=DIRECTION('ref_axis',(1.,0.,0.));
#22221=DIRECTION('center_axis',(0.,0.,1.));
#22222=DIRECTION('ref_axis',(1.,0.,0.));
#22223=DIRECTION('center_axis',(0.,0.,1.));
#22224=DIRECTION('ref_axis',(1.,0.,0.));
#22225=DIRECTION('center_axis',(0.,0.,1.));
#22226=DIRECTION('ref_axis',(1.,0.,0.));
#22227=DIRECTION('center_axis',(0.,0.,1.));
#22228=DIRECTION('ref_axis',(1.,0.,0.));
#22229=DIRECTION('center_axis',(0.,0.,1.));
#22230=DIRECTION('ref_axis',(1.,0.,0.));
#22231=DIRECTION('center_axis',(0.,0.,1.));
#22232=DIRECTION('ref_axis',(1.,0.,0.));
#22233=DIRECTION('center_axis',(0.,0.,1.));
#22234=DIRECTION('ref_axis',(1.,0.,0.));
#22235=DIRECTION('center_axis',(0.,0.,1.));
#22236=DIRECTION('ref_axis',(1.,0.,0.));
#22237=DIRECTION('center_axis',(0.,0.,1.));
#22238=DIRECTION('ref_axis',(1.,0.,0.));
#22239=DIRECTION('center_axis',(0.,0.,1.));
#22240=DIRECTION('ref_axis',(0.997564050259824,-0.0697564737441256,0.));
#22241=DIRECTION('center_axis',(0.,0.,1.));
#22242=DIRECTION('ref_axis',(0.99026806874157,-0.139173100960066,0.));
#22243=DIRECTION('center_axis',(0.,0.,1.));
#22244=DIRECTION('ref_axis',(0.978147600733805,-0.20791169081776,0.));
#22245=DIRECTION('center_axis',(0.,0.,1.));
#22246=DIRECTION('ref_axis',(0.961261695938319,-0.275637355816999,0.));
#22247=DIRECTION('center_axis',(0.,0.,1.));
#22248=DIRECTION('ref_axis',(0.939692620785909,-0.342020143325669,0.));
#22249=DIRECTION('center_axis',(0.,0.,1.));
#22250=DIRECTION('ref_axis',(0.913545457642601,-0.4067366430758,0.));
#22251=DIRECTION('center_axis',(0.,0.,1.));
#22252=DIRECTION('ref_axis',(-0.882947592858927,0.469471562785891,0.));
#22253=DIRECTION('center_axis',(0.,0.,1.));
#22254=DIRECTION('ref_axis',(0.882947592858927,-0.469471562785891,0.));
#22255=DIRECTION('center_axis',(0.,0.,1.));
#22256=DIRECTION('ref_axis',(0.882947592858927,-0.469471562785891,0.));
#22257=DIRECTION('center_axis',(0.,0.,1.));
#22258=DIRECTION('ref_axis',(0.848048096156426,-0.529919264233205,0.));
#22259=DIRECTION('center_axis',(0.,0.,1.));
#22260=DIRECTION('ref_axis',(0.809016994374947,-0.587785252292473,0.));
#22261=DIRECTION('center_axis',(0.,0.,1.));
#22262=DIRECTION('ref_axis',(0.766044443118978,-0.64278760968654,0.));
#22263=DIRECTION('center_axis',(0.,0.,1.));
#22264=DIRECTION('ref_axis',(0.719339800338651,-0.694658370458998,0.));
#22265=DIRECTION('center_axis',(0.,0.,1.));
#22266=DIRECTION('ref_axis',(0.669130606358858,-0.743144825477395,0.));
#22267=DIRECTION('center_axis',(0.,0.,1.));
#22268=DIRECTION('ref_axis',(0.615661475325659,-0.788010753606722,0.));
#22269=DIRECTION('center_axis',(0.,0.,1.));
#22270=DIRECTION('ref_axis',(0.559192903470747,-0.829037572555042,0.));
#22271=DIRECTION('center_axis',(0.,0.,1.));
#22272=DIRECTION('ref_axis',(0.5,-0.866025403784439,0.));
#22273=DIRECTION('center_axis',(0.,0.,1.));
#22274=DIRECTION('ref_axis',(0.438371146789077,-0.898794046299167,0.));
#22275=DIRECTION('center_axis',(0.,0.,1.));
#22276=DIRECTION('ref_axis',(-0.374606593415899,0.927183854566793,0.));
#22277=DIRECTION('center_axis',(0.,0.,1.));
#22278=DIRECTION('ref_axis',(0.374606593415912,-0.927183854566787,0.));
#22279=DIRECTION('center_axis',(0.,0.,1.));
#22280=DIRECTION('ref_axis',(0.374606593415912,-0.927183854566787,0.));
#22281=DIRECTION('center_axis',(0.,0.,1.));
#22282=DIRECTION('ref_axis',(0.309016994374947,-0.951056516295154,0.));
#22283=DIRECTION('center_axis',(0.,0.,1.));
#22284=DIRECTION('ref_axis',(0.241921895599667,-0.970295726275997,0.));
#22285=DIRECTION('center_axis',(0.,0.,1.));
#22286=DIRECTION('ref_axis',(0.17364817766693,-0.984807753012208,0.));
#22287=DIRECTION('center_axis',(0.,0.,1.));
#22288=DIRECTION('ref_axis',(0.104528463267653,-0.994521895368273,0.));
#22289=DIRECTION('center_axis',(0.,0.,1.));
#22290=DIRECTION('ref_axis',(0.0348994967025013,-0.999390827019096,0.));
#22291=DIRECTION('center_axis',(0.,0.,1.));
#22292=DIRECTION('ref_axis',(-0.0348994967025008,-0.999390827019096,0.));
#22293=DIRECTION('center_axis',(0.,0.,1.));
#22294=DIRECTION('ref_axis',(-0.104528463267653,-0.994521895368273,0.));
#22295=DIRECTION('center_axis',(0.,0.,1.));
#22296=DIRECTION('ref_axis',(-0.17364817766693,-0.984807753012208,0.));
#22297=DIRECTION('center_axis',(0.,0.,1.));
#22298=DIRECTION('ref_axis',(-0.241921895599668,-0.970295726275996,0.));
#22299=DIRECTION('center_axis',(0.,0.,1.));
#22300=DIRECTION('ref_axis',(0.309016994374881,0.951056516295175,0.));
#22301=DIRECTION('center_axis',(0.,0.,1.));
#22302=DIRECTION('ref_axis',(-0.309016994374948,-0.951056516295154,0.));
#22303=DIRECTION('center_axis',(0.,0.,1.));
#22304=DIRECTION('ref_axis',(-0.309016994374948,-0.951056516295153,0.));
#22305=DIRECTION('center_axis',(0.,0.,1.));
#22306=DIRECTION('ref_axis',(-0.374606593415912,-0.927183854566787,0.));
#22307=DIRECTION('center_axis',(0.,0.,1.));
#22308=DIRECTION('ref_axis',(-0.438371146789078,-0.898794046299167,0.));
#22309=DIRECTION('center_axis',(0.,0.,1.));
#22310=DIRECTION('ref_axis',(-0.5,-0.866025403784438,0.));
#22311=DIRECTION('center_axis',(0.,0.,1.));
#22312=DIRECTION('ref_axis',(-0.559192903470747,-0.829037572555042,0.));
#22313=DIRECTION('center_axis',(0.,0.,1.));
#22314=DIRECTION('ref_axis',(-0.615661475325658,-0.788010753606722,0.));
#22315=DIRECTION('center_axis',(0.,0.,1.));
#22316=DIRECTION('ref_axis',(-0.669130606358858,-0.743144825477394,0.));
#22317=DIRECTION('center_axis',(0.,0.,1.));
#22318=DIRECTION('ref_axis',(-0.719339800338651,-0.694658370458997,0.));
#22319=DIRECTION('center_axis',(0.,0.,1.));
#22320=DIRECTION('ref_axis',(-0.766044443118978,-0.642787609686539,0.));
#22321=DIRECTION('center_axis',(0.,0.,1.));
#22322=DIRECTION('ref_axis',(-0.809016994374947,-0.587785252292473,0.));
#22323=DIRECTION('center_axis',(0.,0.,1.));
#22324=DIRECTION('ref_axis',(-0.848048096156426,-0.529919264233205,0.));
#22325=DIRECTION('center_axis',(0.,0.,1.));
#22326=DIRECTION('ref_axis',(-0.882947592858927,-0.469471562785891,0.));
#22327=DIRECTION('center_axis',(0.,0.,1.));
#22328=DIRECTION('ref_axis',(-0.913545457642601,-0.4067366430758,0.));
#22329=DIRECTION('center_axis',(0.,0.,1.));
#22330=DIRECTION('ref_axis',(-0.939692620785909,-0.342020143325669,0.));
#22331=DIRECTION('center_axis',(0.,0.,1.));
#22332=DIRECTION('ref_axis',(-0.961261695938319,-0.275637355816999,0.));
#22333=DIRECTION('center_axis',(0.,0.,1.));
#22334=DIRECTION('ref_axis',(-0.978147600733805,-0.20791169081776,0.));
#22335=DIRECTION('center_axis',(0.,0.,1.));
#22336=DIRECTION('ref_axis',(-0.99026806874157,-0.139173100960066,0.));
#22337=DIRECTION('center_axis',(0.,0.,1.));
#22338=DIRECTION('ref_axis',(-0.997564050259824,-0.0697564737441253,0.));
#22339=DIRECTION('center_axis',(0.,0.,1.));
#22340=DIRECTION('ref_axis',(-1.,1.22464679914735E-16,0.));
#22341=DIRECTION('center_axis',(0.,0.,1.));
#22342=DIRECTION('ref_axis',(-0.997564050259824,0.0697564737441255,0.));
#22343=DIRECTION('center_axis',(0.,0.,1.));
#22344=DIRECTION('ref_axis',(-0.99026806874157,0.139173100960065,0.));
#22345=DIRECTION('center_axis',(0.,0.,1.));
#22346=DIRECTION('ref_axis',(-0.978147600733806,0.207911690817759,0.));
#22347=DIRECTION('center_axis',(0.,0.,1.));
#22348=DIRECTION('ref_axis',(-0.961261695938319,0.275637355816999,0.));
#22349=DIRECTION('center_axis',(0.,0.,1.));
#22350=DIRECTION('ref_axis',(-0.939692620785908,0.342020143325669,0.));
#22351=DIRECTION('center_axis',(0.,0.,1.));
#22352=DIRECTION('ref_axis',(-0.913545457642601,0.4067366430758,0.));
#22353=DIRECTION('center_axis',(0.,0.,1.));
#22354=DIRECTION('ref_axis',(-0.882947592858927,0.469471562785891,0.));
#22355=DIRECTION('center_axis',(0.,0.,1.));
#22356=DIRECTION('ref_axis',(-0.848048096156426,0.529919264233205,0.));
#22357=DIRECTION('center_axis',(0.,0.,1.));
#22358=DIRECTION('ref_axis',(-0.809016994374947,0.587785252292473,0.));
#22359=DIRECTION('center_axis',(0.,0.,1.));
#22360=DIRECTION('ref_axis',(-0.766044443118978,0.642787609686539,0.));
#22361=DIRECTION('center_axis',(0.,0.,1.));
#22362=DIRECTION('ref_axis',(-0.719339800338651,0.694658370458997,0.));
#22363=DIRECTION('center_axis',(0.,0.,1.));
#22364=DIRECTION('ref_axis',(-0.669130606358858,0.743144825477394,0.));
#22365=DIRECTION('center_axis',(0.,0.,1.));
#22366=DIRECTION('ref_axis',(-0.615661475325658,0.788010753606722,0.));
#22367=DIRECTION('center_axis',(0.,0.,1.));
#22368=DIRECTION('ref_axis',(-0.559192903470747,0.829037572555042,0.));
#22369=DIRECTION('center_axis',(0.,0.,1.));
#22370=DIRECTION('ref_axis',(-0.5,0.866025403784439,0.));
#22371=DIRECTION('center_axis',(0.,0.,1.));
#22372=DIRECTION('ref_axis',(-0.438371146789078,0.898794046299167,0.));
#22373=DIRECTION('center_axis',(0.,0.,1.));
#22374=DIRECTION('ref_axis',(-0.374606593415912,0.927183854566787,0.));
#22375=DIRECTION('center_axis',(0.,0.,1.));
#22376=DIRECTION('ref_axis',(-0.309016994374947,0.951056516295154,0.));
#22377=DIRECTION('center_axis',(0.,0.,1.));
#22378=DIRECTION('ref_axis',(-0.241921895599668,0.970295726275996,0.));
#22379=DIRECTION('center_axis',(0.,0.,1.));
#22380=DIRECTION('ref_axis',(-0.17364817766693,0.984807753012208,0.));
#22381=DIRECTION('center_axis',(0.,0.,1.));
#22382=DIRECTION('ref_axis',(-0.104528463267654,0.994521895368273,0.));
#22383=DIRECTION('center_axis',(0.,0.,1.));
#22384=DIRECTION('ref_axis',(-0.034899496702501,0.999390827019096,0.));
#22385=DIRECTION('center_axis',(0.,0.,1.));
#22386=DIRECTION('ref_axis',(-0.034899496702501,0.999390827019096,0.));
#22387=DIRECTION('center_axis',(0.,0.,1.));
#22388=DIRECTION('ref_axis',(0.0348994967025652,-0.999390827019094,0.));
#22389=DIRECTION('center_axis',(0.,0.,1.));
#22390=DIRECTION('ref_axis',(0.0348994967025011,0.999390827019096,0.));
#22391=DIRECTION('center_axis',(0.,0.,1.));
#22392=DIRECTION('ref_axis',(0.104528463267653,0.994521895368273,0.));
#22393=DIRECTION('center_axis',(0.,0.,1.));
#22394=DIRECTION('ref_axis',(0.17364817766693,0.984807753012208,0.));
#22395=DIRECTION('center_axis',(0.,0.,1.));
#22396=DIRECTION('ref_axis',(0.241921895599668,0.970295726275996,0.));
#22397=DIRECTION('center_axis',(0.,0.,1.));
#22398=DIRECTION('ref_axis',(0.309016994374948,0.951056516295154,0.));
#22399=DIRECTION('center_axis',(0.,0.,1.));
#22400=DIRECTION('ref_axis',(0.374606593415912,0.927183854566787,0.));
#22401=DIRECTION('center_axis',(0.,0.,1.));
#22402=DIRECTION('ref_axis',(0.438371146789078,0.898794046299167,0.));
#22403=DIRECTION('center_axis',(0.,0.,1.));
#22404=DIRECTION('ref_axis',(0.5,0.866025403784439,0.));
#22405=DIRECTION('center_axis',(0.,0.,1.));
#22406=DIRECTION('ref_axis',(0.559192903470747,0.829037572555042,0.));
#22407=DIRECTION('center_axis',(0.,0.,1.));
#22408=DIRECTION('ref_axis',(-0.615661475325708,-0.788010753606683,0.));
#22409=DIRECTION('center_axis',(0.,0.,1.));
#22410=DIRECTION('ref_axis',(0.615661475325658,0.788010753606722,0.));
#22411=DIRECTION('center_axis',(0.,0.,1.));
#22412=DIRECTION('ref_axis',(0.615661475325658,0.788010753606722,0.));
#22413=DIRECTION('center_axis',(0.,0.,1.));
#22414=DIRECTION('ref_axis',(0.669130606358858,0.743144825477394,0.));
#22415=DIRECTION('center_axis',(0.,0.,1.));
#22416=DIRECTION('ref_axis',(0.719339800338651,0.694658370458997,0.));
#22417=DIRECTION('center_axis',(0.,0.,1.));
#22418=DIRECTION('ref_axis',(0.766044443118978,0.642787609686539,0.));
#22419=DIRECTION('center_axis',(0.,0.,1.));
#22420=DIRECTION('ref_axis',(0.809016994374947,0.587785252292473,0.));
#22421=DIRECTION('center_axis',(0.,0.,1.));
#22422=DIRECTION('ref_axis',(0.848048096156426,0.529919264233205,0.));
#22423=DIRECTION('center_axis',(0.,0.,1.));
#22424=DIRECTION('ref_axis',(0.882947592858927,0.469471562785891,0.));
#22425=DIRECTION('center_axis',(0.,0.,1.));
#22426=DIRECTION('ref_axis',(0.913545457642601,0.4067366430758,0.));
#22427=DIRECTION('center_axis',(0.,0.,1.));
#22428=DIRECTION('ref_axis',(0.939692620785908,0.342020143325669,0.));
#22429=DIRECTION('center_axis',(0.,0.,1.));
#22430=DIRECTION('ref_axis',(0.961261695938319,0.275637355816999,0.));
#22431=DIRECTION('center_axis',(0.,0.,1.));
#22432=DIRECTION('ref_axis',(-0.978147600733819,-0.207911690817698,0.));
#22433=DIRECTION('center_axis',(0.,0.,1.));
#22434=DIRECTION('ref_axis',(0.978147600733806,0.207911690817759,0.));
#22435=DIRECTION('center_axis',(0.,0.,1.));
#22436=DIRECTION('ref_axis',(0.978147600733806,0.207911690817759,0.));
#22437=DIRECTION('center_axis',(0.,0.,1.));
#22438=DIRECTION('ref_axis',(0.99026806874157,0.139173100960065,0.));
#22439=DIRECTION('center_axis',(0.,0.,1.));
#22440=DIRECTION('ref_axis',(0.997564050259824,0.0697564737441253,0.));
#22441=DIRECTION('center_axis',(0.,0.,1.));
#22442=DIRECTION('ref_axis',(1.,0.,0.));
#22443=DIRECTION('center_axis',(0.,0.,-1.));
#22444=DIRECTION('ref_axis',(1.,0.,0.));
#22445=DIRECTION('center_axis',(0.,0.,1.));
#22446=DIRECTION('ref_axis',(1.,0.,0.));
#22447=DIRECTION('',(0.707106781186547,8.65956056235493E-17,0.707106781186548));
#22448=DIRECTION('center_axis',(0.,0.,-1.));
#22449=DIRECTION('ref_axis',(1.,0.,0.));
#22450=DIRECTION('center_axis',(0.,0.,1.));
#22451=DIRECTION('ref_axis',(1.,0.,0.));
#22452=DIRECTION('',(0.707106781186547,8.65956056235493E-17,0.707106781186548));
#22453=DIRECTION('center_axis',(0.,0.,-1.));
#22454=DIRECTION('ref_axis',(1.,0.,0.));
#22455=DIRECTION('center_axis',(0.,0.,1.));
#22456=DIRECTION('ref_axis',(1.,0.,0.));
#22457=DIRECTION('',(0.707106781186547,8.65956056235493E-17,0.707106781186548));
#22458=DIRECTION('center_axis',(0.,0.,-1.));
#22459=DIRECTION('ref_axis',(1.,0.,0.));
#22460=DIRECTION('center_axis',(0.,0.,1.));
#22461=DIRECTION('ref_axis',(1.,0.,0.));
#22462=DIRECTION('',(0.707106781186547,8.65956056235493E-17,0.707106781186548));
#22463=DIRECTION('center_axis',(0.,0.,-1.));
#22464=DIRECTION('ref_axis',(1.,0.,0.));
#22465=DIRECTION('center_axis',(0.,0.,1.));
#22466=DIRECTION('ref_axis',(1.,0.,0.));
#22467=DIRECTION('',(0.707106781186547,8.65956056235493E-17,0.707106781186548));
#22468=DIRECTION('center_axis',(0.,0.,-1.));
#22469=DIRECTION('ref_axis',(1.,0.,0.));
#22470=DIRECTION('',(0.,0.,-1.));
#22471=DIRECTION('center_axis',(0.,0.,1.));
#22472=DIRECTION('ref_axis',(1.,0.,0.));
#22473=DIRECTION('center_axis',(0.,0.,1.));
#22474=DIRECTION('ref_axis',(1.,0.,0.));
#23993=CARTESIAN_POINT('',(0.,0.,0.));
#23994=CARTESIAN_POINT('Origin',(-2.67770341754863,53.2125144041213,14.5));
#23995=CARTESIAN_POINT('',(-2.29739178302164,53.0124970957195,11.0622545443402));
#23996=CARTESIAN_POINT('',(-3.0580150520755,53.412531712523,11.5));
#23997=CARTESIAN_POINT('Ctrl Pts',(-2.29739178302164,53.0124970957195,11.0622545443402));
#23998=CARTESIAN_POINT('Ctrl Pts',(-2.67614114120178,53.2116927560792,11.2776618075212));
#23999=CARTESIAN_POINT('Ctrl Pts',(-3.0580150520755,53.412531712523,11.5));
#24000=CARTESIAN_POINT('',(-3.0580150520755,53.412531712523,24.2));
#24001=CARTESIAN_POINT('',(-3.0580150520755,53.412531712523,14.5));
#24002=CARTESIAN_POINT('',(-2.29739178302176,53.0124970957196,24.2));
#24003=CARTESIAN_POINT('',(-2.43468625658982,53.0847043819776,24.2));
#24004=CARTESIAN_POINT('',(-2.29739178302176,53.0124970957196,14.5));
#24005=CARTESIAN_POINT('Origin',(0.,0.,14.5));
#24006=CARTESIAN_POINT('',(-4.4053330087579,53.318318063138,11.5));
#24007=CARTESIAN_POINT('Origin',(0.,0.,11.5));
#24008=CARTESIAN_POINT('',(-4.4053330087579,53.318318063138,24.2));
#24009=CARTESIAN_POINT('',(-4.4053330087579,53.318318063138,14.5));
#24010=CARTESIAN_POINT('Origin',(0.,0.,24.2));
#24011=CARTESIAN_POINT('Origin',(0.,0.,11.25));
#24012=CARTESIAN_POINT('',(-2.20794196160078,52.953989389792,11.));
#24013=CARTESIAN_POINT('Ctrl Pts',(-2.20794196160078,52.953989389792,11.));
#24014=CARTESIAN_POINT('Ctrl Pts',(-2.24054943696625,52.9719225189241,11.0192759649605));
#24015=CARTESIAN_POINT('Ctrl Pts',(-2.27052551750933,52.9918321844726,11.0404458048696));
#24016=CARTESIAN_POINT('Ctrl Pts',(-2.29739178302161,53.0124970957195,11.0622545443403));
#24017=CARTESIAN_POINT('',(-4.51126784227788,52.8076553394982,11.));
#24018=CARTESIAN_POINT('Origin',(0.,0.,11.));
#24019=CARTESIAN_POINT('',(-4.72678212511287,53.0869825079594,11.2969997378715));
#24020=CARTESIAN_POINT('Ctrl Pts',(-4.51126784227788,52.8076553394982,11.));
#24021=CARTESIAN_POINT('Ctrl Pts',(-4.57608660062692,52.8996682008571,11.0971961933879));
#24022=CARTESIAN_POINT('Ctrl Pts',(-4.64844098161557,52.9953004405385,11.1987310576086));
#24023=CARTESIAN_POINT('Ctrl Pts',(-4.72678212511288,53.0869825079594,11.2969997378715));
#24024=CARTESIAN_POINT('Ctrl Pts',(-4.4053330087579,53.318318063138,11.5));
#24025=CARTESIAN_POINT('Ctrl Pts',(-4.56636307296567,53.2024304236684,11.3977655520829));
#24026=CARTESIAN_POINT('Ctrl Pts',(-4.72678212511287,53.0869825079594,11.2969997378715));
#24027=CARTESIAN_POINT('Origin',(-46.653263217121,-25.7335348523128,14.5));
#24028=CARTESIAN_POINT('',(-46.6542861332861,-25.7671839061264,11.2969997378715));
#24029=CARTESIAN_POINT('',(-46.6663199357044,-26.1630385020257,11.5));
#24030=CARTESIAN_POINT('Ctrl Pts',(-46.6542861332861,-25.7671839061264,
11.2969997378715));
#24031=CARTESIAN_POINT('Ctrl Pts',(-46.6602915975399,-25.9647349828961,
11.3977655520833));
#24032=CARTESIAN_POINT('Ctrl Pts',(-46.6663199357044,-26.1630385020257,
11.5));
#24033=CARTESIAN_POINT('',(-46.6663199357044,-26.1630385020257,24.2));
#24034=CARTESIAN_POINT('',(-46.6663199357044,-26.1630385020257,14.5));
#24035=CARTESIAN_POINT('',(-46.6402064985376,-25.3040312025999,24.2));
#24036=CARTESIAN_POINT('',(-46.6449200416998,-25.459084248916,24.2));
#24037=CARTESIAN_POINT('',(-46.6402064985376,-25.3040312025999,11.5));
#24038=CARTESIAN_POINT('',(-46.6402064985376,-25.3040312025999,14.5));
#24039=CARTESIAN_POINT('Ctrl Pts',(-46.6402064985376,-25.3040312025999,
11.5));
#24040=CARTESIAN_POINT('Ctrl Pts',(-46.6463548096495,-25.5062812584034,
11.4654707447275));
#24041=CARTESIAN_POINT('Ctrl Pts',(-46.6542861332861,-25.7671839061264,
11.2969997378715));
#24042=CARTESIAN_POINT('Origin',(0.,0.,14.5));
#24043=CARTESIAN_POINT('',(-45.9910159507968,-27.3326993144394,11.5));
#24044=CARTESIAN_POINT('Origin',(0.,0.,11.5));
#24045=CARTESIAN_POINT('',(-45.9910159507968,-27.3326993144394,24.2));
#24046=CARTESIAN_POINT('',(-45.9910159507968,-27.3326993144394,14.5));
#24047=CARTESIAN_POINT('Origin',(0.,0.,24.2));
#24048=CARTESIAN_POINT('Origin',(0.,0.,11.25));
#24049=CARTESIAN_POINT('',(-46.3021993580384,-25.7896555736688,11.));
#24050=CARTESIAN_POINT('Ctrl Pts',(-46.6542861332861,-25.7671839061264,
11.2969997378715));
#24051=CARTESIAN_POINT('Ctrl Pts',(-46.5344704431712,-25.7808636960853,
11.1987310576086));
#24052=CARTESIAN_POINT('Ctrl Pts',(-46.4147276669438,-25.787371326691,11.0971961933879));
#24053=CARTESIAN_POINT('Ctrl Pts',(-46.3021993580384,-25.7896555736688,
11.));
#24054=CARTESIAN_POINT('',(-45.135512297021,-27.781028233049,11.));
#24055=CARTESIAN_POINT('Origin',(0.,0.,11.));
#24056=CARTESIAN_POINT('',(-45.2340370888743,-27.7395880641857,11.0622545443403));
#24057=CARTESIAN_POINT('Ctrl Pts',(-45.2340370888743,-27.7395880641857,
11.0622545443404));
#24058=CARTESIAN_POINT('Ctrl Pts',(-45.2018816759998,-27.7503055360096,
11.0404458048696));
#24059=CARTESIAN_POINT('Ctrl Pts',(-45.1686134036895,-27.7640234893725,
11.0192759649605));
#24060=CARTESIAN_POINT('Ctrl Pts',(-45.135512297021,-27.781028233049,11.));
#24061=CARTESIAN_POINT('Ctrl Pts',(-45.9910159507968,-27.3326993144394,
11.5));
#24062=CARTESIAN_POINT('Ctrl Pts',(-45.6109717288891,-27.5369794153495,
11.2776618075202));
#24063=CARTESIAN_POINT('Ctrl Pts',(-45.2340370888743,-27.7395880641857,
11.0622545443403));
#24064=CARTESIAN_POINT('Origin',(-45.6125265198356,-27.5361436893125,14.5));
#24065=CARTESIAN_POINT('',(-45.2340370888744,-27.7395880641857,24.2));
#24066=CARTESIAN_POINT('',(-45.3706737374995,-27.6661435891479,24.2));
#24067=CARTESIAN_POINT('',(-45.2340370888744,-27.7395880641857,14.5));
#24068=CARTESIAN_POINT('Origin',(-45.4553779539844,-28.4036725628998,11.));
#24069=CARTESIAN_POINT('',(-44.7555290624911,-28.3891285237239,11.));
#24070=CARTESIAN_POINT('Origin',(-45.4553779539844,-28.4036725628998,11.));
#24071=CARTESIAN_POINT('',(-44.7614733114311,-28.4958481944022,11.0622545443403));
#24072=CARTESIAN_POINT('Ctrl Pts',(-44.7555290624911,-28.3891285237239,
11.));
#24073=CARTESIAN_POINT('Ctrl Pts',(-44.7547558702061,-28.4263339903097,
11.0192759649605));
#24074=CARTESIAN_POINT('Ctrl Pts',(-44.7570101060804,-28.4622488703402,
11.0404458048696));
#24075=CARTESIAN_POINT('Ctrl Pts',(-44.7614733114311,-28.4958481944021,
11.0622545443403));
#24076=CARTESIAN_POINT('',(-44.7614733114311,-28.4958481944023,24.2));
#24077=CARTESIAN_POINT('',(-44.7614733114311,-28.4958481944023,14.5));
#24078=CARTESIAN_POINT('Origin',(-45.4553779539844,-28.4036725628998,24.2));
#24079=CARTESIAN_POINT('Origin',(-48.3346988609778,-22.4164821240926,14.5));
#24080=CARTESIAN_POINT('',(-48.3380665247094,-22.4499778554777,11.2969997378715));
#24081=CARTESIAN_POINT('',(-48.3776844341152,-22.8440287338545,11.5));
#24082=CARTESIAN_POINT('Ctrl Pts',(-48.3380665247094,-22.4499778554777,
11.2969997378715));
#24083=CARTESIAN_POINT('Ctrl Pts',(-48.3578378264537,-22.6466287877421,
11.3977655520825));
#24084=CARTESIAN_POINT('Ctrl Pts',(-48.3776844341152,-22.8440287338545,
11.5));
#24085=CARTESIAN_POINT('',(-48.3776844341152,-22.8440287338545,24.2));
#24086=CARTESIAN_POINT('',(-48.3776844341152,-22.8440287338545,14.5));
#24087=CARTESIAN_POINT('',(-48.2917132878405,-21.9889355143307,24.2));
#24088=CARTESIAN_POINT('',(-48.3072313028027,-22.1432820590691,24.2));
#24089=CARTESIAN_POINT('',(-48.2917132878405,-21.9889355143307,11.5));
#24090=CARTESIAN_POINT('',(-48.2917132878405,-21.9889355143307,14.5));
#24091=CARTESIAN_POINT('Ctrl Pts',(-48.2917132878405,-21.9889355143307,
11.5));
#24092=CARTESIAN_POINT('Ctrl Pts',(-48.3119548726829,-22.1902640146607,
11.4654707447276));
#24093=CARTESIAN_POINT('Ctrl Pts',(-48.3380665247094,-22.4499778554777,
11.2969997378715));
#24094=CARTESIAN_POINT('Origin',(-48.9660365296434,-21.8010840688629,11.25));
#24095=CARTESIAN_POINT('',(-48.6544270396318,-21.1742670894066,11.5));
#24096=CARTESIAN_POINT('Origin',(-48.9660365296434,-21.8010840688629,11.5));
#24097=CARTESIAN_POINT('',(-49.028064639274,-20.9002167162411,11.2969997378715));
#24098=CARTESIAN_POINT('Ctrl Pts',(-49.028064639274,-20.9002167162411,11.2969997378715));
#24099=CARTESIAN_POINT('Ctrl Pts',(-48.8175875368124,-21.0545944569385,
11.4654707447276));
#24100=CARTESIAN_POINT('Ctrl Pts',(-48.6544270396318,-21.1742670894066,
11.5));
#24101=CARTESIAN_POINT('',(-48.8290062914572,-20.608933611151,11.));
#24102=CARTESIAN_POINT('Ctrl Pts',(-49.028064639274,-20.9002167162411,11.2969997378715));
#24103=CARTESIAN_POINT('Ctrl Pts',(-48.9650785563254,-20.7973785443114,
11.1987310576086));
#24104=CARTESIAN_POINT('Ctrl Pts',(-48.8964856249514,-20.699013451518,11.0971961933879));
#24105=CARTESIAN_POINT('Ctrl Pts',(-48.8290062914572,-20.608933611151,11.));
#24106=CARTESIAN_POINT('',(-47.9884049594373,-22.4969551150606,11.));
#24107=CARTESIAN_POINT('Origin',(-48.9660365296434,-21.8010840688629,11.));
#24108=CARTESIAN_POINT('Ctrl Pts',(-48.3380665247094,-22.4499778554777,
11.2969997378715));
#24109=CARTESIAN_POINT('Ctrl Pts',(-48.2194969535028,-22.4719822421975,
11.1987310576086));
#24110=CARTESIAN_POINT('Ctrl Pts',(-48.1004998140235,-22.4868268543681,
11.0971961933879));
#24111=CARTESIAN_POINT('Ctrl Pts',(-47.9884049594373,-22.4969551150606,
11.));
#24112=CARTESIAN_POINT('Origin',(-48.9660365296434,-21.8010840688629,11.));
#24113=CARTESIAN_POINT('',(-48.6544270396318,-21.1742670894066,24.2));
#24114=CARTESIAN_POINT('Origin',(-48.9660365296434,-21.8010840688629,24.2));
#24115=CARTESIAN_POINT('',(-48.6544270396318,-21.1742670894066,14.5));
#24116=CARTESIAN_POINT('Origin',(-47.4222409819887,-24.2872980186631,14.5));
#24117=CARTESIAN_POINT('',(-47.7856168695246,-24.0579471360089,24.2));
#24118=CARTESIAN_POINT('',(-47.0588650944528,-24.5166489013173,24.2));
#24119=CARTESIAN_POINT('',(-47.1900456754746,-24.4338520425372,24.2));
#24120=CARTESIAN_POINT('',(-47.7856168695246,-24.0579471360089,11.5));
#24121=CARTESIAN_POINT('',(-47.7856168695246,-24.0579471360089,14.5));
#24122=CARTESIAN_POINT('',(-47.4507093193417,-24.2693297424964,11.2969997378715));
#24123=CARTESIAN_POINT('Ctrl Pts',(-47.7856168695246,-24.0579471360089,
11.5));
#24124=CARTESIAN_POINT('Ctrl Pts',(-47.6178447974743,-24.1638393378014,
11.3977655520829));
#24125=CARTESIAN_POINT('Ctrl Pts',(-47.4507093193417,-24.2693297424964,
11.2969997378715));
#24126=CARTESIAN_POINT('',(-47.0588650944528,-24.5166489013173,11.5));
#24127=CARTESIAN_POINT('Ctrl Pts',(-47.4507093193417,-24.2693297424964,
11.2969997378715));
#24128=CARTESIAN_POINT('Ctrl Pts',(-47.2299760817075,-24.4086492863049,
11.4654707447276));
#24129=CARTESIAN_POINT('Ctrl Pts',(-47.0588650944528,-24.5166489013173,
11.5));
#24130=CARTESIAN_POINT('',(-47.0588650944528,-24.5166489013173,14.5));
#24131=CARTESIAN_POINT('Origin',(-47.3259909772385,-25.1636757653237,11.));
#24132=CARTESIAN_POINT('Origin',(-47.3259909772385,-25.1636757653237,24.2));
#24133=CARTESIAN_POINT('Origin',(-47.3259909772385,-25.1636757653237,11.5));
#24134=CARTESIAN_POINT('Origin',(-47.3259909772385,-25.1636757653237,11.25));
#24135=CARTESIAN_POINT('',(-47.2724547499278,-23.9648705799974,11.));
#24136=CARTESIAN_POINT('Ctrl Pts',(-47.4507093193417,-24.2693297424964,
11.2969997378715));
#24137=CARTESIAN_POINT('Ctrl Pts',(-47.3950502955656,-24.1623483921435,
11.1987310576087));
#24138=CARTESIAN_POINT('Ctrl Pts',(-47.3334860551377,-24.0594381107558,
11.0971961933879));
#24139=CARTESIAN_POINT('Ctrl Pts',(-47.2724547499278,-23.9648705799974,
11.));
#24140=CARTESIAN_POINT('Origin',(-47.3259909772385,-25.1636757653237,11.));
#24141=CARTESIAN_POINT('Origin',(-49.7806527105708,-18.9902185482608,14.5));
#24142=CARTESIAN_POINT('',(-49.7863487149497,-19.0233977693811,11.2969997378715));
#24143=CARTESIAN_POINT('',(-49.8533577168707,-19.4137251539658,11.5));
#24144=CARTESIAN_POINT('Ctrl Pts',(-49.7863487149497,-19.0233977693811,
11.2969997378715));
#24145=CARTESIAN_POINT('Ctrl Pts',(-49.8197895303902,-19.2181904935679,
11.3977655520829));
#24146=CARTESIAN_POINT('Ctrl Pts',(-49.8533577168707,-19.4137251539658,
11.5));
#24147=CARTESIAN_POINT('',(-49.8533577168707,-19.4137251539658,24.2));
#24148=CARTESIAN_POINT('',(-49.8533577168707,-19.4137251539658,14.5));
#24149=CARTESIAN_POINT('',(-49.707947704271,-18.5667119425558,24.2));
#24150=CARTESIAN_POINT('',(-49.7341945888243,-18.7196000248653,24.2));
#24151=CARTESIAN_POINT('',(-49.707947704271,-18.5667119425558,11.5));
#24152=CARTESIAN_POINT('',(-49.707947704271,-18.5667119425558,14.5));
#24153=CARTESIAN_POINT('Ctrl Pts',(-49.707947704271,-18.5667119425558,11.5));
#24154=CARTESIAN_POINT('Ctrl Pts',(-49.7421839478772,-18.7661380351961,
11.4654707447276));
#24155=CARTESIAN_POINT('Ctrl Pts',(-49.7863487149497,-19.0233977693811,
11.2969997378715));
#24156=CARTESIAN_POINT('Origin',(-50.3675244741247,-18.3322796822558,11.25));
#24157=CARTESIAN_POINT('',(-50.0129495069995,-17.7287263766662,11.5));
#24158=CARTESIAN_POINT('Origin',(-50.3675244741247,-18.3322796822558,11.5));
#24159=CARTESIAN_POINT('',(-50.3665601565676,-17.4292799350267,11.2969997378715));
#24160=CARTESIAN_POINT('Ctrl Pts',(-50.3665601565676,-17.4292799350267,
11.2969997378715));
#24161=CARTESIAN_POINT('Ctrl Pts',(-50.1673646125647,-17.5979637597785,
11.4654707447276));
#24162=CARTESIAN_POINT('Ctrl Pts',(-50.0129495069995,-17.7287263766662,
11.5));
#24163=CARTESIAN_POINT('',(-50.1476678226092,-17.1525919893539,11.));
#24164=CARTESIAN_POINT('Ctrl Pts',(-50.3665601565676,-17.4292799350267,
11.2969997378715));
#24165=CARTESIAN_POINT('Ctrl Pts',(-50.2965538763113,-17.3310859587567,
11.1987310576086));
#24166=CARTESIAN_POINT('Ctrl Pts',(-50.221266431858,-17.237745279402,11.0971961933879));
#24167=CARTESIAN_POINT('Ctrl Pts',(-50.1476678226092,-17.1525919893539,
11.));
#24168=CARTESIAN_POINT('',(-49.4408158756514,-19.0946517525179,11.));
#24169=CARTESIAN_POINT('Origin',(-50.3675244741247,-18.3322796822558,11.));
#24170=CARTESIAN_POINT('Ctrl Pts',(-49.7863487149497,-19.0233977693811,
11.2969997378715));
#24171=CARTESIAN_POINT('Ctrl Pts',(-49.6696029216838,-19.0536195497014,
11.1987310576086));
#24172=CARTESIAN_POINT('Ctrl Pts',(-49.5519311610546,-19.0767288219785,
11.0971961933879));
#24173=CARTESIAN_POINT('Ctrl Pts',(-49.4408158756514,-19.0946517525179,
11.));
#24174=CARTESIAN_POINT('Origin',(-50.3675244741247,-18.3322796822558,11.));
#24175=CARTESIAN_POINT('',(-50.0129495069995,-17.7287263766662,24.2));
#24176=CARTESIAN_POINT('Origin',(-50.3675244741247,-18.3322796822558,24.2));
#24177=CARTESIAN_POINT('',(-50.0129495069995,-17.7287263766662,14.5));
#24178=CARTESIAN_POINT('Origin',(-49.0009190529448,-20.9201270734172,14.5));
#24179=CARTESIAN_POINT('',(-49.3474110662579,-20.6659870574277,24.2));
#24180=CARTESIAN_POINT('',(-48.7795124544456,-21.0825212248573,24.2));
#24181=CARTESIAN_POINT('',(-49.3474110662579,-20.6659870574277,11.5));
#24182=CARTESIAN_POINT('',(-49.3474110662579,-20.6659870574277,14.5));
#24183=CARTESIAN_POINT('Ctrl Pts',(-49.3474110662579,-20.6659870574277,
11.5));
#24184=CARTESIAN_POINT('Ctrl Pts',(-49.1874343451363,-20.7833244992782,
11.3977655520826));
#24185=CARTESIAN_POINT('Ctrl Pts',(-49.028064639274,-20.9002167162411,11.2969997378715));
#24186=CARTESIAN_POINT('Origin',(-50.34086957183,-17.4510353719535,14.5));
#24187=CARTESIAN_POINT('',(-50.6687896366606,-17.1733443672407,24.2));
#24188=CARTESIAN_POINT('',(-50.131330352038,-17.6284784829776,24.2));
#24189=CARTESIAN_POINT('',(-50.6687896366606,-17.1733443672407,11.5));
#24190=CARTESIAN_POINT('',(-50.6687896366606,-17.1733443672407,14.5));
#24191=CARTESIAN_POINT('Ctrl Pts',(-50.6687896366606,-17.1733443672407,
11.5));
#24192=CARTESIAN_POINT('Ctrl Pts',(-50.5173876569737,-17.3015553929261,
11.3977655520831));
#24193=CARTESIAN_POINT('Ctrl Pts',(-50.3665601565676,-17.4292799350267,
11.2969997378715));
#24194=CARTESIAN_POINT('Origin',(-52.6411144591754,8.22525703532524,14.5));
#24195=CARTESIAN_POINT('',(-52.8002826611136,8.62439278479967,24.2));
#24196=CARTESIAN_POINT('',(-52.4819462572371,7.8261212858508,24.2));
#24197=CARTESIAN_POINT('',(-52.5394068040886,7.97021136259658,24.2));
#24198=CARTESIAN_POINT('',(-52.8002826611136,8.62439278479967,11.5));
#24199=CARTESIAN_POINT('',(-52.8002826611136,8.62439278479967,14.5));
#24200=CARTESIAN_POINT('',(-52.4819462572371,7.82612128585067,11.0622545443402));
#24201=CARTESIAN_POINT('Ctrl Pts',(-52.8002826611136,8.62439278479967,11.5));
#24202=CARTESIAN_POINT('Ctrl Pts',(-52.6404606145519,8.22361743168168,11.2776618075197));
#24203=CARTESIAN_POINT('Ctrl Pts',(-52.4819462572371,7.82612128585067,11.0622545443402));
#24204=CARTESIAN_POINT('',(-52.4819462572371,7.8261212858508,14.5));
#24205=CARTESIAN_POINT('Origin',(-53.0783684845482,7.4596782114595,11.));
#24206=CARTESIAN_POINT('',(-52.4331091150171,7.73104575932093,11.));
#24207=CARTESIAN_POINT('Ctrl Pts',(-52.481946257237,7.82612128585063,11.0622545443403));
#24208=CARTESIAN_POINT('Ctrl Pts',(-52.4642028399839,7.79724212513569,11.0404458048696));
#24209=CARTESIAN_POINT('Ctrl Pts',(-52.4475355953004,7.76534912995433,11.0192759649605));
#24210=CARTESIAN_POINT('Ctrl Pts',(-52.4331091150171,7.73104575932093,11.));
#24211=CARTESIAN_POINT('',(-52.5329044020197,7.0209653957459,11.));
#24212=CARTESIAN_POINT('Origin',(-53.0783684845482,7.4596782114595,11.));
#24213=CARTESIAN_POINT('',(-52.6060560429105,6.94303427461877,11.0622545443404));
#24214=CARTESIAN_POINT('Ctrl Pts',(-52.6060560429105,6.94303427461877,11.0622545443404));
#24215=CARTESIAN_POINT('Ctrl Pts',(-52.5810436316806,6.96590045416114,11.0404491452186));
#24216=CARTESIAN_POINT('Ctrl Pts',(-52.5562282907997,6.99196614352735,11.0192767711931));
#24217=CARTESIAN_POINT('Ctrl Pts',(-52.5329044020197,7.02096539574591,11.));
#24218=CARTESIAN_POINT('',(-52.6060560429105,6.94303427461877,24.2));
#24219=CARTESIAN_POINT('',(-52.6060560429105,6.94303427461877,14.5));
#24220=CARTESIAN_POINT('Origin',(-53.0783684845482,7.4596782114595,24.2));
#24221=CARTESIAN_POINT('Origin',(0.,0.,11.25));
#24222=CARTESIAN_POINT('',(-52.5657520484127,9.95448198475441,11.5));
#24223=CARTESIAN_POINT('Origin',(0.,0.,11.5));
#24224=CARTESIAN_POINT('',(-51.9935887462791,10.5957343592208,11.0622545443404));
#24225=CARTESIAN_POINT('Ctrl Pts',(-52.5657520484127,9.95448198475441,11.5));
#24226=CARTESIAN_POINT('Ctrl Pts',(-52.3754957821832,10.1677118127105,11.3527407245743));
#24227=CARTESIAN_POINT('Ctrl Pts',(-52.184766529217,10.3814717408442,11.2067970124645));
#24228=CARTESIAN_POINT('Ctrl Pts',(-51.9935887462791,10.5957343592208,11.0622545443404));
#24229=CARTESIAN_POINT('',(-51.9151790989041,10.6683728435365,11.));
#24230=CARTESIAN_POINT('Ctrl Pts',(-51.9935887462791,10.5957343592208,11.0622545443404));
#24231=CARTESIAN_POINT('Ctrl Pts',(-51.9670422000274,10.6168000602485,11.0404491452634));
#24232=CARTESIAN_POINT('Ctrl Pts',(-51.940469057341,10.6410712243803,11.0192767711182));
#24233=CARTESIAN_POINT('Ctrl Pts',(-51.9151790989041,10.6683728435365,11.));
#24234=CARTESIAN_POINT('Origin',(0.,0.,11.));
#24235=CARTESIAN_POINT('Origin',(-51.4355644344077,13.8969239803297,14.5));
#24236=CARTESIAN_POINT('',(-51.4596748556074,13.8734294539541,11.2969997378715));
#24237=CARTESIAN_POINT('',(-51.7433149571623,13.5970348695554,11.5));
#24238=CARTESIAN_POINT('Ctrl Pts',(-51.4596748556074,13.8734294539541,11.2969997378715));
#24239=CARTESIAN_POINT('Ctrl Pts',(-51.6012253341346,13.7354948478477,11.3977655520825));
#24240=CARTESIAN_POINT('Ctrl Pts',(-51.7433149571623,13.5970348695554,11.5));
#24241=CARTESIAN_POINT('',(-51.7433149571623,13.5970348695554,24.2));
#24242=CARTESIAN_POINT('',(-51.7433149571623,13.5970348695554,14.5));
#24243=CARTESIAN_POINT('',(-51.1278139116531,14.1968130911041,24.2));
#24244=CARTESIAN_POINT('',(-51.238913447339,14.0885515659373,24.2));
#24245=CARTESIAN_POINT('',(-51.1278139116531,14.1968130911041,11.5));
#24246=CARTESIAN_POINT('',(-51.1278139116531,14.1968130911041,14.5));
#24247=CARTESIAN_POINT('Ctrl Pts',(-51.1278139116531,14.1968130911041,11.5));
#24248=CARTESIAN_POINT('Ctrl Pts',(-51.2727313307305,14.055597552122,11.4654707447276));
#24249=CARTESIAN_POINT('Ctrl Pts',(-51.4596748556074,13.8734294539541,11.2969997378715));
#24250=CARTESIAN_POINT('Origin',(0.,0.,14.5));
#24251=CARTESIAN_POINT('',(-52.0700565974321,12.286545728569,11.5));
#24252=CARTESIAN_POINT('Origin',(0.,0.,11.5));
#24253=CARTESIAN_POINT('',(-52.0700565974321,12.286545728569,24.2));
#24254=CARTESIAN_POINT('',(-52.0700565974321,12.286545728569,14.5));
#24255=CARTESIAN_POINT('Origin',(0.,0.,24.2));
#24256=CARTESIAN_POINT('Origin',(0.,0.,11.25));
#24257=CARTESIAN_POINT('',(-51.2220149569553,13.6126846635571,11.));
#24258=CARTESIAN_POINT('Ctrl Pts',(-51.4596748556074,13.8734294539541,11.2969997378715));
#24259=CARTESIAN_POINT('Ctrl Pts',(-51.3829894416038,13.7803580645257,11.1987310576087));
#24260=CARTESIAN_POINT('Ctrl Pts',(-51.3013742769325,13.6924965450168,11.0971961933879));
#24261=CARTESIAN_POINT('Ctrl Pts',(-51.2220149569553,13.6126846635571,11.));
#24262=CARTESIAN_POINT('',(-51.766094205967,11.3697621197168,11.));
#24263=CARTESIAN_POINT('Origin',(0.,0.,11.));
#24264=CARTESIAN_POINT('',(-51.8081802498931,11.4680127538716,11.0622545443405));
#24265=CARTESIAN_POINT('Ctrl Pts',(-51.766094205967,11.3697621197168,11.));
#24266=CARTESIAN_POINT('Ctrl Pts',(-51.7780925319007,11.4049878878031,11.0192757561174));
#24267=CARTESIAN_POINT('Ctrl Pts',(-51.7924947217674,11.4379665269991,11.0404460254343));
#24268=CARTESIAN_POINT('Ctrl Pts',(-51.8081802498931,11.4680127538716,11.0622545443405));
#24269=CARTESIAN_POINT('Ctrl Pts',(-52.0700565974321,12.286545728569,11.5));
#24270=CARTESIAN_POINT('Ctrl Pts',(-51.9829772340571,12.0143663927566,11.352740724575));
#24271=CARTESIAN_POINT('Ctrl Pts',(-51.8956813869632,11.7415104052956,11.2067970124648));
#24272=CARTESIAN_POINT('Ctrl Pts',(-51.8081802498931,11.4680127538716,11.0622545443405));
#24273=CARTESIAN_POINT('Origin',(-50.9840802240917,15.4714365365517,14.5));
#24274=CARTESIAN_POINT('',(-51.0861504520718,15.8888398565875,24.2));
#24275=CARTESIAN_POINT('',(-50.8820099961117,15.054033216516,24.2));
#24276=CARTESIAN_POINT('',(-50.9188578780728,15.204717981028,24.2));
#24277=CARTESIAN_POINT('',(-51.0861504520718,15.8888398565875,11.5));
#24278=CARTESIAN_POINT('',(-51.0861504520718,15.8888398565875,14.5));
#24279=CARTESIAN_POINT('',(-50.9920768187572,15.5041376015772,11.2969997378715));
#24280=CARTESIAN_POINT('Ctrl Pts',(-51.0861504520718,15.8888398565875,11.5));
#24281=CARTESIAN_POINT('Ctrl Pts',(-51.0390242276022,15.6961231071135,11.3977655520829));
#24282=CARTESIAN_POINT('Ctrl Pts',(-50.9920768187572,15.5041376015772,11.2969997378715));
#24283=CARTESIAN_POINT('',(-50.8820099961117,15.054033216516,11.5));
#24284=CARTESIAN_POINT('Ctrl Pts',(-50.9920768187572,15.5041376015772,11.2969997378715));
#24285=CARTESIAN_POINT('Ctrl Pts',(-50.9300741029444,15.2505853175896,11.4654707447276));
#24286=CARTESIAN_POINT('Ctrl Pts',(-50.8820099961117,15.054033216516,11.5));
#24287=CARTESIAN_POINT('',(-50.8820099961117,15.054033216516,14.5));
#24288=CARTESIAN_POINT('Origin',(0.,0.,11.25));
#24289=CARTESIAN_POINT('',(-50.6687896366605,17.173344367241,11.5));
#24290=CARTESIAN_POINT('Origin',(0.,0.,11.5));
#24291=CARTESIAN_POINT('',(-50.3665601565677,17.4292799350268,11.2969997378715));
#24292=CARTESIAN_POINT('Ctrl Pts',(-50.3665601565677,17.4292799350268,11.2969997378715));
#24293=CARTESIAN_POINT('Ctrl Pts',(-50.5173876569729,17.301555392927,11.3977655520826));
#24294=CARTESIAN_POINT('Ctrl Pts',(-50.6687896366605,17.173344367241,11.5));
#24295=CARTESIAN_POINT('',(-50.1476678226092,17.1525919893539,11.));
#24296=CARTESIAN_POINT('Ctrl Pts',(-50.3665601565677,17.4292799350268,11.2969997378715));
#24297=CARTESIAN_POINT('Ctrl Pts',(-50.2965538763113,17.3310859587568,11.1987310576087));
#24298=CARTESIAN_POINT('Ctrl Pts',(-50.221266431858,17.237745279402,11.0971961933879));
#24299=CARTESIAN_POINT('Ctrl Pts',(-50.1476678226092,17.1525919893539,11.));
#24300=CARTESIAN_POINT('',(-50.6523561066928,15.5993211660246,11.));
#24301=CARTESIAN_POINT('Origin',(0.,0.,11.));
#24302=CARTESIAN_POINT('Ctrl Pts',(-50.9920768187572,15.5041376015772,11.2969997378715));
#24303=CARTESIAN_POINT('Ctrl Pts',(-50.8777235772014,15.5424295380224,11.1987310576087));
#24304=CARTESIAN_POINT('Ctrl Pts',(-50.7619504804118,15.5736908843544,11.0971961933879));
#24305=CARTESIAN_POINT('Ctrl Pts',(-50.6523561066928,15.5993211660246,11.));
#24306=CARTESIAN_POINT('Origin',(0.,0.,14.5));
#24307=CARTESIAN_POINT('',(-50.6687896366605,17.173344367241,24.2));
#24308=CARTESIAN_POINT('Origin',(0.,0.,24.2));
#24309=CARTESIAN_POINT('',(-50.6687896366605,17.173344367241,14.5));
#24310=CARTESIAN_POINT('Origin',(-50.3408695718299,17.4510353719536,14.5));
#24311=CARTESIAN_POINT('',(-50.0129495069994,17.7287263766663,24.2));
#24312=CARTESIAN_POINT('',(-50.131330352038,17.6284784829776,24.2));
#24313=CARTESIAN_POINT('',(-50.0129495069994,17.7287263766663,11.5));
#24314=CARTESIAN_POINT('',(-50.0129495069994,17.7287263766663,14.5));
#24315=CARTESIAN_POINT('Ctrl Pts',(-50.0129495069994,17.7287263766663,11.5));
#24316=CARTESIAN_POINT('Ctrl Pts',(-50.1673646125647,17.5979637597785,11.4654707447276));
#24317=CARTESIAN_POINT('Ctrl Pts',(-50.3665601565677,17.4292799350268,11.2969997378715));
#24318=CARTESIAN_POINT('Origin',(-49.7806527105709,18.9902185482606,14.5));
#24319=CARTESIAN_POINT('',(-49.8533577168709,19.4137251539655,24.2));
#24320=CARTESIAN_POINT('',(-49.7079477042709,18.5667119425557,24.2));
#24321=CARTESIAN_POINT('',(-49.7341945888243,18.7196000248653,24.2));
#24322=CARTESIAN_POINT('',(-49.8533577168709,19.4137251539655,11.5));
#24323=CARTESIAN_POINT('',(-49.8533577168709,19.4137251539655,14.5));
#24324=CARTESIAN_POINT('',(-49.7863487149498,19.0233977693811,11.2969997378715));
#24325=CARTESIAN_POINT('Ctrl Pts',(-49.8533577168709,19.4137251539655,11.5));
#24326=CARTESIAN_POINT('Ctrl Pts',(-49.8197895303904,19.2181904935684,11.3977655520833));
#24327=CARTESIAN_POINT('Ctrl Pts',(-49.7863487149498,19.0233977693811,11.2969997378715));
#24328=CARTESIAN_POINT('',(-49.7079477042709,18.5667119425557,11.5));
#24329=CARTESIAN_POINT('Ctrl Pts',(-49.7863487149498,19.0233977693811,11.2969997378715));
#24330=CARTESIAN_POINT('Ctrl Pts',(-49.7421839478773,18.7661380351961,11.4654707447276));
#24331=CARTESIAN_POINT('Ctrl Pts',(-49.7079477042709,18.5667119425557,11.5));
#24332=CARTESIAN_POINT('',(-49.7079477042709,18.5667119425557,14.5));
#24333=CARTESIAN_POINT('Origin',(0.,0.,11.25));
#24334=CARTESIAN_POINT('',(-49.3474110662579,20.6659870574277,11.5));
#24335=CARTESIAN_POINT('Origin',(0.,0.,11.5));
#24336=CARTESIAN_POINT('',(-49.028064639274,20.9002167162411,11.2969997378715));
#24337=CARTESIAN_POINT('Ctrl Pts',(-49.028064639274,20.9002167162411,11.2969997378715));
#24338=CARTESIAN_POINT('Ctrl Pts',(-49.1874343451368,20.7833244992778,11.3977655520829));
#24339=CARTESIAN_POINT('Ctrl Pts',(-49.3474110662579,20.6659870574277,11.5));
#24340=CARTESIAN_POINT('',(-48.8290062914572,20.608933611151,11.));
#24341=CARTESIAN_POINT('Ctrl Pts',(-49.028064639274,20.9002167162411,11.2969997378715));
#24342=CARTESIAN_POINT('Ctrl Pts',(-48.9650785563254,20.7973785443115,11.1987310576086));
#24343=CARTESIAN_POINT('Ctrl Pts',(-48.8964856249514,20.699013451518,11.0971961933879));
#24344=CARTESIAN_POINT('Ctrl Pts',(-48.8290062914572,20.608933611151,11.));
#24345=CARTESIAN_POINT('',(-49.4408158756514,19.0946517525179,11.));
#24346=CARTESIAN_POINT('Origin',(0.,0.,11.));
#24347=CARTESIAN_POINT('Ctrl Pts',(-49.7863487149498,19.0233977693811,11.2969997378715));
#24348=CARTESIAN_POINT('Ctrl Pts',(-49.6696029216838,19.0536195497014,11.1987310576087));
#24349=CARTESIAN_POINT('Ctrl Pts',(-49.5519311610546,19.0767288219785,11.0971961933879));
#24350=CARTESIAN_POINT('Ctrl Pts',(-49.4408158756514,19.0946517525179,11.));
#24351=CARTESIAN_POINT('Origin',(0.,0.,14.5));
#24352=CARTESIAN_POINT('',(-49.3474110662579,20.6659870574277,24.2));
#24353=CARTESIAN_POINT('Origin',(0.,0.,24.2));
#24354=CARTESIAN_POINT('',(-49.3474110662579,20.6659870574277,14.5));
#24355=CARTESIAN_POINT('Origin',(-49.0009190529448,20.9201270734172,14.5));
#24356=CARTESIAN_POINT('',(-48.6544270396318,21.1742670894066,24.2));
#24357=CARTESIAN_POINT('',(-48.7795124544456,21.0825212248573,24.2));
#24358=CARTESIAN_POINT('',(-48.6544270396318,21.1742670894066,11.5));
#24359=CARTESIAN_POINT('',(-48.6544270396318,21.1742670894066,14.5));
#24360=CARTESIAN_POINT('Ctrl Pts',(-48.6544270396318,21.1742670894066,11.5));
#24361=CARTESIAN_POINT('Ctrl Pts',(-48.8175875368124,21.0545944569386,11.4654707447276));
#24362=CARTESIAN_POINT('Ctrl Pts',(-49.028064639274,20.9002167162411,11.2969997378715));
#24363=CARTESIAN_POINT('Origin',(-48.3346988609778,22.4164821240926,14.5));
#24364=CARTESIAN_POINT('',(-48.3776844341152,22.8440287338545,24.2));
#24365=CARTESIAN_POINT('',(-48.2917132878404,21.9889355143307,24.2));
#24366=CARTESIAN_POINT('',(-48.3072313028027,22.1432820590691,24.2));
#24367=CARTESIAN_POINT('',(-48.3776844341152,22.8440287338545,11.5));
#24368=CARTESIAN_POINT('',(-48.3776844341152,22.8440287338545,14.5));
#24369=CARTESIAN_POINT('',(-48.3380665247094,22.4499778554778,11.2969997378715));
#24370=CARTESIAN_POINT('Ctrl Pts',(-48.3776844341152,22.8440287338545,11.5));
#24371=CARTESIAN_POINT('Ctrl Pts',(-48.3578378264537,22.6466287877423,11.3977655520826));
#24372=CARTESIAN_POINT('Ctrl Pts',(-48.3380665247094,22.4499778554778,11.2969997378715));
#24373=CARTESIAN_POINT('',(-48.2917132878404,21.9889355143307,11.5));
#24374=CARTESIAN_POINT('Ctrl Pts',(-48.3380665247094,22.4499778554778,11.2969997378715));
#24375=CARTESIAN_POINT('Ctrl Pts',(-48.3119548726828,22.1902640146608,11.4654707447276));
#24376=CARTESIAN_POINT('Ctrl Pts',(-48.2917132878404,21.9889355143307,11.5));
#24377=CARTESIAN_POINT('',(-48.2917132878404,21.9889355143307,14.5));
#24378=CARTESIAN_POINT('Origin',(0.,0.,11.25));
#24379=CARTESIAN_POINT('',(-47.7856168695246,24.0579471360089,11.5));
#24380=CARTESIAN_POINT('Origin',(0.,0.,11.5));
#24381=CARTESIAN_POINT('',(-47.4507093193417,24.2693297424964,11.2969997378715));
#24382=CARTESIAN_POINT('Ctrl Pts',(-47.4507093193417,24.2693297424964,11.2969997378715));
#24383=CARTESIAN_POINT('Ctrl Pts',(-47.6178447974735,24.1638393378019,11.3977655520824));
#24384=CARTESIAN_POINT('Ctrl Pts',(-47.7856168695246,24.0579471360089,11.5));
#24385=CARTESIAN_POINT('',(-47.2724547499278,23.9648705799974,11.));
#24386=CARTESIAN_POINT('Ctrl Pts',(-47.4507093193417,24.2693297424964,11.2969997378715));
#24387=CARTESIAN_POINT('Ctrl Pts',(-47.3950502955656,24.1623483921435,11.1987310576087));
#24388=CARTESIAN_POINT('Ctrl Pts',(-47.3334860551377,24.0594381107558,11.0971961933879));
#24389=CARTESIAN_POINT('Ctrl Pts',(-47.2724547499278,23.9648705799974,11.));
#24390=CARTESIAN_POINT('',(-47.9884049594373,22.4969551150606,11.));
#24391=CARTESIAN_POINT('Origin',(0.,0.,11.));
#24392=CARTESIAN_POINT('Ctrl Pts',(-48.3380665247094,22.4499778554778,11.2969997378715));
#24393=CARTESIAN_POINT('Ctrl Pts',(-48.2194969535028,22.4719822421975,11.1987310576086));
#24394=CARTESIAN_POINT('Ctrl Pts',(-48.1004998140235,22.4868268543681,11.0971961933879));
#24395=CARTESIAN_POINT('Ctrl Pts',(-47.9884049594373,22.4969551150606,11.));
#24396=CARTESIAN_POINT('Origin',(0.,0.,14.5));
#24397=CARTESIAN_POINT('',(-47.7856168695246,24.0579471360089,24.2));
#24398=CARTESIAN_POINT('Origin',(0.,0.,24.2));
#24399=CARTESIAN_POINT('',(-47.7856168695246,24.0579471360089,14.5));
#24400=CARTESIAN_POINT('Origin',(-47.4222409819887,24.2872980186631,14.5));
#24401=CARTESIAN_POINT('',(-47.0588650944528,24.5166489013173,24.2));
#24402=CARTESIAN_POINT('',(-47.1900456754746,24.4338520425371,24.2));
#24403=CARTESIAN_POINT('',(-47.0588650944528,24.5166489013173,11.5));
#24404=CARTESIAN_POINT('',(-47.0588650944528,24.5166489013173,14.5));
#24405=CARTESIAN_POINT('Ctrl Pts',(-47.0588650944528,24.5166489013173,11.5));
#24406=CARTESIAN_POINT('Ctrl Pts',(-47.2299760817074,24.4086492863049,11.4654707447276));
#24407=CARTESIAN_POINT('Ctrl Pts',(-47.4507093193417,24.2693297424964,11.2969997378715));
#24408=CARTESIAN_POINT('Origin',(-46.653263217121,25.7335348523128,14.5));
#24409=CARTESIAN_POINT('',(-46.6663199357044,26.1630385020256,24.2));
#24410=CARTESIAN_POINT('',(-46.6402064985376,25.3040312025999,24.2));
#24411=CARTESIAN_POINT('',(-46.6449200416998,25.459084248916,24.2));
#24412=CARTESIAN_POINT('',(-46.6663199357044,26.1630385020256,11.5));
#24413=CARTESIAN_POINT('',(-46.6663199357044,26.1630385020257,14.5));
#24414=CARTESIAN_POINT('',(-46.6542861332861,25.7671839061264,11.2969997378715));
#24415=CARTESIAN_POINT('Ctrl Pts',(-46.6663199357044,26.1630385020256,11.5));
#24416=CARTESIAN_POINT('Ctrl Pts',(-46.6602915975399,25.9647349828969,11.3977655520838));
#24417=CARTESIAN_POINT('Ctrl Pts',(-46.6542861332861,25.7671839061264,11.2969997378715));
#24418=CARTESIAN_POINT('',(-46.6402064985376,25.3040312025999,11.5));
#24419=CARTESIAN_POINT('Ctrl Pts',(-46.6542861332861,25.7671839061264,11.2969997378715));
#24420=CARTESIAN_POINT('Ctrl Pts',(-46.6463548096495,25.5062812584035,11.4654707447276));
#24421=CARTESIAN_POINT('Ctrl Pts',(-46.6402064985376,25.3040312025999,11.5));
#24422=CARTESIAN_POINT('',(-46.6402064985376,25.3040312025999,14.5));
#24423=CARTESIAN_POINT('Origin',(0.,0.,11.25));
#24424=CARTESIAN_POINT('',(-45.9910159507968,27.3326993144394,11.5));
#24425=CARTESIAN_POINT('Origin',(0.,0.,11.5));
#24426=CARTESIAN_POINT('',(-45.6421789133341,27.5202050337906,11.2969997378715));
#24427=CARTESIAN_POINT('Ctrl Pts',(-45.6421789133341,27.5202050337906,11.2969997378715));
#24428=CARTESIAN_POINT('Ctrl Pts',(-45.8162658964882,27.4266303800113,11.3977655520832));
#24429=CARTESIAN_POINT('Ctrl Pts',(-45.9910159507968,27.3326993144394,11.5));
#24430=CARTESIAN_POINT('',(-45.4855965606673,27.2040531083184,11.));
#24431=CARTESIAN_POINT('Ctrl Pts',(-45.6421789133341,27.5202050337906,11.2969997378715));
#24432=CARTESIAN_POINT('Ctrl Pts',(-45.5941181138995,27.4096017073997,11.1987310576086));
#24433=CARTESIAN_POINT('Ctrl Pts',(-45.5398824992087,27.3026476059643,11.0971961933879));
#24434=CARTESIAN_POINT('Ctrl Pts',(-45.4855965606673,27.2040531083184,11.));
#24435=CARTESIAN_POINT('',(-46.3021993580384,25.7896555736688,11.));
#24436=CARTESIAN_POINT('Origin',(0.,0.,11.));
#24437=CARTESIAN_POINT('Ctrl Pts',(-46.6542861332861,25.7671839061264,11.2969997378715));
#24438=CARTESIAN_POINT('Ctrl Pts',(-46.5344704431712,25.7808636960853,11.1987310576086));
#24439=CARTESIAN_POINT('Ctrl Pts',(-46.4147276669438,25.787371326691,11.0971961933879));
#24440=CARTESIAN_POINT('Ctrl Pts',(-46.3021993580384,25.7896555736688,11.));
#24441=CARTESIAN_POINT('Origin',(0.,0.,14.5));
#24442=CARTESIAN_POINT('',(-45.9910159507968,27.3326993144394,24.2));
#24443=CARTESIAN_POINT('Origin',(0.,0.,24.2));
#24444=CARTESIAN_POINT('',(-45.9910159507968,27.3326993144394,14.5));
#24445=CARTESIAN_POINT('Origin',(-45.6125265198356,27.5361436893125,14.5));
#24446=CARTESIAN_POINT('',(-45.2340370888744,27.7395880641857,24.2));
#24447=CARTESIAN_POINT('',(-45.3706737374995,27.6661435891479,24.2));
#24448=CARTESIAN_POINT('',(-45.2340370888744,27.7395880641857,11.5));
#24449=CARTESIAN_POINT('',(-45.2340370888744,27.7395880641857,14.5));
#24450=CARTESIAN_POINT('Ctrl Pts',(-45.2340370888744,27.7395880641857,11.5));
#24451=CARTESIAN_POINT('Ctrl Pts',(-45.412264930673,27.6437876298971,11.4654707447275));
#24452=CARTESIAN_POINT('Ctrl Pts',(-45.6421789133341,27.5202050337906,11.2969997378715));
#24453=CARTESIAN_POINT('Origin',(-44.74453756444,28.9252163854584,14.5));
#24454=CARTESIAN_POINT('',(-44.727601817449,29.3545845765144,24.2));
#24455=CARTESIAN_POINT('',(-44.7614733114311,28.4958481944023,24.2));
#24456=CARTESIAN_POINT('',(-44.7553594188847,28.6508523394404,24.2));
#24457=CARTESIAN_POINT('',(-44.727601817449,29.3545845765144,11.5));
#24458=CARTESIAN_POINT('',(-44.727601817449,29.3545845765144,14.5));
#24459=CARTESIAN_POINT('',(-44.7432107494939,28.9588548268927,11.2969997378715));
#24460=CARTESIAN_POINT('Ctrl Pts',(-44.727601817449,29.3545845765144,11.5));
#24461=CARTESIAN_POINT('Ctrl Pts',(-44.7354211182388,29.1563435991768,11.3977655520828));
#24462=CARTESIAN_POINT('Ctrl Pts',(-44.7432107494939,28.9588548268927,11.2969997378715));
#24463=CARTESIAN_POINT('',(-44.7614733114311,28.4958481944023,11.5));
#24464=CARTESIAN_POINT('Ctrl Pts',(-44.7432107494939,28.9588548268927,11.2969997378715));
#24465=CARTESIAN_POINT('Ctrl Pts',(-44.7534983948587,28.6980344637377,11.4654707447276));
#24466=CARTESIAN_POINT('Ctrl Pts',(-44.7614733114311,28.4958481944023,11.5));
#24467=CARTESIAN_POINT('',(-44.7614733114311,28.4958481944023,14.5));
#24468=CARTESIAN_POINT('Origin',(0.,0.,11.25));
#24469=CARTESIAN_POINT('',(-43.9723514253571,30.4742893292837,11.5));
#24470=CARTESIAN_POINT('Origin',(0.,0.,11.5));
#24471=CARTESIAN_POINT('',(-43.6112843995965,30.6370046524817,11.2969997378715));
#24472=CARTESIAN_POINT('Ctrl Pts',(-43.6112843995965,30.6370046524817,11.2969997378715));
#24473=CARTESIAN_POINT('Ctrl Pts',(-43.7914747534883,30.5558016359257,11.397765552083));
#24474=CARTESIAN_POINT('Ctrl Pts',(-43.9723514253571,30.4742893292837,11.5));
#24475=CARTESIAN_POINT('',(-43.4771371171594,30.3107002244375,11.));
#24476=CARTESIAN_POINT('Ctrl Pts',(-43.6112843995965,30.6370046524817,11.2969997378715));
#24477=CARTESIAN_POINT('Ctrl Pts',(-43.5710559718872,30.5233181983411,11.1987310576087));
#24478=CARTESIAN_POINT('Ctrl Pts',(-43.5244132133966,30.4128413464891,11.0971961933879));
#24479=CARTESIAN_POINT('Ctrl Pts',(-43.4771371171594,30.3107002244375,11.));
#24480=CARTESIAN_POINT('',(-44.390414095648,28.9567114226892,11.));
#24481=CARTESIAN_POINT('Origin',(0.,0.,11.));
#24482=CARTESIAN_POINT('Ctrl Pts',(-44.7432107494939,28.9588548268927,11.2969997378715));
#24483=CARTESIAN_POINT('Ctrl Pts',(-44.6227326704691,28.9641433735292,11.1987310576086));
#24484=CARTESIAN_POINT('Ctrl Pts',(-44.5028276322629,28.9622823180478,11.0971961933879));
#24485=CARTESIAN_POINT('Ctrl Pts',(-44.390414095648,28.9567114226892,11.));
#24486=CARTESIAN_POINT('Origin',(0.,0.,14.5));
#24487=CARTESIAN_POINT('',(-43.9723514253571,30.4742893292837,24.2));
#24488=CARTESIAN_POINT('Origin',(0.,0.,24.2));
#24489=CARTESIAN_POINT('',(-43.9723514253571,30.4742893292837,14.5));
#24490=CARTESIAN_POINT('Origin',(-43.5805924134327,30.6508360358314,14.5));
#24491=CARTESIAN_POINT('',(-43.1888334015084,30.827382742379,24.2));
#24492=CARTESIAN_POINT('',(-43.3302604377194,30.7636484651835,24.2));
#24493=CARTESIAN_POINT('',(-43.1888334015084,30.827382742379,11.5));
#24494=CARTESIAN_POINT('',(-43.1888334015084,30.827382742379,14.5));
#24495=CARTESIAN_POINT('Ctrl Pts',(-43.1888334015084,30.827382742379,11.5));
#24496=CARTESIAN_POINT('Ctrl Pts',(-43.3733097897212,30.7442482189004,11.4654707447276));
#24497=CARTESIAN_POINT('Ctrl Pts',(-43.6112843995965,30.6370046524817,11.2969997378715));
#24498=CARTESIAN_POINT('Origin',(-42.6178210224504,31.9759771719264,14.5));
#24499=CARTESIAN_POINT('',(-42.5709753191419,32.4031180656586,24.2));
#24500=CARTESIAN_POINT('',(-42.6646667257588,31.5488362781942,24.2));
#24501=CARTESIAN_POINT('',(-42.6477551837739,31.7030363573407,24.2));
#24502=CARTESIAN_POINT('',(-42.5709753191419,32.4031180656586,11.5));
#24503=CARTESIAN_POINT('',(-42.5709753191419,32.4031180656586,14.5));
#24504=CARTESIAN_POINT('',(-42.614150940502,32.0094411178763,11.2969997378715));
#24505=CARTESIAN_POINT('Ctrl Pts',(-42.5709753191419,32.4031180656586,11.5));
#24506=CARTESIAN_POINT('Ctrl Pts',(-42.5926041640386,32.2059054402286,11.3977655520829));
#24507=CARTESIAN_POINT('Ctrl Pts',(-42.614150940502,32.0094411178763,11.2969997378715));
#24508=CARTESIAN_POINT('',(-42.6646667257588,31.5488362781942,11.5));
#24509=CARTESIAN_POINT('Ctrl Pts',(-42.614150940502,32.0094411178763,11.2969997378715));
#24510=CARTESIAN_POINT('Ctrl Pts',(-42.642607434494,31.7499737298808,11.4654707447276));
#24511=CARTESIAN_POINT('Ctrl Pts',(-42.6646667257588,31.5488362781942,11.5));
#24512=CARTESIAN_POINT('',(-42.6646667257588,31.5488362781942,14.5));
#24513=CARTESIAN_POINT('Origin',(0.,0.,11.25));
#24514=CARTESIAN_POINT('',(-41.7394580238585,33.4674116697804,11.5));
#24515=CARTESIAN_POINT('Origin',(0.,0.,11.5));
#24516=CARTESIAN_POINT('',(-41.3679200920551,33.6045438641268,11.2969997378715));
#24517=CARTESIAN_POINT('Ctrl Pts',(-41.3679200920551,33.6045438641268,11.2969997378715));
#24518=CARTESIAN_POINT('Ctrl Pts',(-41.5533359473934,33.5361080977281,11.397765552083));
#24519=CARTESIAN_POINT('Ctrl Pts',(-41.7394580238585,33.4674116697804,11.5));
#24520=CARTESIAN_POINT('',(-41.2568614319233,33.2696766558841,11.));
#24521=CARTESIAN_POINT('Ctrl Pts',(-41.3679200920551,33.6045438641268,11.2969997378715));
#24522=CARTESIAN_POINT('Ctrl Pts',(-41.3357200249272,33.4883281512133,11.1987310576087));
#24523=CARTESIAN_POINT('Ctrl Pts',(-41.2968973614676,33.3748667810619,11.097196193388));
#24524=CARTESIAN_POINT('Ctrl Pts',(-41.2568614319233,33.2696766558841,11.));
#24525=CARTESIAN_POINT('',(-42.2623631978924,31.9826930843766,11.));
#24526=CARTESIAN_POINT('Origin',(0.,0.,11.));
#24527=CARTESIAN_POINT('Ctrl Pts',(-42.614150940502,32.0094411178763,11.2969997378715));
#24528=CARTESIAN_POINT('Ctrl Pts',(-42.4935974296579,32.0063126559227,11.1987310576087));
#24529=CARTESIAN_POINT('Ctrl Pts',(-42.3741142947661,31.9960919812296,11.0971961933879));
#24530=CARTESIAN_POINT('Ctrl Pts',(-42.2623631978924,31.9826930843766,11.));
#24531=CARTESIAN_POINT('Origin',(0.,0.,14.5));
#24532=CARTESIAN_POINT('',(-41.7394580238585,33.4674116697804,24.2));
#24533=CARTESIAN_POINT('Origin',(0.,0.,24.2));
#24534=CARTESIAN_POINT('',(-41.7394580238585,33.4674116697804,14.5));
#24535=CARTESIAN_POINT('Origin',(-41.3363380414976,33.6162005901948,14.5));
#24536=CARTESIAN_POINT('',(-40.9332180591366,33.7649895106092,24.2));
#24537=CARTESIAN_POINT('',(-41.0787464646293,33.7112759382477,24.2));
#24538=CARTESIAN_POINT('',(-40.9332180591366,33.7649895106092,11.5));
#24539=CARTESIAN_POINT('',(-40.9332180591366,33.7649895106092,14.5));
#24540=CARTESIAN_POINT('Ctrl Pts',(-40.9332180591366,33.7649895106092,11.5));
#24541=CARTESIAN_POINT('Ctrl Pts',(-41.1230442433438,33.6949259209822,11.4654707447276));
#24542=CARTESIAN_POINT('Ctrl Pts',(-41.3679200920551,33.6045438641268,11.2969997378715));
#24543=CARTESIAN_POINT('Origin',(-40.2834747403676,34.870954211827,14.5));
#24544=CARTESIAN_POINT('',(-40.2069473082993,35.2937868207372,24.2));
#24545=CARTESIAN_POINT('',(-40.3600021724359,34.4481216029168,24.2));
#24546=CARTESIAN_POINT('',(-40.332375372345,34.600766368886,24.2));
#24547=CARTESIAN_POINT('',(-40.2069473082993,35.2937868207372,11.5));
#24548=CARTESIAN_POINT('',(-40.2069473082993,35.2937868207372,14.5));
#24549=CARTESIAN_POINT('',(-40.2774792716874,34.9040806293114,11.2969997378715));
#24550=CARTESIAN_POINT('Ctrl Pts',(-40.2069473082993,35.2937868207372,11.5));
#24551=CARTESIAN_POINT('Ctrl Pts',(-40.2422803237447,35.098563347302,11.3977655520829));
#24552=CARTESIAN_POINT('Ctrl Pts',(-40.2774792716874,34.9040806293114,11.2969997378715));
#24553=CARTESIAN_POINT('',(-40.3600021724359,34.4481216029168,11.5));
#24554=CARTESIAN_POINT('Ctrl Pts',(-40.2774792716874,34.9040806293114,11.2969997378715));
#24555=CARTESIAN_POINT('Ctrl Pts',(-40.3239659771285,34.6472303155083,11.4654707447276));
#24556=CARTESIAN_POINT('Ctrl Pts',(-40.3600021724359,34.4481216029168,11.5));
#24557=CARTESIAN_POINT('',(-40.3600021724359,34.4481216029168,14.5));
#24558=CARTESIAN_POINT('Origin',(0.,0.,11.25));
#24559=CARTESIAN_POINT('',(-39.3032141785034,36.2974841447543,11.5));
#24560=CARTESIAN_POINT('Origin',(0.,0.,11.5));
#24561=CARTESIAN_POINT('',(-38.923015436114,36.4083651159827,11.2969997378715));
#24562=CARTESIAN_POINT('Ctrl Pts',(-38.923015436114,36.4083651159827,11.2969997378715));
#24563=CARTESIAN_POINT('Ctrl Pts',(-39.11275346549,36.353030011916,11.3977655520832));
#24564=CARTESIAN_POINT('Ctrl Pts',(-39.3032141785034,36.2974841447543,11.5));
#24565=CARTESIAN_POINT('',(-38.835586464916,36.0665665669195,11.));
#24566=CARTESIAN_POINT('Ctrl Pts',(-38.923015436114,36.4083651159827,11.2969997378715));
#24567=CARTESIAN_POINT('Ctrl Pts',(-38.8990006050577,36.2901863355677,11.1987310576087));
#24568=CARTESIAN_POINT('Ctrl Pts',(-38.868187176743,36.1742932195071,11.0971961933879));
#24569=CARTESIAN_POINT('Ctrl Pts',(-38.835586464916,36.0665665669195,11.));
#24570=CARTESIAN_POINT('',(-39.9284143148345,34.8528582802461,11.));
#24571=CARTESIAN_POINT('Origin',(0.,0.,11.));
#24572=CARTESIAN_POINT('Ctrl Pts',(-40.2774792716874,34.9040806293114,11.2969997378715));
#24573=CARTESIAN_POINT('Ctrl Pts',(-40.1574376536108,34.8925504003199,11.1987310576087));
#24574=CARTESIAN_POINT('Ctrl Pts',(-40.0389585318564,34.8740199005147,11.0971961933879));
#24575=CARTESIAN_POINT('Ctrl Pts',(-39.9284143148345,34.8528582802461,11.));
#24576=CARTESIAN_POINT('Origin',(0.,0.,14.5));
#24577=CARTESIAN_POINT('',(-39.3032141785034,36.2974841447543,24.2));
#24578=CARTESIAN_POINT('Origin',(0.,0.,24.2));
#24579=CARTESIAN_POINT('',(-39.3032141785034,36.2974841447543,14.5));
#24580=CARTESIAN_POINT('Origin',(-38.8906971857384,36.4177903943714,14.5));
#24581=CARTESIAN_POINT('',(-38.4781801929734,36.5380966439885,24.2));
#24582=CARTESIAN_POINT('',(-38.6271009679847,36.4946654635864,24.2));
#24583=CARTESIAN_POINT('',(-38.4781801929734,36.5380966439885,11.5));
#24584=CARTESIAN_POINT('',(-38.4781801929734,36.5380966439885,14.5));
#24585=CARTESIAN_POINT('Ctrl Pts',(-38.4781801929734,36.5380966439885,11.5));
#24586=CARTESIAN_POINT('Ctrl Pts',(-38.6724313590868,36.481445330979,11.4654707447276));
#24587=CARTESIAN_POINT('Ctrl Pts',(-38.923015436114,36.4083651159827,11.2969997378715));
#24588=CARTESIAN_POINT('Origin',(-37.7528714186305,37.5960434680237,14.5));
#24589=CARTESIAN_POINT('',(-37.6470350917587,38.0125077941444,24.2));
#24590=CARTESIAN_POINT('',(-37.8587077455022,37.179579141903,24.2));
#24591=CARTESIAN_POINT('',(-37.8205002822982,37.329924924739,24.2));
#24592=CARTESIAN_POINT('',(-37.6470350917587,38.0125077941444,11.5));
#24593=CARTESIAN_POINT('',(-37.6470350917587,38.0125077941444,14.5));
#24594=CARTESIAN_POINT('',(-37.7445797725392,37.6286709684663,11.2969997378715));
#24595=CARTESIAN_POINT('Ctrl Pts',(-37.6470350917587,38.0125077941444,11.5));
#24596=CARTESIAN_POINT('Ctrl Pts',(-37.6959001388532,37.8202245818431,11.397765552083));
#24597=CARTESIAN_POINT('Ctrl Pts',(-37.7445797725392,37.6286709684663,11.2969997378715));
#24598=CARTESIAN_POINT('',(-37.8587077455022,37.179579141903,11.5));
#24599=CARTESIAN_POINT('Ctrl Pts',(-37.7445797725392,37.6286709684663,11.2969997378715));
#24600=CARTESIAN_POINT('Ctrl Pts',(-37.8088702108732,37.375689077766,11.4654707447276));
#24601=CARTESIAN_POINT('Ctrl Pts',(-37.8587077455022,37.179579141903,11.5));
#24602=CARTESIAN_POINT('',(-37.8587077455022,37.179579141903,14.5));
#24603=CARTESIAN_POINT('Origin',(0.,0.,11.25));
#24604=CARTESIAN_POINT('',(-36.6754890244158,38.9507189255854,11.5));
#24605=CARTESIAN_POINT('Origin',(0.,0.,11.5));
#24606=CARTESIAN_POINT('',(-36.288481761496,39.0348084727497,11.2969997378715));
#24607=CARTESIAN_POINT('Ctrl Pts',(-36.288481761496,39.0348084727497,11.2969997378715));
#24608=CARTESIAN_POINT('Ctrl Pts',(-36.4816175803016,38.99284361808,11.3977655520827));
#24609=CARTESIAN_POINT('Ctrl Pts',(-36.6754890244158,38.9507189255854,11.5));
#24610=CARTESIAN_POINT('',(-36.2251084243911,38.6877437910394,11.));
#24611=CARTESIAN_POINT('Ctrl Pts',(-36.288481761496,39.0348084727497,11.2969997378715));
#24612=CARTESIAN_POINT('Ctrl Pts',(-36.2727691643543,38.9152423799721,11.1987310576087));
#24613=CARTESIAN_POINT('Ctrl Pts',(-36.2501150911098,38.7974821376142,11.0971961933879));
#24614=CARTESIAN_POINT('Ctrl Pts',(-36.2251084243911,38.6877437910394,11.));
#24615=CARTESIAN_POINT('',(-37.3999382108249,37.5532238539712,11.));
#24616=CARTESIAN_POINT('Origin',(0.,0.,11.));
#24617=CARTESIAN_POINT('Ctrl Pts',(-37.7445797725392,37.6286709684663,11.2969997378715));
#24618=CARTESIAN_POINT('Ctrl Pts',(-37.6256348779268,37.6087951465536,11.1987310576086));
#24619=CARTESIAN_POINT('Ctrl Pts',(-37.5087369876814,37.5820451003687,11.0971961933879));
#24620=CARTESIAN_POINT('Ctrl Pts',(-37.399938210825,37.5532238539712,11.));
#24621=CARTESIAN_POINT('Origin',(0.,0.,14.5));
#24622=CARTESIAN_POINT('',(-36.6754890244158,38.9507189255854,24.2));
#24623=CARTESIAN_POINT('Origin',(0.,0.,24.2));
#24624=CARTESIAN_POINT('',(-36.6754890244158,38.9507189255854,14.5));
#24625=CARTESIAN_POINT('Origin',(-36.2555847625695,39.0419563844502,14.5));
#24626=CARTESIAN_POINT('',(-35.8356805007232,39.1331938433149,24.2));
#24627=CARTESIAN_POINT('',(-35.9872681182067,39.1002566472175,24.2));
#24628=CARTESIAN_POINT('',(-35.8356805007232,39.1331938433149,11.5));
#24629=CARTESIAN_POINT('',(-35.8356805007232,39.1331938433149,14.5));
#24630=CARTESIAN_POINT('Ctrl Pts',(-35.8356805007232,39.1331938433149,11.5));
#24631=CARTESIAN_POINT('Ctrl Pts',(-36.0334102765874,39.0902308064254,11.4654707447276));
#24632=CARTESIAN_POINT('Ctrl Pts',(-36.288481761496,39.0348084727497,11.2969997378715));
#24633=CARTESIAN_POINT('Origin',(-35.8654005008348,39.8325626455883,11.25));
#24634=CARTESIAN_POINT('',(-35.1729694999764,39.729901508588,11.5));
#24635=CARTESIAN_POINT('Origin',(-35.8654005008348,39.8325626455883,11.5));
#24636=CARTESIAN_POINT('',(-35.027792474811,40.1699382050837,11.2969997378714));
#24637=CARTESIAN_POINT('Ctrl Pts',(-35.027792474811,40.1699382050837,11.2969997378714));
#24638=CARTESIAN_POINT('Ctrl Pts',(-35.1095734294849,39.9220572398278,11.4654707447275));
#24639=CARTESIAN_POINT('Ctrl Pts',(-35.1729694999764,39.729901508588,11.5));
#24640=CARTESIAN_POINT('',(-34.6892533672809,40.0706338959167,11.));
#24641=CARTESIAN_POINT('Ctrl Pts',(-34.6892533672809,40.0706338959167,11.));
#24642=CARTESIAN_POINT('Ctrl Pts',(-34.7645593265508,40.0963245531492,11.0687122343714));
#24643=CARTESIAN_POINT('Ctrl Pts',(-34.841627036511,40.1204761473162,11.1374591885178));
#24644=CARTESIAN_POINT('Ctrl Pts',(-34.955624113946,40.1519342014003,11.2360127801162));
#24645=CARTESIAN_POINT('Ctrl Pts',(-34.9916111096869,40.161260817967,11.2666805180049));
#24646=CARTESIAN_POINT('Ctrl Pts',(-35.027792474811,40.1699382050837,11.2969997378714));
#24647=CARTESIAN_POINT('Origin',(-35.8654005008348,39.8325626455883,11.));
#24648=CARTESIAN_POINT('Origin',(0.,0.,11.25));
#24649=CARTESIAN_POINT('Origin',(0.,0.,11.));
#24650=CARTESIAN_POINT('Origin',(0.,0.,11.5));
#24651=CARTESIAN_POINT('Origin',(0.,0.,11.25));
#24652=CARTESIAN_POINT('Origin',(0.,0.,11.));
#24653=CARTESIAN_POINT('Origin',(0.,0.,11.5));
#24654=CARTESIAN_POINT('Origin',(0.,0.,11.25));
#24655=CARTESIAN_POINT('',(-51.0861504520717,-15.8888398565878,11.5));
#24656=CARTESIAN_POINT('Origin',(0.,0.,11.5));
#24657=CARTESIAN_POINT('',(-50.8820099961117,-15.0540332165161,11.0622545443405));
#24658=CARTESIAN_POINT('Ctrl Pts',(-51.0861504520717,-15.8888398565878,
11.5));
#24659=CARTESIAN_POINT('Ctrl Pts',(-50.9836609313633,-15.4697218918374,
11.2776618075213));
#24660=CARTESIAN_POINT('Ctrl Pts',(-50.8820099961117,-15.0540332165161,
11.0622545443405));
#24661=CARTESIAN_POINT('',(-50.8468800894551,-14.9530861419499,11.));
#24662=CARTESIAN_POINT('Ctrl Pts',(-50.8468800894551,-14.9530861419499,
11.));
#24663=CARTESIAN_POINT('Ctrl Pts',(-50.8563919627033,-14.9890630627436,
11.0192757561174));
#24664=CARTESIAN_POINT('Ctrl Pts',(-50.86845859598,-15.0229660136113,11.0404460254343));
#24665=CARTESIAN_POINT('Ctrl Pts',(-50.8820099961117,-15.0540332165161,
11.0622545443405));
#24666=CARTESIAN_POINT('Origin',(0.,0.,11.));
#24667=CARTESIAN_POINT('Origin',(0.,0.,11.));
#24668=CARTESIAN_POINT('',(-51.0445282617143,-14.2638050512144,11.));
#24669=CARTESIAN_POINT('Origin',(-51.5236269022939,-14.7741622717911,11.));
#24670=CARTESIAN_POINT('',(-51.766094205967,-11.3697621197168,11.));
#24671=CARTESIAN_POINT('Origin',(0.,0.,11.));
#24672=CARTESIAN_POINT('',(-51.9151790989041,-10.6683728435365,11.));
#24673=CARTESIAN_POINT('Origin',(-52.428711399332,-11.1440666278319,11.));
#24674=CARTESIAN_POINT('',(-52.4331091150171,-7.73104575932095,11.));
#24675=CARTESIAN_POINT('Origin',(0.,0.,11.));
#24676=CARTESIAN_POINT('',(-52.5329044020197,-7.02096539574591,11.));
#24677=CARTESIAN_POINT('Origin',(-53.0783684845482,-7.45967821145951,11.));
#24678=CARTESIAN_POINT('',(-52.8446751870164,-4.05466452110769,11.));
#24679=CARTESIAN_POINT('Origin',(0.,0.,11.));
#24680=CARTESIAN_POINT('',(-52.8946946754777,-3.33935251029225,11.));
#24681=CARTESIAN_POINT('Origin',(-53.4694330939266,-3.73894699268512,11.));
#24682=CARTESIAN_POINT('',(-52.9987873134328,-0.358529364921027,11.));
#24683=CARTESIAN_POINT('Origin',(0.,0.,11.));
#24684=CARTESIAN_POINT('',(-52.9987873134328,0.35852936492104,11.));
#24685=CARTESIAN_POINT('Origin',(-53.6,6.56410684342981E-15,11.));
#24686=CARTESIAN_POINT('',(-52.8946946754776,3.33935251029228,11.));
#24687=CARTESIAN_POINT('Origin',(0.,0.,11.));
#24688=CARTESIAN_POINT('',(-52.8446751870164,4.05466452110769,11.));
#24689=CARTESIAN_POINT('Origin',(-53.4694330939266,3.73894699268513,11.));
#24690=CARTESIAN_POINT('Origin',(0.,0.,11.));
#24691=CARTESIAN_POINT('Origin',(-52.428711399332,11.1440666278319,11.));
#24692=CARTESIAN_POINT('Origin',(-51.5236269022939,14.7741622717912,11.));
#24693=CARTESIAN_POINT('Origin',(-50.3675244741247,18.3322796822559,11.));
#24694=CARTESIAN_POINT('Origin',(-48.9660365296434,21.8010840688629,11.));
#24695=CARTESIAN_POINT('Origin',(-47.3259909772385,25.1636757653237,11.));
#24696=CARTESIAN_POINT('Origin',(-45.4553779539844,28.4036725628998,11.));
#24697=CARTESIAN_POINT('Origin',(-43.3633108984972,31.5052895228766,11.));
#24698=CARTESIAN_POINT('Origin',(-41.0599821511772,34.4534158791985,11.));
#24699=CARTESIAN_POINT('Origin',(-38.5566132981517,37.2336886566023,11.));
#24700=CARTESIAN_POINT('',(-33.4381452969578,41.1204382162877,11.));
#24701=CARTESIAN_POINT('Origin',(0.,0.,11.));
#24702=CARTESIAN_POINT('',(-31.809565968283,42.3928238374073,11.));
#24703=CARTESIAN_POINT('Origin',(-32.9994550774553,42.2373763933203,11.));
#24704=CARTESIAN_POINT('',(-30.4882748868283,43.3527979999583,11.));
#24705=CARTESIAN_POINT('Origin',(0.,0.,11.));
#24706=CARTESIAN_POINT('',(-28.774905561374,44.5084802024739,11.));
#24707=CARTESIAN_POINT('Origin',(-29.972739626032,44.4364138889502,11.));
#24708=CARTESIAN_POINT('',(-27.3898686661209,45.3739473095812,11.));
#24709=CARTESIAN_POINT('Origin',(0.,0.,11.));
#24710=CARTESIAN_POINT('',(-25.6000567070134,46.4072957259707,11.));
#24711=CARTESIAN_POINT('Origin',(-26.8,46.4189616428459,11.));
#24712=CARTESIAN_POINT('',(-24.1580217584921,47.174039308885,11.));
#24713=CARTESIAN_POINT('Origin',(0.,0.,11.));
#24714=CARTESIAN_POINT('',(-22.300486949685,48.0800195695356,11.));
#24715=CARTESIAN_POINT('Origin',(-23.4966934678946,48.1753608816354,11.));
#24716=CARTESIAN_POINT('',(-20.8084793972118,48.7443041305937,11.));
#24717=CARTESIAN_POINT('Origin',(0.,0.,11.));
#24718=CARTESIAN_POINT('',(-18.8922714615747,49.5185023907445,11.));
#24719=CARTESIAN_POINT('Origin',(-20.0789134070929,49.6970546047798,11.));
#24720=CARTESIAN_POINT('',(-17.3575602159692,50.0770916023385,11.));
#24721=CARTESIAN_POINT('Origin',(0.,0.,11.));
#24722=CARTESIAN_POINT('',(-15.3920147259482,50.7157360458881,11.));
#24723=CARTESIAN_POINT('Origin',(-16.5633108984972,50.9766292734202,11.));
#24724=CARTESIAN_POINT('',(-13.8220767461304,51.1659085175284,11.));
#24725=CARTESIAN_POINT('Origin',(0.,0.,11.));
#24726=CARTESIAN_POINT('',(-11.8167696417768,51.6658877329441,11.));
#24727=CARTESIAN_POINT('Origin',(-12.9670136041422,52.0078509283934,11.));
#24728=CARTESIAN_POINT('',(-10.2192535077747,52.0054502696,11.));
#24729=CARTESIAN_POINT('Origin',(0.,0.,11.));
#24730=CARTESIAN_POINT('',(-8.18395444372813,52.3643284084021,11.));
#24731=CARTESIAN_POINT('Origin',(-9.30754232294747,52.7856955614544,11.));
#24732=CARTESIAN_POINT('',(-6.56664309356487,52.5916266955277,11.));
#24733=CARTESIAN_POINT('Origin',(0.,0.,11.));
#24734=CARTESIAN_POINT('Origin',(-5.60272563114623,53.3063735917395,11.));
#24735=CARTESIAN_POINT('',(-1.49132004456261,52.9790143785696,11.));
#24736=CARTESIAN_POINT('Origin',(-1.87061302325405,53.5673483282235,11.));
#24737=CARTESIAN_POINT('',(1.49132004456262,52.9790143785696,11.));
#24738=CARTESIAN_POINT('Origin',(0.,0.,11.));
#24739=CARTESIAN_POINT('',(2.2079419616008,52.953989389792,11.));
#24740=CARTESIAN_POINT('Origin',(1.87061302325406,53.5673483282235,11.));
#24741=CARTESIAN_POINT('',(4.51126784227787,52.8076553394982,11.));
#24742=CARTESIAN_POINT('Origin',(0.,0.,11.));
#24743=CARTESIAN_POINT('',(6.56664309356487,52.5916266955277,11.));
#24744=CARTESIAN_POINT('Origin',(5.60272563114623,53.3063735917395,11.));
#24745=CARTESIAN_POINT('',(8.18395444372813,52.3643284084021,11.));
#24746=CARTESIAN_POINT('Origin',(0.,0.,11.));
#24747=CARTESIAN_POINT('',(10.2192535077747,52.0054502696,11.));
#24748=CARTESIAN_POINT('Origin',(9.30754232294747,52.7856955614544,11.));
#24749=CARTESIAN_POINT('',(11.8167696417768,51.6658877329441,11.));
#24750=CARTESIAN_POINT('Origin',(0.,0.,11.));
#24751=CARTESIAN_POINT('',(13.8220767461304,51.1659085175284,11.));
#24752=CARTESIAN_POINT('Origin',(12.9670136041422,52.0078509283934,11.));
#24753=CARTESIAN_POINT('',(15.3920147259482,50.7157360458881,11.));
#24754=CARTESIAN_POINT('Origin',(0.,0.,11.));
#24755=CARTESIAN_POINT('',(17.3575602159693,50.0770916023385,11.));
#24756=CARTESIAN_POINT('Origin',(16.5633108984972,50.9766292734202,11.));
#24757=CARTESIAN_POINT('',(18.8922714615747,49.5185023907445,11.));
#24758=CARTESIAN_POINT('Origin',(0.,0.,11.));
#24759=CARTESIAN_POINT('',(20.8084793972118,48.7443041305937,11.));
#24760=CARTESIAN_POINT('Origin',(20.0789134070929,49.6970546047798,11.));
#24761=CARTESIAN_POINT('',(22.300486949685,48.0800195695356,11.));
#24762=CARTESIAN_POINT('Origin',(0.,0.,11.));
#24763=CARTESIAN_POINT('',(24.1580217584921,47.1740393088849,11.));
#24764=CARTESIAN_POINT('Origin',(23.4966934678946,48.1753608816354,11.));
#24765=CARTESIAN_POINT('',(25.6000567070134,46.4072957259707,11.));
#24766=CARTESIAN_POINT('Origin',(0.,0.,11.));
#24767=CARTESIAN_POINT('',(27.3898686661209,45.3739473095812,11.));
#24768=CARTESIAN_POINT('Origin',(26.8,46.4189616428459,11.));
#24769=CARTESIAN_POINT('',(28.774905561374,44.5084802024738,11.));
#24770=CARTESIAN_POINT('Origin',(0.,0.,11.));
#24771=CARTESIAN_POINT('',(30.4882748868283,43.3527979999583,11.));
#24772=CARTESIAN_POINT('Origin',(29.972739626032,44.4364138889502,11.));
#24773=CARTESIAN_POINT('',(32.3467865928173,41.9843470488554,11.));
#24774=CARTESIAN_POINT('Origin',(0.,0.,11.));
#24775=CARTESIAN_POINT('',(32.9118365829004,41.5428816133457,11.));
#24776=CARTESIAN_POINT('Origin',(32.9994550774553,42.2373763933203,11.));
#24777=CARTESIAN_POINT('',(34.6892533672809,40.0706338959167,11.));
#24778=CARTESIAN_POINT('Origin',(0.,0.,11.));
#24779=CARTESIAN_POINT('',(36.2251084243911,38.6877437910394,11.));
#24780=CARTESIAN_POINT('Origin',(35.8654005008348,39.8325626455883,11.));
#24781=CARTESIAN_POINT('',(37.8750816598377,37.0739556732301,11.));
#24782=CARTESIAN_POINT('Origin',(0.,0.,11.));
#24783=CARTESIAN_POINT('',(38.3731925086332,36.5581467896744,11.));
#24784=CARTESIAN_POINT('Origin',(38.5566132981517,37.2336886566023,11.));
#24785=CARTESIAN_POINT('',(39.9284143148345,34.8528582802461,11.));
#24786=CARTESIAN_POINT('Origin',(0.,0.,11.));
#24787=CARTESIAN_POINT('',(41.2568614319233,33.2696766558841,11.));
#24788=CARTESIAN_POINT('Origin',(41.0599821511772,34.4534158791985,11.));
#24789=CARTESIAN_POINT('',(42.2623631978924,31.9826930843766,11.));
#24790=CARTESIAN_POINT('Origin',(0.,0.,11.));
#24791=CARTESIAN_POINT('',(43.4771371171594,30.3107002244375,11.));
#24792=CARTESIAN_POINT('Origin',(43.3633108984972,31.5052895228766,11.));
#24793=CARTESIAN_POINT('',(44.390414095648,28.9567114226892,11.));
#24794=CARTESIAN_POINT('Origin',(0.,0.,11.));
#24795=CARTESIAN_POINT('',(45.4855965606673,27.2040531083184,11.));
#24796=CARTESIAN_POINT('Origin',(45.4553779539844,28.4036725628998,11.));
#24797=CARTESIAN_POINT('',(46.3021993580384,25.7896555736688,11.));
#24798=CARTESIAN_POINT('Origin',(0.,0.,11.));
#24799=CARTESIAN_POINT('',(47.2724547499278,23.9648705799974,11.));
#24800=CARTESIAN_POINT('Origin',(47.3259909772385,25.1636757653237,11.));
#24801=CARTESIAN_POINT('',(47.9884049594373,22.4969551150606,11.));
#24802=CARTESIAN_POINT('Origin',(0.,0.,11.));
#24803=CARTESIAN_POINT('',(48.8290062914572,20.608933611151,11.));
#24804=CARTESIAN_POINT('Origin',(48.9660365296434,21.8010840688629,11.));
#24805=CARTESIAN_POINT('',(49.4408158756514,19.0946517525179,11.));
#24806=CARTESIAN_POINT('Origin',(0.,0.,11.));
#24807=CARTESIAN_POINT('',(50.1476678226092,17.1525919893539,11.));
#24808=CARTESIAN_POINT('Origin',(50.3675244741247,18.3322796822558,11.));
#24809=CARTESIAN_POINT('',(50.6523561066928,15.5993211660246,11.));
#24810=CARTESIAN_POINT('Origin',(0.,0.,11.));
#24811=CARTESIAN_POINT('',(51.2220149569554,13.6126846635571,11.));
#24812=CARTESIAN_POINT('Origin',(51.5236269022939,14.7741622717912,11.));
#24813=CARTESIAN_POINT('',(51.766094205967,11.3697621197168,11.));
#24814=CARTESIAN_POINT('Origin',(0.,0.,11.));
#24815=CARTESIAN_POINT('',(51.9151790989041,10.6683728435365,11.));
#24816=CARTESIAN_POINT('Origin',(52.428711399332,11.1440666278319,11.));
#24817=CARTESIAN_POINT('',(52.3304167585326,8.39806417445676,11.));
#24818=CARTESIAN_POINT('Origin',(0.,0.,11.));
#24819=CARTESIAN_POINT('',(52.6180453654948,6.35148029318636,11.));
#24820=CARTESIAN_POINT('Origin',(53.0783684845482,7.45967821145951,11.));
#24821=CARTESIAN_POINT('',(52.7887618365133,4.7272215695773,11.));
#24822=CARTESIAN_POINT('Origin',(0.,0.,11.));
#24823=CARTESIAN_POINT('',(52.9329273198661,2.66555910641112,11.));
#24824=CARTESIAN_POINT('Origin',(53.4694330939266,3.73894699268512,11.));
#24825=CARTESIAN_POINT('',(52.9987873134328,0.358529364921033,11.));
#24826=CARTESIAN_POINT('Origin',(0.,0.,11.));
#24827=CARTESIAN_POINT('',(52.9987873134328,-0.358529364921033,11.));
#24828=CARTESIAN_POINT('Origin',(53.6,0.,11.));
#24829=CARTESIAN_POINT('',(52.9329273198661,-2.66555910641113,11.));
#24830=CARTESIAN_POINT('Origin',(0.,0.,11.));
#24831=CARTESIAN_POINT('',(52.7887618365133,-4.72722156957733,11.));
#24832=CARTESIAN_POINT('Origin',(53.4694330939266,-3.73894699268513,11.));
#24833=CARTESIAN_POINT('',(52.6180453654948,-6.35148029318637,11.));
#24834=CARTESIAN_POINT('Origin',(0.,0.,11.));
#24835=CARTESIAN_POINT('',(52.3304167585326,-8.39806417445679,11.));
#24836=CARTESIAN_POINT('Origin',(53.0783684845482,-7.45967821145953,11.));
#24837=CARTESIAN_POINT('',(52.0468135832501,-10.0064577064218,11.));
#24838=CARTESIAN_POINT('Origin',(0.,0.,11.));
#24839=CARTESIAN_POINT('',(51.6171231503394,-12.0279922548487,11.));
#24840=CARTESIAN_POINT('Origin',(52.428711399332,-11.1440666278319,11.));
#24841=CARTESIAN_POINT('',(51.2220149569554,-13.6126846635571,11.));
#24842=CARTESIAN_POINT('Origin',(0.,0.,11.));
#24843=CARTESIAN_POINT('',(50.6523561066928,-15.5993211660246,11.));
#24844=CARTESIAN_POINT('Origin',(51.5236269022939,-14.7741622717911,11.));
#24845=CARTESIAN_POINT('',(50.1476678226092,-17.1525919893539,11.));
#24846=CARTESIAN_POINT('Origin',(0.,0.,11.));
#24847=CARTESIAN_POINT('',(49.4408158756514,-19.0946517525179,11.));
#24848=CARTESIAN_POINT('Origin',(50.3675244741247,-18.3322796822558,11.));
#24849=CARTESIAN_POINT('',(48.8290062914572,-20.608933611151,11.));
#24850=CARTESIAN_POINT('Origin',(0.,0.,11.));
#24851=CARTESIAN_POINT('',(47.9884049594373,-22.4969551150606,11.));
#24852=CARTESIAN_POINT('Origin',(48.9660365296434,-21.8010840688629,11.));
#24853=CARTESIAN_POINT('',(46.9634710240919,-24.5648608660681,11.));
#24854=CARTESIAN_POINT('Origin',(0.,0.,11.));
#24855=CARTESIAN_POINT('',(46.6268323415836,-25.1979861455206,11.));
#24856=CARTESIAN_POINT('Origin',(47.3259909772385,-25.1636757653237,11.));
#24857=CARTESIAN_POINT('',(45.4855965606673,-27.2040531083184,11.));
#24858=CARTESIAN_POINT('Origin',(0.,0.,11.));
#24859=CARTESIAN_POINT('',(44.390414095648,-28.9567114226892,11.));
#24860=CARTESIAN_POINT('Origin',(45.4553779539844,-28.4036725628998,11.));
#24861=CARTESIAN_POINT('',(43.4771371171594,-30.3107002244375,11.));
#24862=CARTESIAN_POINT('Origin',(0.,0.,11.));
#24863=CARTESIAN_POINT('',(42.2623631978924,-31.9826930843766,11.));
#24864=CARTESIAN_POINT('Origin',(43.3633108984972,-31.5052895228766,11.));
#24865=CARTESIAN_POINT('',(41.2568614319233,-33.2696766558841,11.));
#24866=CARTESIAN_POINT('Origin',(0.,0.,11.));
#24867=CARTESIAN_POINT('',(39.9284143148345,-34.8528582802461,11.));
#24868=CARTESIAN_POINT('Origin',(41.0599821511772,-34.4534158791985,11.));
#24869=CARTESIAN_POINT('',(38.3731925086332,-36.5581467896744,11.));
#24870=CARTESIAN_POINT('Origin',(0.,0.,11.));
#24871=CARTESIAN_POINT('',(37.8750816598376,-37.0739556732301,11.));
#24872=CARTESIAN_POINT('Origin',(38.5566132981517,-37.2336886566023,11.));
#24873=CARTESIAN_POINT('',(36.2251084243911,-38.6877437910394,11.));
#24874=CARTESIAN_POINT('Origin',(0.,0.,11.));
#24875=CARTESIAN_POINT('',(34.6892533672809,-40.0706338959167,11.));
#24876=CARTESIAN_POINT('Origin',(35.8654005008348,-39.8325626455884,11.));
#24877=CARTESIAN_POINT('',(33.4381452969578,-41.1204382162877,11.));
#24878=CARTESIAN_POINT('Origin',(0.,0.,11.));
#24879=CARTESIAN_POINT('',(31.809565968283,-42.3928238374073,11.));
#24880=CARTESIAN_POINT('Origin',(32.9994550774553,-42.2373763933203,11.));
#24881=CARTESIAN_POINT('',(30.4882748868283,-43.3527979999583,11.));
#24882=CARTESIAN_POINT('Origin',(0.,0.,11.));
#24883=CARTESIAN_POINT('',(28.774905561374,-44.5084802024738,11.));
#24884=CARTESIAN_POINT('Origin',(29.972739626032,-44.4364138889502,11.));
#24885=CARTESIAN_POINT('',(27.3898686661209,-45.3739473095812,11.));
#24886=CARTESIAN_POINT('Origin',(0.,0.,11.));
#24887=CARTESIAN_POINT('',(25.6000567070134,-46.4072957259707,11.));
#24888=CARTESIAN_POINT('Origin',(26.8,-46.4189616428459,11.));
#24889=CARTESIAN_POINT('',(24.1580217584921,-47.174039308885,11.));
#24890=CARTESIAN_POINT('Origin',(0.,0.,11.));
#24891=CARTESIAN_POINT('',(22.300486949685,-48.0800195695357,11.));
#24892=CARTESIAN_POINT('Origin',(23.4966934678945,-48.1753608816354,11.));
#24893=CARTESIAN_POINT('',(20.1861178092024,-49.0053124446014,11.));
#24894=CARTESIAN_POINT('Origin',(0.,0.,11.));
#24895=CARTESIAN_POINT('',(19.5212725321166,-49.2739273726667,11.));
#24896=CARTESIAN_POINT('Origin',(20.0789134070929,-49.6970546047798,11.));
#24897=CARTESIAN_POINT('',(17.3575602159692,-50.0770916023385,11.));
#24898=CARTESIAN_POINT('Origin',(0.,0.,11.));
#24899=CARTESIAN_POINT('',(15.3920147259482,-50.7157360458881,11.));
#24900=CARTESIAN_POINT('Origin',(16.5633108984972,-50.9766292734202,11.));
#24901=CARTESIAN_POINT('',(13.8220767461304,-51.1659085175284,11.));
#24902=CARTESIAN_POINT('Origin',(0.,0.,11.));
#24903=CARTESIAN_POINT('',(11.8167696417768,-51.6658877329441,11.));
#24904=CARTESIAN_POINT('Origin',(12.9670136041422,-52.0078509283934,11.));
#24905=CARTESIAN_POINT('',(10.2192535077747,-52.0054502696,11.));
#24906=CARTESIAN_POINT('Origin',(0.,0.,11.));
#24907=CARTESIAN_POINT('',(8.18395444372811,-52.3643284084021,11.));
#24908=CARTESIAN_POINT('Origin',(9.30754232294745,-52.7856955614544,11.));
#24909=CARTESIAN_POINT('',(6.56664309356483,-52.5916266955277,11.));
#24910=CARTESIAN_POINT('Origin',(0.,0.,11.));
#24911=CARTESIAN_POINT('',(4.51126784227785,-52.8076553394982,11.));
#24912=CARTESIAN_POINT('Origin',(5.6027256311462,-53.3063735917395,11.));
#24913=CARTESIAN_POINT('',(2.2079419616008,-52.953989389792,11.));
#24914=CARTESIAN_POINT('Origin',(0.,0.,11.));
#24915=CARTESIAN_POINT('',(1.49132004456263,-52.9790143785696,11.));
#24916=CARTESIAN_POINT('Origin',(1.87061302325407,-53.5673483282235,11.));
#24917=CARTESIAN_POINT('',(-0.816602797371066,-52.9937086819872,11.));
#24918=CARTESIAN_POINT('Origin',(0.,0.,11.));
#24919=CARTESIAN_POINT('',(-2.88204065427986,-52.9215820026866,11.));
#24920=CARTESIAN_POINT('Origin',(-1.87061302325404,-53.5673483282235,11.));
#24921=CARTESIAN_POINT('',(-4.51126784227786,-52.8076553394982,11.));
#24922=CARTESIAN_POINT('Origin',(0.,0.,11.));
#24923=CARTESIAN_POINT('',(-6.56664309356486,-52.5916266955277,11.));
#24924=CARTESIAN_POINT('Origin',(-5.60272563114622,-53.3063735917395,11.));
#24925=CARTESIAN_POINT('',(-8.18395444372813,-52.3643284084021,11.));
#24926=CARTESIAN_POINT('Origin',(0.,0.,11.));
#24927=CARTESIAN_POINT('',(-10.2192535077747,-52.0054502696,11.));
#24928=CARTESIAN_POINT('Origin',(-9.30754232294747,-52.7856955614544,11.));
#24929=CARTESIAN_POINT('',(-11.8167696417768,-51.6658877329441,11.));
#24930=CARTESIAN_POINT('Origin',(0.,0.,11.));
#24931=CARTESIAN_POINT('',(-13.8220767461304,-51.1659085175284,11.));
#24932=CARTESIAN_POINT('Origin',(-12.9670136041422,-52.0078509283934,11.));
#24933=CARTESIAN_POINT('',(-16.0365442723228,-50.5156336969243,11.));
#24934=CARTESIAN_POINT('Origin',(0.,0.,11.));
#24935=CARTESIAN_POINT('',(-16.7185076499055,-50.2940503634382,11.));
#24936=CARTESIAN_POINT('Origin',(-16.5633108984972,-50.9766292734202,11.));
#24937=CARTESIAN_POINT('',(-18.8922714615747,-49.5185023907445,11.));
#24938=CARTESIAN_POINT('Origin',(0.,0.,11.));
#24939=CARTESIAN_POINT('',(-20.8084793972118,-48.7443041305937,11.));
#24940=CARTESIAN_POINT('Origin',(-20.0789134070929,-49.6970546047798,11.));
#24941=CARTESIAN_POINT('',(-22.300486949685,-48.0800195695356,11.));
#24942=CARTESIAN_POINT('Origin',(0.,0.,11.));
#24943=CARTESIAN_POINT('',(-24.1580217584921,-47.1740393088849,11.));
#24944=CARTESIAN_POINT('Origin',(-23.4966934678946,-48.1753608816353,11.));
#24945=CARTESIAN_POINT('',(-25.6000567070134,-46.4072957259707,11.));
#24946=CARTESIAN_POINT('Origin',(0.,0.,11.));
#24947=CARTESIAN_POINT('',(-27.3898686661209,-45.3739473095812,11.));
#24948=CARTESIAN_POINT('Origin',(-26.8,-46.4189616428459,11.));
#24949=CARTESIAN_POINT('',(-28.774905561374,-44.5084802024739,11.));
#24950=CARTESIAN_POINT('Origin',(0.,0.,11.));
#24951=CARTESIAN_POINT('',(-30.4882748868283,-43.3527979999583,11.));
#24952=CARTESIAN_POINT('Origin',(-29.972739626032,-44.4364138889502,11.));
#24953=CARTESIAN_POINT('',(-31.809565968283,-42.3928238374073,11.));
#24954=CARTESIAN_POINT('Origin',(0.,0.,11.));
#24955=CARTESIAN_POINT('',(-33.4381452969578,-41.1204382162877,11.));
#24956=CARTESIAN_POINT('Origin',(-32.9994550774553,-42.2373763933203,11.));
#24957=CARTESIAN_POINT('',(-35.1966714489987,-39.6256775199017,11.));
#24958=CARTESIAN_POINT('Origin',(0.,0.,11.));
#24959=CARTESIAN_POINT('',(-35.7295499336443,-39.1458715772075,11.));
#24960=CARTESIAN_POINT('Origin',(-35.8654005008348,-39.8325626455883,11.));
#24961=CARTESIAN_POINT('',(-37.3999382108249,-37.5532238539713,11.));
#24962=CARTESIAN_POINT('Origin',(0.,0.,11.));
#24963=CARTESIAN_POINT('',(-38.835586464916,-36.0665665669195,11.));
#24964=CARTESIAN_POINT('Origin',(-38.5566132981517,-37.2336886566023,11.));
#24965=CARTESIAN_POINT('',(-39.9284143148345,-34.8528582802461,11.));
#24966=CARTESIAN_POINT('Origin',(0.,0.,11.));
#24967=CARTESIAN_POINT('',(-41.2568614319233,-33.2696766558841,11.));
#24968=CARTESIAN_POINT('Origin',(-41.0599821511772,-34.4534158791985,11.));
#24969=CARTESIAN_POINT('',(-42.2623631978924,-31.9826930843766,11.));
#24970=CARTESIAN_POINT('Origin',(0.,0.,11.));
#24971=CARTESIAN_POINT('',(-43.4771371171594,-30.3107002244375,11.));
#24972=CARTESIAN_POINT('Origin',(-43.3633108984972,-31.5052895228766,11.));
#24973=CARTESIAN_POINT('Origin',(0.,0.,11.));
#24974=CARTESIAN_POINT('',(-50.,6.12323399573677E-15,11.));
#24975=CARTESIAN_POINT('Origin',(0.,0.,11.));
#24976=CARTESIAN_POINT('Origin',(-51.5236269022939,-14.7741622717911,11.));
#24977=CARTESIAN_POINT('',(-50.8820099961117,-15.0540332165161,24.2));
#24978=CARTESIAN_POINT('',(-50.8820099961117,-15.0540332165161,14.5));
#24979=CARTESIAN_POINT('',(-51.1278139116532,-14.196813091104,24.2));
#24980=CARTESIAN_POINT('Origin',(-51.5236269022939,-14.7741622717911,24.2));
#24981=CARTESIAN_POINT('',(-51.1278139116532,-14.196813091104,11.0622545443405));
#24982=CARTESIAN_POINT('',(-51.1278139116532,-14.196813091104,14.5));
#24983=CARTESIAN_POINT('Ctrl Pts',(-51.0445282617143,-14.2638050512144,
11.));
#24984=CARTESIAN_POINT('Ctrl Pts',(-51.0716596511096,-14.2383354169029,
11.0192757561174));
#24985=CARTESIAN_POINT('Ctrl Pts',(-51.0998585632662,-14.2159784253933,
11.0404460254343));
#24986=CARTESIAN_POINT('Ctrl Pts',(-51.1278139116532,-14.196813091104,11.0622545443405));
#24987=CARTESIAN_POINT('Origin',(-50.9840802240917,-15.4714365365519,14.5));
#24988=CARTESIAN_POINT('',(-51.0861504520717,-15.8888398565878,24.2));
#24989=CARTESIAN_POINT('',(-51.0861504520717,-15.8888398565878,14.5));
#24990=CARTESIAN_POINT('',(-50.9188578780728,-15.204717981028,24.2));
#24991=CARTESIAN_POINT('Origin',(-37.7528714186306,-37.5960434680236,14.5));
#24992=CARTESIAN_POINT('',(-37.7445797725392,-37.6286709684663,11.2969997378715));
#24993=CARTESIAN_POINT('',(-37.6470350917589,-38.0125077941442,11.5));
#24994=CARTESIAN_POINT('Ctrl Pts',(-37.7445797725392,-37.6286709684663,
11.2969997378715));
#24995=CARTESIAN_POINT('Ctrl Pts',(-37.6959001388536,-37.8202245818423,
11.3977655520827));
#24996=CARTESIAN_POINT('Ctrl Pts',(-37.6470350917589,-38.0125077941442,
11.5));
#24997=CARTESIAN_POINT('',(-37.6470350917589,-38.0125077941442,24.2));
#24998=CARTESIAN_POINT('',(-37.6470350917589,-38.0125077941442,14.5));
#24999=CARTESIAN_POINT('',(-37.8587077455022,-37.179579141903,24.2));
#25000=CARTESIAN_POINT('',(-37.8205002822983,-37.329924924739,24.2));
#25001=CARTESIAN_POINT('',(-37.8587077455022,-37.179579141903,11.5));
#25002=CARTESIAN_POINT('',(-37.8587077455022,-37.179579141903,14.5));
#25003=CARTESIAN_POINT('Ctrl Pts',(-37.8587077455022,-37.179579141903,11.5));
#25004=CARTESIAN_POINT('Ctrl Pts',(-37.8088702108732,-37.3756890777659,
11.4654707447276));
#25005=CARTESIAN_POINT('Ctrl Pts',(-37.7445797725392,-37.6286709684663,
11.2969997378715));
#25006=CARTESIAN_POINT('Origin',(-38.5566132981517,-37.2336886566023,11.25));
#25007=CARTESIAN_POINT('',(-38.4781801929734,-36.5380966439885,11.5));
#25008=CARTESIAN_POINT('Origin',(-38.5566132981517,-37.2336886566023,11.5));
#25009=CARTESIAN_POINT('',(-38.923015436114,-36.4083651159828,11.2969997378716));
#25010=CARTESIAN_POINT('Ctrl Pts',(-38.923015436114,-36.4083651159828,11.2969997378716));
#25011=CARTESIAN_POINT('Ctrl Pts',(-38.6724313590868,-36.4814453309791,
11.4654707447277));
#25012=CARTESIAN_POINT('Ctrl Pts',(-38.4781801929734,-36.5380966439885,
11.5));
#25013=CARTESIAN_POINT('Ctrl Pts',(-38.923015436114,-36.4083651159828,11.2969997378716));
#25014=CARTESIAN_POINT('Ctrl Pts',(-38.8990006050577,-36.2901863355678,
11.1987310576087));
#25015=CARTESIAN_POINT('Ctrl Pts',(-38.868187176743,-36.1742932195071,11.0971961933879));
#25016=CARTESIAN_POINT('Ctrl Pts',(-38.835586464916,-36.0665665669195,11.));
#25017=CARTESIAN_POINT('Ctrl Pts',(-37.7445797725392,-37.6286709684663,
11.2969997378715));
#25018=CARTESIAN_POINT('Ctrl Pts',(-37.6256348779269,-37.6087951465537,
11.1987310576087));
#25019=CARTESIAN_POINT('Ctrl Pts',(-37.5087369876815,-37.5820451003687,
11.0971961933879));
#25020=CARTESIAN_POINT('Ctrl Pts',(-37.399938210825,-37.5532238539713,11.));
#25021=CARTESIAN_POINT('Origin',(-38.5566132981517,-37.2336886566023,11.));
#25022=CARTESIAN_POINT('',(-38.4781801929734,-36.5380966439885,24.2));
#25023=CARTESIAN_POINT('Origin',(-38.5566132981517,-37.2336886566023,24.2));
#25024=CARTESIAN_POINT('',(-38.4781801929734,-36.5380966439885,14.5));
#25025=CARTESIAN_POINT('Origin',(-38.8906971857383,-36.4177903943715,14.5));
#25026=CARTESIAN_POINT('',(-39.3032141785032,-36.2974841447544,24.2));
#25027=CARTESIAN_POINT('',(-38.6271009679847,-36.4946654635865,24.2));
#25028=CARTESIAN_POINT('',(-39.3032141785032,-36.2974841447544,11.5));
#25029=CARTESIAN_POINT('',(-39.3032141785032,-36.2974841447545,14.5));
#25030=CARTESIAN_POINT('Ctrl Pts',(-39.3032141785032,-36.2974841447544,
11.5));
#25031=CARTESIAN_POINT('Ctrl Pts',(-39.1127534654889,-36.3530300119163,
11.3977655520827));
#25032=CARTESIAN_POINT('Ctrl Pts',(-38.923015436114,-36.4083651159828,11.2969997378716));
#25033=CARTESIAN_POINT('Origin',(-40.2834747403675,-34.8709542118271,14.5));
#25034=CARTESIAN_POINT('',(-40.2774792716873,-34.9040806293113,11.2969997378715));
#25035=CARTESIAN_POINT('',(-40.2069473082991,-35.2937868207374,11.5));
#25036=CARTESIAN_POINT('Ctrl Pts',(-40.2774792716873,-34.9040806293113,
11.2969997378715));
#25037=CARTESIAN_POINT('Ctrl Pts',(-40.2422803237447,-35.0985633473019,
11.3977655520827));
#25038=CARTESIAN_POINT('Ctrl Pts',(-40.2069473082991,-35.2937868207374,
11.5));
#25039=CARTESIAN_POINT('',(-40.2069473082991,-35.2937868207374,24.2));
#25040=CARTESIAN_POINT('',(-40.2069473082991,-35.2937868207374,14.5));
#25041=CARTESIAN_POINT('',(-40.3600021724359,-34.4481216029168,24.2));
#25042=CARTESIAN_POINT('',(-40.332375372345,-34.600766368886,24.2));
#25043=CARTESIAN_POINT('',(-40.3600021724359,-34.4481216029168,11.5));
#25044=CARTESIAN_POINT('',(-40.3600021724359,-34.4481216029168,14.5));
#25045=CARTESIAN_POINT('Ctrl Pts',(-40.3600021724359,-34.4481216029168,
11.5));
#25046=CARTESIAN_POINT('Ctrl Pts',(-40.3239659771285,-34.6472303155083,
11.4654707447276));
#25047=CARTESIAN_POINT('Ctrl Pts',(-40.2774792716873,-34.9040806293113,
11.2969997378715));
#25048=CARTESIAN_POINT('Origin',(-41.0599821511772,-34.4534158791985,11.25));
#25049=CARTESIAN_POINT('',(-40.9332180591367,-33.7649895106091,11.5));
#25050=CARTESIAN_POINT('Origin',(-41.0599821511772,-34.4534158791985,11.5));
#25051=CARTESIAN_POINT('',(-41.3679200920551,-33.6045438641267,11.2969997378715));
#25052=CARTESIAN_POINT('Ctrl Pts',(-41.3679200920551,-33.6045438641267,
11.2969997378715));
#25053=CARTESIAN_POINT('Ctrl Pts',(-41.1230442433439,-33.6949259209821,
11.4654707447276));
#25054=CARTESIAN_POINT('Ctrl Pts',(-40.9332180591367,-33.7649895106091,
11.5));
#25055=CARTESIAN_POINT('Ctrl Pts',(-41.3679200920551,-33.6045438641267,
11.2969997378715));
#25056=CARTESIAN_POINT('Ctrl Pts',(-41.3357200249272,-33.4883281512132,
11.1987310576086));
#25057=CARTESIAN_POINT('Ctrl Pts',(-41.2968973614675,-33.3748667810618,
11.0971961933879));
#25058=CARTESIAN_POINT('Ctrl Pts',(-41.2568614319233,-33.2696766558841,
11.));
#25059=CARTESIAN_POINT('Ctrl Pts',(-40.2774792716873,-34.9040806293113,
11.2969997378715));
#25060=CARTESIAN_POINT('Ctrl Pts',(-40.1574376536108,-34.8925504003199,
11.1987310576086));
#25061=CARTESIAN_POINT('Ctrl Pts',(-40.0389585318563,-34.8740199005147,
11.0971961933879));
#25062=CARTESIAN_POINT('Ctrl Pts',(-39.9284143148345,-34.8528582802461,
11.));
#25063=CARTESIAN_POINT('Origin',(-41.0599821511772,-34.4534158791985,11.));
#25064=CARTESIAN_POINT('',(-40.9332180591367,-33.7649895106091,24.2));
#25065=CARTESIAN_POINT('Origin',(-41.0599821511772,-34.4534158791985,24.2));
#25066=CARTESIAN_POINT('',(-40.9332180591367,-33.7649895106091,14.5));
#25067=CARTESIAN_POINT('Origin',(-41.3363380414977,-33.6162005901946,14.5));
#25068=CARTESIAN_POINT('',(-41.7394580238587,-33.4674116697801,24.2));
#25069=CARTESIAN_POINT('',(-41.0787464646293,-33.7112759382477,24.2));
#25070=CARTESIAN_POINT('',(-41.7394580238587,-33.4674116697801,11.5));
#25071=CARTESIAN_POINT('',(-41.7394580238587,-33.4674116697801,14.5));
#25072=CARTESIAN_POINT('Ctrl Pts',(-41.7394580238587,-33.4674116697801,
11.5));
#25073=CARTESIAN_POINT('Ctrl Pts',(-41.5533359473925,-33.5361080977283,
11.3977655520824));
#25074=CARTESIAN_POINT('Ctrl Pts',(-41.3679200920551,-33.6045438641267,
11.2969997378715));
#25075=CARTESIAN_POINT('Origin',(-42.6178210224503,-31.9759771719266,14.5));
#25076=CARTESIAN_POINT('',(-42.6141509405019,-32.0094411178763,11.2969997378715));
#25077=CARTESIAN_POINT('',(-42.5709753191418,-32.4031180656588,11.5));
#25078=CARTESIAN_POINT('Ctrl Pts',(-42.6141509405019,-32.0094411178763,
11.2969997378715));
#25079=CARTESIAN_POINT('Ctrl Pts',(-42.5926041640386,-32.2059054402279,
11.3977655520824));
#25080=CARTESIAN_POINT('Ctrl Pts',(-42.5709753191418,-32.4031180656588,
11.5));
#25081=CARTESIAN_POINT('',(-42.5709753191418,-32.4031180656588,24.2));
#25082=CARTESIAN_POINT('',(-42.5709753191418,-32.4031180656588,14.5));
#25083=CARTESIAN_POINT('',(-42.6646667257588,-31.5488362781943,24.2));
#25084=CARTESIAN_POINT('',(-42.6477551837739,-31.7030363573407,24.2));
#25085=CARTESIAN_POINT('',(-42.6646667257588,-31.5488362781943,11.5));
#25086=CARTESIAN_POINT('',(-42.6646667257588,-31.5488362781943,14.5));
#25087=CARTESIAN_POINT('Ctrl Pts',(-42.6646667257588,-31.5488362781943,
11.5));
#25088=CARTESIAN_POINT('Ctrl Pts',(-42.642607434494,-31.7499737298808,11.4654707447276));
#25089=CARTESIAN_POINT('Ctrl Pts',(-42.6141509405019,-32.0094411178763,
11.2969997378715));
#25090=CARTESIAN_POINT('Origin',(-43.3633108984972,-31.5052895228766,11.25));
#25091=CARTESIAN_POINT('',(-43.1888334015084,-30.827382742379,11.5));
#25092=CARTESIAN_POINT('Origin',(-43.3633108984972,-31.5052895228766,11.5));
#25093=CARTESIAN_POINT('',(-43.6112843995965,-30.6370046524817,11.2969997378715));
#25094=CARTESIAN_POINT('Ctrl Pts',(-43.6112843995965,-30.6370046524817,
11.2969997378715));
#25095=CARTESIAN_POINT('Ctrl Pts',(-43.3733097897213,-30.7442482189004,
11.4654707447276));
#25096=CARTESIAN_POINT('Ctrl Pts',(-43.1888334015084,-30.827382742379,11.5));
#25097=CARTESIAN_POINT('Ctrl Pts',(-43.6112843995965,-30.6370046524817,
11.2969997378715));
#25098=CARTESIAN_POINT('Ctrl Pts',(-43.5710559718872,-30.523318198341,11.1987310576087));
#25099=CARTESIAN_POINT('Ctrl Pts',(-43.5244132133966,-30.412841346489,11.0971961933879));
#25100=CARTESIAN_POINT('Ctrl Pts',(-43.4771371171594,-30.3107002244375,
11.));
#25101=CARTESIAN_POINT('Ctrl Pts',(-42.6141509405019,-32.0094411178763,
11.2969997378715));
#25102=CARTESIAN_POINT('Ctrl Pts',(-42.4935974296578,-32.0063126559227,
11.1987310576086));
#25103=CARTESIAN_POINT('Ctrl Pts',(-42.3741142947661,-31.9960919812296,
11.0971961933879));
#25104=CARTESIAN_POINT('Ctrl Pts',(-42.2623631978924,-31.9826930843766,
11.));
#25105=CARTESIAN_POINT('Origin',(-43.3633108984972,-31.5052895228766,11.));
#25106=CARTESIAN_POINT('',(-43.1888334015084,-30.827382742379,24.2));
#25107=CARTESIAN_POINT('Origin',(-43.3633108984972,-31.5052895228766,24.2));
#25108=CARTESIAN_POINT('',(-43.1888334015084,-30.827382742379,14.5));
#25109=CARTESIAN_POINT('Origin',(-44.74453756444,-28.9252163854583,14.5));
#25110=CARTESIAN_POINT('',(-44.727601817449,-29.3545845765143,11.5));
#25111=CARTESIAN_POINT('Ctrl Pts',(-44.7614733114311,-28.4958481944022,
11.0622545443403));
#25112=CARTESIAN_POINT('Ctrl Pts',(-44.744607134536,-28.9234525904335,11.2776618075214));
#25113=CARTESIAN_POINT('Ctrl Pts',(-44.727601817449,-29.3545845765143,11.5));
#25114=CARTESIAN_POINT('',(-44.727601817449,-29.3545845765143,24.2));
#25115=CARTESIAN_POINT('',(-44.727601817449,-29.3545845765143,14.5));
#25116=CARTESIAN_POINT('',(-44.7553594188848,-28.6508523394404,24.2));
#25117=CARTESIAN_POINT('Origin',(0.,0.,14.5));
#25118=CARTESIAN_POINT('',(-43.9723514253571,-30.4742893292837,11.5));
#25119=CARTESIAN_POINT('Origin',(0.,0.,11.5));
#25120=CARTESIAN_POINT('',(-43.9723514253571,-30.4742893292837,24.2));
#25121=CARTESIAN_POINT('',(-43.9723514253571,-30.4742893292837,14.5));
#25122=CARTESIAN_POINT('Origin',(0.,0.,24.2));
#25123=CARTESIAN_POINT('Origin',(0.,0.,11.25));
#25124=CARTESIAN_POINT('Ctrl Pts',(-43.9723514253571,-30.4742893292837,
11.5));
#25125=CARTESIAN_POINT('Ctrl Pts',(-43.7914747534877,-30.555801635926,11.3977655520827));
#25126=CARTESIAN_POINT('Ctrl Pts',(-43.6112843995965,-30.6370046524817,
11.2969997378715));
#25127=CARTESIAN_POINT('Origin',(-43.5805924134327,-30.6508360358314,14.5));
#25128=CARTESIAN_POINT('',(-43.3302604377194,-30.7636484651835,24.2));
#25129=CARTESIAN_POINT('Origin',(-17.2413304950988,-50.4130767515726,14.5));
#25130=CARTESIAN_POINT('',(-17.6620417438948,-50.5005176353364,24.2));
#25131=CARTESIAN_POINT('',(-16.8206192463028,-50.3256358678088,24.2));
#25132=CARTESIAN_POINT('',(-16.9724981902626,-50.3572024805936,24.2));
#25133=CARTESIAN_POINT('',(-17.6620417438948,-50.5005176353364,11.5));
#25134=CARTESIAN_POINT('',(-17.6620417438948,-50.5005176353364,14.5));
#25135=CARTESIAN_POINT('',(-16.8206192463027,-50.3256358678088,11.0622545443403));
#25136=CARTESIAN_POINT('Ctrl Pts',(-17.6620417438948,-50.5005176353364,
11.5));
#25137=CARTESIAN_POINT('Ctrl Pts',(-17.2396022617919,-50.412717554503,11.27766180752));
#25138=CARTESIAN_POINT('Ctrl Pts',(-16.8206192463027,-50.3256358678088,
11.0622545443403));
#25139=CARTESIAN_POINT('',(-16.8206192463028,-50.3256358678088,14.5));
#25140=CARTESIAN_POINT('Origin',(0.,0.,11.25));
#25141=CARTESIAN_POINT('',(-18.9311980867048,-50.0385825039234,11.5));
#25142=CARTESIAN_POINT('Origin',(0.,0.,11.5));
#25143=CARTESIAN_POINT('',(-19.1764300887141,-49.7276051113597,11.2969997378715));
#25144=CARTESIAN_POINT('Ctrl Pts',(-19.1764300887141,-49.7276051113597,
11.2969997378715));
#25145=CARTESIAN_POINT('Ctrl Pts',(-19.0540471568067,-49.8827982539636,
11.3977655520831));
#25146=CARTESIAN_POINT('Ctrl Pts',(-18.9311980867048,-50.0385825039234,
11.5));
#25147=CARTESIAN_POINT('Ctrl Pts',(-19.1764300887141,-49.7276051113597,
11.2969997378715));
#25148=CARTESIAN_POINT('Ctrl Pts',(-19.0758527456145,-49.6610683973889,
11.1987310576087));
#25149=CARTESIAN_POINT('Ctrl Pts',(-18.9799414329601,-49.5890843587438,
11.0971961933879));
#25150=CARTESIAN_POINT('Ctrl Pts',(-18.8922714615747,-49.5185023907445,
11.));
#25151=CARTESIAN_POINT('Ctrl Pts',(-16.8206192463027,-50.3256358678088,
11.0622545443403));
#25152=CARTESIAN_POINT('Ctrl Pts',(-16.7890977128585,-50.3131768265636,
11.0404458048696));
#25153=CARTESIAN_POINT('Ctrl Pts',(-16.7547950072711,-50.3023009552715,
11.0192759649605));
#25154=CARTESIAN_POINT('Ctrl Pts',(-16.7185076499055,-50.2940503634382,
11.));
#25155=CARTESIAN_POINT('Origin',(0.,0.,14.5));
#25156=CARTESIAN_POINT('',(-18.9311980867048,-50.0385825039234,24.2));
#25157=CARTESIAN_POINT('Origin',(0.,0.,24.2));
#25158=CARTESIAN_POINT('',(-18.9311980867048,-50.0385825039234,14.5));
#25159=CARTESIAN_POINT('Origin',(-19.1972756843392,-49.7011709228329,14.5));
#25160=CARTESIAN_POINT('',(-19.4633532819736,-49.3637593417425,24.2));
#25161=CARTESIAN_POINT('',(-19.3672978885043,-49.485566673404,24.2));
#25162=CARTESIAN_POINT('',(-19.4633532819736,-49.3637593417425,11.5));
#25163=CARTESIAN_POINT('',(-19.4633532819736,-49.3637593417425,14.5));
#25164=CARTESIAN_POINT('Ctrl Pts',(-19.4633532819736,-49.3637593417425,
11.5));
#25165=CARTESIAN_POINT('Ctrl Pts',(-19.3380593316065,-49.5226439313144,
11.4654707447276));
#25166=CARTESIAN_POINT('Ctrl Pts',(-19.1764300887141,-49.7276051113597,
11.2969997378715));
#25167=CARTESIAN_POINT('Origin',(-20.7159699453405,-49.087578612363,14.5));
#25168=CARTESIAN_POINT('',(-21.1417559303916,-49.1454591613483,24.2));
#25169=CARTESIAN_POINT('',(-20.2901839602894,-49.0296980633778,24.2));
#25170=CARTESIAN_POINT('',(-20.4438949103711,-49.0505932419138,24.2));
#25171=CARTESIAN_POINT('',(-21.1417559303916,-49.1454591613483,11.5));
#25172=CARTESIAN_POINT('',(-21.1417559303916,-49.1454591613483,14.5));
#25173=CARTESIAN_POINT('',(-20.7493277422619,-49.0921132087719,11.2969997378715));
#25174=CARTESIAN_POINT('Ctrl Pts',(-21.1417559303916,-49.1454591613483,
11.5));
#25175=CARTESIAN_POINT('Ctrl Pts',(-20.945168871612,-49.1187354849356,11.3977655520828));
#25176=CARTESIAN_POINT('Ctrl Pts',(-20.7493277422619,-49.0921132087719,
11.2969997378715));
#25177=CARTESIAN_POINT('',(-20.2901839602894,-49.0296980633778,11.5));
#25178=CARTESIAN_POINT('Ctrl Pts',(-20.7493277422619,-49.0921132087719,
11.2969997378715));
#25179=CARTESIAN_POINT('Ctrl Pts',(-20.4906833956133,-49.056953580927,11.4654707447276));
#25180=CARTESIAN_POINT('Ctrl Pts',(-20.2901839602894,-49.0296980633778,
11.5));
#25181=CARTESIAN_POINT('',(-20.2901839602894,-49.0296980633778,14.5));
#25182=CARTESIAN_POINT('Origin',(0.,0.,11.25));
#25183=CARTESIAN_POINT('',(-22.3755977062724,-48.5961174095941,11.5));
#25184=CARTESIAN_POINT('Origin',(0.,0.,11.5));
#25185=CARTESIAN_POINT('',(-22.5985396491308,-48.2687910226197,11.2969997378715));
#25186=CARTESIAN_POINT('Ctrl Pts',(-22.5985396491308,-48.2687910226197,
11.2969997378715));
#25187=CARTESIAN_POINT('Ctrl Pts',(-22.4872805622725,-48.4321431243036,
11.3977655520825));
#25188=CARTESIAN_POINT('Ctrl Pts',(-22.3755977062724,-48.5961174095941,
11.5));
#25189=CARTESIAN_POINT('Ctrl Pts',(-22.5985396491308,-48.2687910226197,
11.2969997378715));
#25190=CARTESIAN_POINT('Ctrl Pts',(-22.4935659408428,-48.2094323095332,
11.1987310576086));
#25191=CARTESIAN_POINT('Ctrl Pts',(-22.3928669106239,-48.1443140553513,
11.0971961933879));
#25192=CARTESIAN_POINT('Ctrl Pts',(-22.300486949685,-48.0800195695356,11.));
#25193=CARTESIAN_POINT('Ctrl Pts',(-20.7493277422619,-49.0921132087719,
11.2969997378715));
#25194=CARTESIAN_POINT('Ctrl Pts',(-20.7754567428632,-48.9743838089662,
11.1987310576087));
#25195=CARTESIAN_POINT('Ctrl Pts',(-20.7944452523739,-48.8559772288226,
11.0971961933879));
#25196=CARTESIAN_POINT('Ctrl Pts',(-20.8084793972118,-48.7443041305937,
11.));
#25197=CARTESIAN_POINT('Origin',(0.,0.,14.5));
#25198=CARTESIAN_POINT('',(-22.3755977062724,-48.5961174095941,24.2));
#25199=CARTESIAN_POINT('Origin',(0.,0.,24.2));
#25200=CARTESIAN_POINT('',(-22.3755977062724,-48.5961174095941,14.5));
#25201=CARTESIAN_POINT('Origin',(-22.6174905101547,-48.2409671112037,14.5));
#25202=CARTESIAN_POINT('',(-22.859383314037,-47.8858168128132,24.2));
#25203=CARTESIAN_POINT('',(-22.7720587566113,-48.0140279134694,24.2));
#25204=CARTESIAN_POINT('',(-22.859383314037,-47.8858168128132,11.5));
#25205=CARTESIAN_POINT('',(-22.859383314037,-47.8858168128132,14.5));
#25206=CARTESIAN_POINT('Ctrl Pts',(-22.859383314037,-47.8858168128132,11.5));
#25207=CARTESIAN_POINT('Ctrl Pts',(-22.7454778021365,-48.0530544316696,
11.4654707447276));
#25208=CARTESIAN_POINT('Ctrl Pts',(-22.5985396491308,-48.2687910226197,
11.2969997378715));
#25209=CARTESIAN_POINT('Origin',(-24.0896832723708,-47.5229307244201,14.5));
#25210=CARTESIAN_POINT('',(-24.5184696071579,-47.5509689504102,24.2));
#25211=CARTESIAN_POINT('',(-23.6608969375837,-47.49489249843,24.2));
#25212=CARTESIAN_POINT('',(-23.8156910294893,-47.5050144435077,24.2));
#25213=CARTESIAN_POINT('',(-24.5184696071579,-47.5509689504102,11.5));
#25214=CARTESIAN_POINT('',(-24.5184696071579,-47.5509689504102,14.5));
#25215=CARTESIAN_POINT('',(-24.1232761288307,-47.5251273524949,11.2969997378715));
#25216=CARTESIAN_POINT('Ctrl Pts',(-24.5184696071579,-47.5509689504102,
11.5));
#25217=CARTESIAN_POINT('Ctrl Pts',(-24.3204972751409,-47.5380235915343,
11.3977655520827));
#25218=CARTESIAN_POINT('Ctrl Pts',(-24.1232761288307,-47.5251273524949,
11.2969997378715));
#25219=CARTESIAN_POINT('',(-23.6608969375837,-47.49489249843,11.5));
#25220=CARTESIAN_POINT('Ctrl Pts',(-24.1232761288307,-47.5251273524949,
11.2969997378715));
#25221=CARTESIAN_POINT('Ctrl Pts',(-23.8628092151545,-47.5080954893125,
11.4654707447276));
#25222=CARTESIAN_POINT('Ctrl Pts',(-23.6608969375837,-47.49489249843,11.5));
#25223=CARTESIAN_POINT('',(-23.6608969375837,-47.49489249843,14.5));
#25224=CARTESIAN_POINT('Origin',(0.,0.,11.25));
#25225=CARTESIAN_POINT('',(-25.7109856630024,-46.9168969161099,11.5));
#25226=CARTESIAN_POINT('Origin',(0.,0.,11.5));
#25227=CARTESIAN_POINT('',(-25.9105513959742,-46.5748162359794,11.2969997378715));
#25228=CARTESIAN_POINT('Ctrl Pts',(-25.9105513959742,-46.5748162359794,
11.2969997378715));
#25229=CARTESIAN_POINT('Ctrl Pts',(-25.8109581972506,-46.7455314617269,
11.3977655520837));
#25230=CARTESIAN_POINT('Ctrl Pts',(-25.7109856630024,-46.9168969161099,
11.5));
#25231=CARTESIAN_POINT('Ctrl Pts',(-25.9105513959742,-46.5748162359794,
11.2969997378714));
#25232=CARTESIAN_POINT('Ctrl Pts',(-25.8016927438527,-46.5229247134606,
11.1987310576086));
#25233=CARTESIAN_POINT('Ctrl Pts',(-25.6966965916221,-46.4649894933305,
11.0971961933879));
#25234=CARTESIAN_POINT('Ctrl Pts',(-25.6000567070135,-46.4072957259707,
11.));
#25235=CARTESIAN_POINT('Ctrl Pts',(-24.1232761288307,-47.5251273524949,
11.2969997378715));
#25236=CARTESIAN_POINT('Ctrl Pts',(-24.1411290927132,-47.4058620686457,
11.1987310576086));
#25237=CARTESIAN_POINT('Ctrl Pts',(-24.1518117216703,-47.2864193495151,
11.0971961933879));
#25238=CARTESIAN_POINT('Ctrl Pts',(-24.1580217584921,-47.174039308885,11.));
#25239=CARTESIAN_POINT('Origin',(0.,0.,14.5));
#25240=CARTESIAN_POINT('',(-25.7109856630024,-46.9168969161099,24.2));
#25241=CARTESIAN_POINT('Origin',(0.,0.,24.2));
#25242=CARTESIAN_POINT('',(-25.7109856630024,-46.9168969161099,14.5));
#25243=CARTESIAN_POINT('Origin',(-25.927515195707,-46.5457381569737,14.5));
#25244=CARTESIAN_POINT('',(-26.1440447284116,-46.1745793978374,24.2));
#25245=CARTESIAN_POINT('',(-26.0658764434955,-46.3085696358935,24.2));
#25246=CARTESIAN_POINT('',(-26.1440447284116,-46.1745793978374,11.5));
#25247=CARTESIAN_POINT('',(-26.1440447284116,-46.1745793978374,14.5));
#25248=CARTESIAN_POINT('Ctrl Pts',(-26.1440447284116,-46.1745793978374,
11.5));
#25249=CARTESIAN_POINT('Ctrl Pts',(-26.0420825911821,-46.3493552811098,
11.4654707447276));
#25250=CARTESIAN_POINT('Ctrl Pts',(-25.9105513959742,-46.5748162359794,
11.2969997378715));
#25251=CARTESIAN_POINT('Origin',(-27.3460340839844,-45.7267558949761,14.5));
#25252=CARTESIAN_POINT('',(-27.7757317645859,-45.7248151985525,24.2));
#25253=CARTESIAN_POINT('',(-26.916336403383,-45.7286965913998,24.2));
#25254=CARTESIAN_POINT('',(-27.0714594958568,-45.7279959899202,24.2));
#25255=CARTESIAN_POINT('',(-27.7757317645859,-45.7248151985525,11.5));
#25256=CARTESIAN_POINT('',(-27.7757317645859,-45.7248151985525,14.5));
#25257=CARTESIAN_POINT('',(-27.379698338963,-45.7266038529657,11.2969997378715));
#25258=CARTESIAN_POINT('Ctrl Pts',(-27.7757317645859,-45.7248151985525,
11.5));
#25259=CARTESIAN_POINT('Ctrl Pts',(-27.5773386606333,-45.7257112257006,
11.3977655520828));
#25260=CARTESIAN_POINT('Ctrl Pts',(-27.379698338963,-45.7266038529657,11.2969997378715));
#25261=CARTESIAN_POINT('',(-26.916336403383,-45.7286965913998,11.5));
#25262=CARTESIAN_POINT('Ctrl Pts',(-27.379698338963,-45.7266038529657,11.2969997378715));
#25263=CARTESIAN_POINT('Ctrl Pts',(-27.1186778268806,-45.727782731971,11.4654707447276));
#25264=CARTESIAN_POINT('Ctrl Pts',(-26.916336403383,-45.7286965913998,11.5));
#25265=CARTESIAN_POINT('',(-26.916336403383,-45.7286965913998,14.5));
#25266=CARTESIAN_POINT('Origin',(0.,0.,11.25));
#25267=CARTESIAN_POINT('',(-28.9211122820413,-45.0091020169205,11.5));
#25268=CARTESIAN_POINT('Origin',(0.,0.,11.5));
#25269=CARTESIAN_POINT('',(-29.0963295409359,-44.6539336263215,11.2969997378715));
#25270=CARTESIAN_POINT('Ctrl Pts',(-29.0963295409359,-44.6539336263215,
11.2969997378715));
#25271=CARTESIAN_POINT('Ctrl Pts',(-29.0088874384024,-44.8311802687092,
11.3977655520826));
#25272=CARTESIAN_POINT('Ctrl Pts',(-28.9211122820413,-45.0091020169205,
11.5));
#25273=CARTESIAN_POINT('Ctrl Pts',(-29.0963295409359,-44.6539336263215,
11.2969997378715));
#25274=CARTESIAN_POINT('Ctrl Pts',(-28.9841162933917,-44.6097621046521,
11.1987310576087));
#25275=CARTESIAN_POINT('Ctrl Pts',(-28.875334549849,-44.5592921731428,11.0971961933879));
#25276=CARTESIAN_POINT('Ctrl Pts',(-28.774905561374,-44.5084802024738,11.));
#25277=CARTESIAN_POINT('Ctrl Pts',(-27.379698338963,-45.7266038529657,11.2969997378715));
#25278=CARTESIAN_POINT('Ctrl Pts',(-27.3891882882814,-45.6063837335473,
11.1987310576086));
#25279=CARTESIAN_POINT('Ctrl Pts',(-27.3915129919902,-45.486486788351,11.0971961933879));
#25280=CARTESIAN_POINT('Ctrl Pts',(-27.3898686661209,-45.3739473095812,
11.));
#25281=CARTESIAN_POINT('Origin',(0.,0.,14.5));
#25282=CARTESIAN_POINT('',(-28.9211122820413,-45.0091020169205,24.2));
#25283=CARTESIAN_POINT('Origin',(0.,0.,24.2));
#25284=CARTESIAN_POINT('',(-28.9211122820413,-45.0091020169205,14.5));
#25285=CARTESIAN_POINT('Origin',(-29.1112236334504,-44.6237430452042,14.5));
#25286=CARTESIAN_POINT('',(-29.3013349848595,-44.2383840734879,24.2));
#25287=CARTESIAN_POINT('',(-29.2327038004797,-44.3775006619728,24.2));
#25288=CARTESIAN_POINT('',(-29.3013349848595,-44.2383840734879,11.5));
#25289=CARTESIAN_POINT('',(-29.3013349848595,-44.2383840734879,14.5));
#25290=CARTESIAN_POINT('Ctrl Pts',(-29.3013349848595,-44.2383840734879,
11.5));
#25291=CARTESIAN_POINT('Ctrl Pts',(-29.2118129715843,-44.4198467306414,
11.4654707447275));
#25292=CARTESIAN_POINT('Ctrl Pts',(-29.0963295409359,-44.6539336263215,
11.2969997378715));
#25293=CARTESIAN_POINT('Origin',(-30.4691577663544,-43.7078049072494,14.5));
#25294=CARTESIAN_POINT('',(-30.8976733488633,-43.67589474329,24.2));
#25295=CARTESIAN_POINT('',(-30.0406421838456,-43.7397150712088,24.2));
#25296=CARTESIAN_POINT('',(-30.1953385327739,-43.728195336432,24.2));
#25297=CARTESIAN_POINT('',(-30.8976733488633,-43.67589474329,11.5));
#25298=CARTESIAN_POINT('',(-30.8976733488632,-43.67589474329,14.5));
#25299=CARTESIAN_POINT('',(-30.5027294109855,-43.7053049358871,11.2969997378715));
#25300=CARTESIAN_POINT('Ctrl Pts',(-30.8976733488633,-43.67589474329,11.5));
#25301=CARTESIAN_POINT('Ctrl Pts',(-30.6998260242329,-43.690627791108,11.3977655520818));
#25302=CARTESIAN_POINT('Ctrl Pts',(-30.5027294109855,-43.7053049358871,
11.2969997378715));
#25303=CARTESIAN_POINT('',(-30.0406421838456,-43.7397150712088,11.5));
#25304=CARTESIAN_POINT('Ctrl Pts',(-30.5027294109855,-43.7053049358871,
11.2969997378715));
#25305=CARTESIAN_POINT('Ctrl Pts',(-30.242426966194,-43.7246888137001,11.4654707447276));
#25306=CARTESIAN_POINT('Ctrl Pts',(-30.0406421838456,-43.7397150712088,
11.5));
#25307=CARTESIAN_POINT('',(-30.0406421838456,-43.7397150712088,14.5));
#25308=CARTESIAN_POINT('Origin',(0.,0.,11.25));
#25309=CARTESIAN_POINT('',(-31.9903381491823,-42.8820272970037,11.5));
#25310=CARTESIAN_POINT('Origin',(0.,0.,11.5));
#25311=CARTESIAN_POINT('',(-32.140353293127,-42.5155015406339,11.2969997378715));
#25312=CARTESIAN_POINT('Ctrl Pts',(-32.140353293127,-42.5155015406339,11.2969997378715));
#25313=CARTESIAN_POINT('Ctrl Pts',(-32.0654882959165,-42.6984160718384,
11.3977655520825));
#25314=CARTESIAN_POINT('Ctrl Pts',(-31.9903381491823,-42.8820272970037,
11.5));
#25315=CARTESIAN_POINT('Ctrl Pts',(-32.140353293127,-42.515501540634,11.2969997378715));
#25316=CARTESIAN_POINT('Ctrl Pts',(-32.0253321418224,-42.4792652190273,
11.1987310576087));
#25317=CARTESIAN_POINT('Ctrl Pts',(-31.9132947806875,-42.4365064605718,
11.0971961933879));
#25318=CARTESIAN_POINT('Ctrl Pts',(-31.809565968283,-42.3928238374073,11.));
#25319=CARTESIAN_POINT('Ctrl Pts',(-30.5027294109855,-43.7053049358871,
11.2969997378715));
#25320=CARTESIAN_POINT('Ctrl Pts',(-30.5038101116606,-43.5847156812369,
11.1987310576087));
#25321=CARTESIAN_POINT('Ctrl Pts',(-30.4977655643985,-43.4649486358399,
11.0971961933879));
#25322=CARTESIAN_POINT('Ctrl Pts',(-30.4882748868283,-43.3527979999583,
11.));
#25323=CARTESIAN_POINT('Origin',(0.,0.,14.5));
#25324=CARTESIAN_POINT('',(-31.9903381491823,-42.8820272970037,24.2));
#25325=CARTESIAN_POINT('Origin',(0.,0.,24.2));
#25326=CARTESIAN_POINT('',(-31.9903381491823,-42.8820272970037,14.5));
#25327=CARTESIAN_POINT('Origin',(-32.1531051159017,-42.4843455428814,14.5));
#25328=CARTESIAN_POINT('',(-32.3158720826212,-42.0866637887591,24.2));
#25329=CARTESIAN_POINT('',(-32.2571123630091,-42.2302289656376,24.2));
#25330=CARTESIAN_POINT('',(-32.3158720826212,-42.0866637887591,11.5));
#25331=CARTESIAN_POINT('',(-32.3158720826212,-42.0866637887591,14.5));
#25332=CARTESIAN_POINT('Ctrl Pts',(-32.3158720826212,-42.0866637887591,
11.5));
#25333=CARTESIAN_POINT('Ctrl Pts',(-32.2392263355501,-42.2739291519686,
11.4654707447276));
#25334=CARTESIAN_POINT('Ctrl Pts',(-32.140353293127,-42.5155015406339,11.2969997378715));
#25335=CARTESIAN_POINT('Origin',(-33.443838774836,-41.4759138875076,14.5));
#25336=CARTESIAN_POINT('',(-33.8690845744085,-41.4141897191236,24.2));
#25337=CARTESIAN_POINT('',(-33.0185929752635,-41.5376380558916,24.2));
#25338=CARTESIAN_POINT('',(-33.1721089155843,-41.5153553108074,24.2));
#25339=CARTESIAN_POINT('',(-33.8690845744085,-41.4141897191236,11.5));
#25340=CARTESIAN_POINT('',(-33.8690845744085,-41.4141897191236,14.5));
#25341=CARTESIAN_POINT('',(-33.4771542514413,-41.4710781664027,11.2969997378715));
#25342=CARTESIAN_POINT('Ctrl Pts',(-33.8690845744085,-41.4141897191236,
11.5));
#25343=CARTESIAN_POINT('Ctrl Pts',(-33.6727469213825,-41.4426880096833,
11.3977655520828));
#25344=CARTESIAN_POINT('Ctrl Pts',(-33.4771542514413,-41.4710781664027,
11.2969997378715));
#25345=CARTESIAN_POINT('',(-33.0185929752635,-41.5376380558916,11.5));
#25346=CARTESIAN_POINT('Ctrl Pts',(-33.4771542514414,-41.4710781664027,
11.2969997378715));
#25347=CARTESIAN_POINT('Ctrl Pts',(-33.2188380412863,-41.5085726067192,
11.4654707447276));
#25348=CARTESIAN_POINT('Ctrl Pts',(-33.0185929752635,-41.5376380558916,
11.5));
#25349=CARTESIAN_POINT('',(-33.0185929752635,-41.5376380558916,14.5));
#25350=CARTESIAN_POINT('Origin',(0.,0.,11.25));
#25351=CARTESIAN_POINT('',(-34.9037103045182,-40.546035650582,11.5));
#25352=CARTESIAN_POINT('Origin',(0.,0.,11.5));
#25353=CARTESIAN_POINT('',(-35.1729694999764,-39.7299015085879,11.0622545443402));
#25354=CARTESIAN_POINT('Ctrl Pts',(-35.1729694999764,-39.7299015085879,
11.0622545443402));
#25355=CARTESIAN_POINT('Ctrl Pts',(-35.0388929451123,-40.1362922871065,
11.2776618075219));
#25356=CARTESIAN_POINT('Ctrl Pts',(-34.9037103045182,-40.546035650582,11.5));
#25357=CARTESIAN_POINT('Ctrl Pts',(-35.1966714489987,-39.6256775199017,
11.));
#25358=CARTESIAN_POINT('Ctrl Pts',(-35.1856729924399,-39.6612285891332,
11.0192759649605));
#25359=CARTESIAN_POINT('Ctrl Pts',(-35.1779404204734,-39.6963735392364,
11.0404458048696));
#25360=CARTESIAN_POINT('Ctrl Pts',(-35.1729694999764,-39.7299015085879,
11.0622545443403));
#25361=CARTESIAN_POINT('Ctrl Pts',(-33.4771542514414,-41.4710781664027,
11.2969997378715));
#25362=CARTESIAN_POINT('Ctrl Pts',(-33.4698204384081,-41.3507072752478,
11.1987310576087));
#25363=CARTESIAN_POINT('Ctrl Pts',(-33.4554360886017,-41.2316536226562,
11.0971961933879));
#25364=CARTESIAN_POINT('Ctrl Pts',(-33.4381452969578,-41.1204382162877,
11.));
#25365=CARTESIAN_POINT('Origin',(0.,0.,14.5));
#25366=CARTESIAN_POINT('',(-34.9037103045182,-40.546035650582,24.2));
#25367=CARTESIAN_POINT('Origin',(0.,0.,24.2));
#25368=CARTESIAN_POINT('',(-34.9037103045182,-40.546035650582,14.5));
#25369=CARTESIAN_POINT('Origin',(-36.2555847625695,-39.0419563844502,14.5));
#25370=CARTESIAN_POINT('',(-35.8356805007232,-39.1331938433149,11.0622545443404));
#25371=CARTESIAN_POINT('',(-35.8356805007232,-39.1331938433149,24.2));
#25372=CARTESIAN_POINT('',(-35.8356805007232,-39.1331938433149,14.5));
#25373=CARTESIAN_POINT('',(-36.6754890244158,-38.9507189255854,24.2));
#25374=CARTESIAN_POINT('',(-35.9872681182067,-39.1002566472175,24.2));
#25375=CARTESIAN_POINT('',(-36.6754890244158,-38.9507189255854,11.5));
#25376=CARTESIAN_POINT('',(-36.6754890244158,-38.9507189255854,14.5));
#25377=CARTESIAN_POINT('Ctrl Pts',(-36.6754890244158,-38.9507189255854,
11.5));
#25378=CARTESIAN_POINT('Ctrl Pts',(-36.3962351235305,-39.0113956526632,
11.3527407245755));
#25379=CARTESIAN_POINT('Ctrl Pts',(-36.1162869832672,-39.0722232251656,
11.206797012465));
#25380=CARTESIAN_POINT('Ctrl Pts',(-35.8356805007232,-39.1331938433149,
11.0622545443404));
#25381=CARTESIAN_POINT('Origin',(0.,0.,11.25));
#25382=CARTESIAN_POINT('Ctrl Pts',(-35.7295499336443,-39.1458715772075,
11.));
#25383=CARTESIAN_POINT('Ctrl Pts',(-35.7660555066417,-39.1386495482258,
11.0192757561174));
#25384=CARTESIAN_POINT('Ctrl Pts',(-35.8018169409009,-39.1346328909224,
11.0404460254343));
#25385=CARTESIAN_POINT('Ctrl Pts',(-35.8356805007232,-39.1331938433149,
11.0622545443404));
#25386=CARTESIAN_POINT('Origin',(0.,0.,11.5));
#25387=CARTESIAN_POINT('Origin',(0.,0.,11.25));
#25388=CARTESIAN_POINT('Origin',(0.,0.,11.5));
#25389=CARTESIAN_POINT('Origin',(0.,0.,11.25));
#25390=CARTESIAN_POINT('Origin',(0.,0.,11.5));
#25391=CARTESIAN_POINT('Origin',(0.,0.,14.5));
#25392=CARTESIAN_POINT('Origin',(0.,0.,24.2));
#25393=CARTESIAN_POINT('Origin',(0.,0.,14.5));
#25394=CARTESIAN_POINT('Origin',(0.,0.,24.2));
#25395=CARTESIAN_POINT('Origin',(0.,0.,14.5));
#25396=CARTESIAN_POINT('Origin',(0.,0.,24.2));
#25397=CARTESIAN_POINT('Origin',(-35.0383399022473,-40.137968579585,14.5));
#25398=CARTESIAN_POINT('',(-35.1729694999764,-39.729901508588,24.2));
#25399=CARTESIAN_POINT('',(-35.1243675165795,-39.8772158387497,24.2));
#25400=CARTESIAN_POINT('',(-35.1729694999764,-39.729901508588,14.5));
#25401=CARTESIAN_POINT('Origin',(-20.0789134070929,-49.6970546047798,11.25));
#25402=CARTESIAN_POINT('Origin',(-20.0789134070929,-49.6970546047798,11.5));
#25403=CARTESIAN_POINT('Origin',(-23.4966934678946,-48.1753608816353,11.25));
#25404=CARTESIAN_POINT('Origin',(-23.4966934678946,-48.1753608816353,11.5));
#25405=CARTESIAN_POINT('Origin',(-26.8,-46.4189616428459,11.25));
#25406=CARTESIAN_POINT('Origin',(-26.8,-46.4189616428459,11.5));
#25407=CARTESIAN_POINT('Origin',(-29.972739626032,-44.4364138889502,11.25));
#25408=CARTESIAN_POINT('Origin',(-29.972739626032,-44.4364138889502,11.5));
#25409=CARTESIAN_POINT('Origin',(-32.9994550774553,-42.2373763933203,11.25));
#25410=CARTESIAN_POINT('Origin',(-32.9994550774553,-42.2373763933203,11.5));
#25411=CARTESIAN_POINT('Origin',(-35.8654005008348,-39.8325626455883,11.));
#25412=CARTESIAN_POINT('Origin',(-35.8654005008348,-39.8325626455883,24.2));
#25413=CARTESIAN_POINT('Origin',(-32.9994550774553,-42.2373763933203,11.));
#25414=CARTESIAN_POINT('Origin',(-32.9994550774553,-42.2373763933203,24.2));
#25415=CARTESIAN_POINT('Origin',(-29.972739626032,-44.4364138889502,11.));
#25416=CARTESIAN_POINT('Origin',(-29.972739626032,-44.4364138889502,24.2));
#25417=CARTESIAN_POINT('Origin',(-26.8,-46.4189616428459,11.));
#25418=CARTESIAN_POINT('Origin',(-26.8,-46.4189616428459,24.2));
#25419=CARTESIAN_POINT('Origin',(-23.4966934678946,-48.1753608816353,11.));
#25420=CARTESIAN_POINT('Origin',(-23.4966934678946,-48.1753608816353,24.2));
#25421=CARTESIAN_POINT('Origin',(-20.0789134070929,-49.6970546047798,11.));
#25422=CARTESIAN_POINT('Origin',(-20.0789134070929,-49.6970546047798,24.2));
#25423=CARTESIAN_POINT('Origin',(-1.04073669728539,-53.2696785416253,14.5));
#25424=CARTESIAN_POINT('',(-1.012107219952,-53.287388939917,11.2969997378715));
#25425=CARTESIAN_POINT('',(-0.675303984907606,-53.495737816465,11.5));
#25426=CARTESIAN_POINT('Ctrl Pts',(-1.012107219952,-53.287388939917,11.2969997378715));
#25427=CARTESIAN_POINT('Ctrl Pts',(-0.844025701051962,-53.3913653629068,
11.397765552083));
#25428=CARTESIAN_POINT('Ctrl Pts',(-0.675303984907606,-53.495737816465,
11.5));
#25429=CARTESIAN_POINT('',(-0.675303984907606,-53.495737816465,24.2));
#25430=CARTESIAN_POINT('',(-0.675303984907606,-53.495737816465,14.5));
#25431=CARTESIAN_POINT('',(-1.40616940966318,-53.0436192667856,24.2));
#25432=CARTESIAN_POINT('',(-1.27424630420036,-53.1252278380639,24.2));
#25433=CARTESIAN_POINT('',(-1.40616940966318,-53.0436192667856,11.5));
#25434=CARTESIAN_POINT('',(-1.40616940966318,-53.0436192667856,14.5));
#25435=CARTESIAN_POINT('Ctrl Pts',(-1.40616940966318,-53.0436192667856,
11.5));
#25436=CARTESIAN_POINT('Ctrl Pts',(-1.23408987897642,-53.1500688883006,
11.4654707447276));
#25437=CARTESIAN_POINT('Ctrl Pts',(-1.012107219952,-53.287388939917,11.2969997378715));
#25438=CARTESIAN_POINT('Origin',(-1.87061302325404,-53.5673483282235,11.25));
#25439=CARTESIAN_POINT('',(-2.29739178302175,-53.0124970957196,11.5));
#25440=CARTESIAN_POINT('Origin',(-1.87061302325404,-53.5673483282235,11.5));
#25441=CARTESIAN_POINT('',(-2.70749856984771,-53.2281845693891,11.2969997378715));
#25442=CARTESIAN_POINT('Ctrl Pts',(-2.70749856984771,-53.2281845693891,
11.2969997378715));
#25443=CARTESIAN_POINT('Ctrl Pts',(-2.47647768684878,-53.1066837500425,
11.4654707447276));
#25444=CARTESIAN_POINT('Ctrl Pts',(-2.29739178302175,-53.0124970957196,
11.5));
#25445=CARTESIAN_POINT('Ctrl Pts',(-2.88204065427986,-52.9215820026866,
11.));
#25446=CARTESIAN_POINT('Ctrl Pts',(-2.83065842287485,-53.0217204288036,
11.0971961933879));
#25447=CARTESIAN_POINT('Ctrl Pts',(-2.77231762509644,-53.1264917656727,
11.1987310576087));
#25448=CARTESIAN_POINT('Ctrl Pts',(-2.70749856984771,-53.2281845693891,
11.2969997378715));
#25449=CARTESIAN_POINT('Ctrl Pts',(-1.01210721995201,-53.287388939917,11.2969997378715));
#25450=CARTESIAN_POINT('Ctrl Pts',(-0.940352329271679,-53.190465403485,
11.1987310576086));
#25451=CARTESIAN_POINT('Ctrl Pts',(-0.874845167735035,-53.0900189326552,
11.0971961933879));
#25452=CARTESIAN_POINT('Ctrl Pts',(-0.816602797371071,-52.9937086819872,
11.));
#25453=CARTESIAN_POINT('Origin',(-1.87061302325404,-53.5673483282235,11.));
#25454=CARTESIAN_POINT('',(-2.29739178302175,-53.0124970957196,24.2));
#25455=CARTESIAN_POINT('Origin',(-1.87061302325404,-53.5673483282235,24.2));
#25456=CARTESIAN_POINT('',(-2.29739178302175,-53.0124970957196,14.5));
#25457=CARTESIAN_POINT('Origin',(-2.67770341754862,-53.2125144041213,14.5));
#25458=CARTESIAN_POINT('',(-3.05801505207549,-53.412531712523,24.2));
#25459=CARTESIAN_POINT('',(-2.43468625658981,-53.0847043819776,24.2));
#25460=CARTESIAN_POINT('',(-3.05801505207549,-53.412531712523,11.5));
#25461=CARTESIAN_POINT('',(-3.05801505207549,-53.412531712523,14.5));
#25462=CARTESIAN_POINT('Ctrl Pts',(-3.05801505207549,-53.412531712523,11.5));
#25463=CARTESIAN_POINT('Ctrl Pts',(-2.88242367923521,-53.320182936978,11.3977655520828));
#25464=CARTESIAN_POINT('Ctrl Pts',(-2.70749856984771,-53.2281845693891,
11.2969997378715));
#25465=CARTESIAN_POINT('Origin',(0.,0.,11.25));
#25466=CARTESIAN_POINT('',(-4.40533300875789,-53.318318063138,11.5));
#25467=CARTESIAN_POINT('Origin',(0.,0.,11.5));
#25468=CARTESIAN_POINT('',(-4.72678212511286,-53.0869825079594,11.2969997378715));
#25469=CARTESIAN_POINT('Ctrl Pts',(-4.72678212511286,-53.0869825079594,
11.2969997378715));
#25470=CARTESIAN_POINT('Ctrl Pts',(-4.56636307296501,-53.2024304236689,
11.3977655520833));
#25471=CARTESIAN_POINT('Ctrl Pts',(-4.40533300875789,-53.318318063138,11.5));
#25472=CARTESIAN_POINT('Ctrl Pts',(-4.72678212511287,-53.0869825079594,
11.2969997378715));
#25473=CARTESIAN_POINT('Ctrl Pts',(-4.64844098161556,-52.9953004405385,
11.1987310576086));
#25474=CARTESIAN_POINT('Ctrl Pts',(-4.57608660062692,-52.8996682008571,
11.0971961933879));
#25475=CARTESIAN_POINT('Ctrl Pts',(-4.51126784227787,-52.8076553394982,
11.));
#25476=CARTESIAN_POINT('Origin',(-4.75410644754494,-53.0673181599239,14.5));
#25477=CARTESIAN_POINT('',(-4.40533300875789,-53.318318063138,24.2));
#25478=CARTESIAN_POINT('',(-4.40533300875789,-53.318318063138,14.5));
#25479=CARTESIAN_POINT('',(-5.10287988633199,-52.8163182567097,24.2));
#25480=CARTESIAN_POINT('',(-4.97697086508331,-52.9069305242525,24.2));
#25481=CARTESIAN_POINT('',(-5.10287988633199,-52.8163182567097,11.5));
#25482=CARTESIAN_POINT('',(-5.10287988633199,-52.8163182567097,14.5));
#25483=CARTESIAN_POINT('Ctrl Pts',(-5.10287988633199,-52.8163182567097,
11.5));
#25484=CARTESIAN_POINT('Ctrl Pts',(-4.93864508296158,-52.9345122335611,
11.4654707447276));
#25485=CARTESIAN_POINT('Ctrl Pts',(-4.72678212511286,-53.0869825079594,
11.2969997378715));
#25486=CARTESIAN_POINT('Origin',(-5.60272563114622,-53.3063735917395,11.25));
#25487=CARTESIAN_POINT('',(-5.98976031387286,-52.7231033676009,11.5));
#25488=CARTESIAN_POINT('Origin',(-5.60272563114622,-53.3063735917395,11.5));
#25489=CARTESIAN_POINT('',(-6.413913698772,-52.9096578341174,11.2969997378716));
#25490=CARTESIAN_POINT('Ctrl Pts',(-6.413913698772,-52.9096578341174,11.2969997378716));
#25491=CARTESIAN_POINT('Ctrl Pts',(-6.17498010231831,-52.8045681868194,
11.4654707447277));
#25492=CARTESIAN_POINT('Ctrl Pts',(-5.98976031387286,-52.7231033676009,
11.5));
#25493=CARTESIAN_POINT('Ctrl Pts',(-6.41391369877199,-52.9096578341175,
11.2969997378716));
#25494=CARTESIAN_POINT('Ctrl Pts',(-6.47148112666751,-52.8036912002343,
11.1987310576087));
#25495=CARTESIAN_POINT('Ctrl Pts',(-6.52237133018529,-52.6951054327476,
11.0971961933879));
#25496=CARTESIAN_POINT('Ctrl Pts',(-6.56664309356486,-52.5916266955277,
11.));
#25497=CARTESIAN_POINT('Origin',(-5.60272563114622,-53.3063735917395,11.));
#25498=CARTESIAN_POINT('',(-5.98976031387285,-52.7231033676009,24.2));
#25499=CARTESIAN_POINT('Origin',(-5.60272563114622,-53.3063735917395,24.2));
#25500=CARTESIAN_POINT('',(-5.98976031387285,-52.7231033676009,14.5));
#25501=CARTESIAN_POINT('Origin',(-6.38309803049425,-52.8961042453437,14.5));
#25502=CARTESIAN_POINT('',(-6.77643574711566,-53.0691051230866,24.2));
#25503=CARTESIAN_POINT('',(-6.13175727067173,-52.785557582198,24.2));
#25504=CARTESIAN_POINT('',(-6.77643574711566,-53.0691051230866,11.5));
#25505=CARTESIAN_POINT('',(-6.77643574711566,-53.0691051230866,14.5));
#25506=CARTESIAN_POINT('Ctrl Pts',(-6.77643574711566,-53.0691051230866,
11.5));
#25507=CARTESIAN_POINT('Ctrl Pts',(-6.594830181098,-52.9892299395067,11.3977655520829));
#25508=CARTESIAN_POINT('Ctrl Pts',(-6.413913698772,-52.9096578341174,11.2969997378716));
#25509=CARTESIAN_POINT('Origin',(-8.44431466907315,-52.6064191384554,14.5));
#25510=CARTESIAN_POINT('',(-8.41842862289463,-52.6279416335078,11.2969997378715));
#25511=CARTESIAN_POINT('',(-8.11389969301203,-52.8811368237459,11.5));
#25512=CARTESIAN_POINT('Ctrl Pts',(-8.41842862289463,-52.6279416335078,
11.2969997378715));
#25513=CARTESIAN_POINT('Ctrl Pts',(-8.26645358299721,-52.7542985912954,
11.3977655520826));
#25514=CARTESIAN_POINT('Ctrl Pts',(-8.11389969301203,-52.8811368237459,
11.5));
#25515=CARTESIAN_POINT('',(-8.11389969301203,-52.8811368237459,24.2));
#25516=CARTESIAN_POINT('',(-8.11389969301203,-52.8811368237459,14.5));
#25517=CARTESIAN_POINT('',(-8.77472964513427,-52.3317014531649,24.2));
#25518=CARTESIAN_POINT('',(-8.65544812419494,-52.430875963113,24.2));
#25519=CARTESIAN_POINT('',(-8.77472964513427,-52.3317014531649,11.5));
#25520=CARTESIAN_POINT('',(-8.77472964513427,-52.3317014531649,14.5));
#25521=CARTESIAN_POINT('Ctrl Pts',(-8.77472964513427,-52.3317014531649,
11.5));
#25522=CARTESIAN_POINT('Ctrl Pts',(-8.6191397045334,-52.4610639561783,11.4654707447276));
#25523=CARTESIAN_POINT('Ctrl Pts',(-8.41842862289463,-52.6279416335078,
11.2969997378715));
#25524=CARTESIAN_POINT('Origin',(-9.30754232294747,-52.7856955614544,11.25));
#25525=CARTESIAN_POINT('',(-9.65294733456354,-52.1768479795831,11.5));
#25526=CARTESIAN_POINT('Origin',(-9.30754232294747,-52.7856955614544,11.5));
#25527=CARTESIAN_POINT('',(-10.0890808848803,-52.3333605643381,11.2969997378715));
#25528=CARTESIAN_POINT('Ctrl Pts',(-10.0890808848803,-52.3333605643381,
11.2969997378715));
#25529=CARTESIAN_POINT('Ctrl Pts',(-9.84339863543634,-52.2451940752868,
11.4654707447276));
#25530=CARTESIAN_POINT('Ctrl Pts',(-9.65294733456354,-52.1768479795831,
11.5));
#25531=CARTESIAN_POINT('Ctrl Pts',(-10.0890808848803,-52.3333605643381,
11.2969997378715));
#25532=CARTESIAN_POINT('Ctrl Pts',(-10.1391162227005,-52.2236363590767,
11.1987310576086));
#25533=CARTESIAN_POINT('Ctrl Pts',(-10.1823079000016,-52.1117651799167,
11.0971961933879));
#25534=CARTESIAN_POINT('Ctrl Pts',(-10.2192535077747,-52.0054502696,11.));
#25535=CARTESIAN_POINT('Ctrl Pts',(-8.41842862289464,-52.6279416335078,
11.2969997378715));
#25536=CARTESIAN_POINT('Ctrl Pts',(-8.33388289675662,-52.5419477009147,
11.1987310576086));
#25537=CARTESIAN_POINT('Ctrl Pts',(-8.25503379958712,-52.4515956030403,
11.0971961933879));
#25538=CARTESIAN_POINT('Ctrl Pts',(-8.18395444372813,-52.3643284084021,
11.));
#25539=CARTESIAN_POINT('Origin',(-9.30754232294747,-52.7856955614544,11.));
#25540=CARTESIAN_POINT('',(-9.65294733456354,-52.1768479795831,24.2));
#25541=CARTESIAN_POINT('Origin',(-9.30754232294747,-52.7856955614544,24.2));
#25542=CARTESIAN_POINT('',(-9.65294733456355,-52.1768479795831,14.5));
#25543=CARTESIAN_POINT('Origin',(-10.0573948314625,-52.3219895837806,14.5));
#25544=CARTESIAN_POINT('',(-10.4618423283614,-52.4671311879781,24.2));
#25545=CARTESIAN_POINT('',(-9.79895497969307,-52.2292448518636,24.2));
#25546=CARTESIAN_POINT('',(-10.4618423283614,-52.4671311879781,11.5));
#25547=CARTESIAN_POINT('',(-10.4618423283614,-52.4671311879781,14.5));
#25548=CARTESIAN_POINT('Ctrl Pts',(-10.4618423283614,-52.4671311879781,
11.5));
#25549=CARTESIAN_POINT('Ctrl Pts',(-10.275107333229,-52.4001187402287,11.397765552083));
#25550=CARTESIAN_POINT('Ctrl Pts',(-10.0890808848803,-52.3333605643381,
11.2969997378715));
#25551=CARTESIAN_POINT('Origin',(-12.0933830383532,-51.8892269309232,14.5));
#25552=CARTESIAN_POINT('',(-12.0690613826431,-51.9125027175599,11.2969997378715));
#25553=CARTESIAN_POINT('',(-11.7829362735682,-52.1863240013419,11.5));
#25554=CARTESIAN_POINT('Ctrl Pts',(-12.0690613826431,-51.9125027175599,
11.2969997378715));
#25555=CARTESIAN_POINT('Ctrl Pts',(-11.9262707621126,-52.0491531190297,
11.3977655520828));
#25556=CARTESIAN_POINT('Ctrl Pts',(-11.7829362735682,-52.1863240013419,
11.5));
#25557=CARTESIAN_POINT('',(-11.7829362735682,-52.1863240013419,24.2));
#25558=CARTESIAN_POINT('',(-11.7829362735682,-52.1863240013419,14.5));
#25559=CARTESIAN_POINT('',(-12.4038298031382,-51.5921298605045,24.2));
#25560=CARTESIAN_POINT('',(-12.2917569100881,-51.6993834446145,24.2));
#25561=CARTESIAN_POINT('',(-12.4038298031382,-51.5921298605045,11.5));
#25562=CARTESIAN_POINT('',(-12.4038298031382,-51.5921298605045,14.5));
#25563=CARTESIAN_POINT('Ctrl Pts',(-12.4038298031382,-51.5921298605045,
11.5));
#25564=CARTESIAN_POINT('Ctrl Pts',(-12.2576427438576,-51.7320306485686,
11.4654707447276));
#25565=CARTESIAN_POINT('Ctrl Pts',(-12.0690613826431,-51.9125027175599,
11.2969997378715));
#25566=CARTESIAN_POINT('Origin',(-12.9670136041422,-52.0078509283934,11.25));
#25567=CARTESIAN_POINT('',(-13.269106166151,-51.3763922330071,11.5));
#25568=CARTESIAN_POINT('Origin',(-12.9670136041422,-52.0078509283934,11.5));
#25569=CARTESIAN_POINT('',(-13.7150950830682,-51.5021004224203,11.2969997378715));
#25570=CARTESIAN_POINT('Ctrl Pts',(-13.7150950830682,-51.5021004224203,
11.2969997378715));
#25571=CARTESIAN_POINT('Ctrl Pts',(-13.4638611198574,-51.4312866298879,
11.4654707447276));
#25572=CARTESIAN_POINT('Ctrl Pts',(-13.269106166151,-51.3763922330071,11.5));
#25573=CARTESIAN_POINT('Ctrl Pts',(-13.7150950830682,-51.5021004224203,
11.2969997378715));
#25574=CARTESIAN_POINT('Ctrl Pts',(-13.7573545636769,-51.3891532110793,
11.1987310576086));
#25575=CARTESIAN_POINT('Ctrl Pts',(-13.7926372892511,-51.2745416453855,
11.0971961933879));
#25576=CARTESIAN_POINT('Ctrl Pts',(-13.8220767461304,-51.1659085175284,
11.));
#25577=CARTESIAN_POINT('Ctrl Pts',(-12.0690613826432,-51.9125027175599,
11.2969997378715));
#25578=CARTESIAN_POINT('Ctrl Pts',(-11.9787229721437,-51.8326158735901,
11.1987310576086));
#25579=CARTESIAN_POINT('Ctrl Pts',(-11.8937633036688,-51.7479841038615,
11.0971961933879));
#25580=CARTESIAN_POINT('Ctrl Pts',(-11.8167696417768,-51.6658877329441,
11.));
#25581=CARTESIAN_POINT('Origin',(-12.9670136041422,-52.0078509283934,11.));
#25582=CARTESIAN_POINT('',(-13.269106166151,-51.3763922330071,24.2));
#25583=CARTESIAN_POINT('Origin',(-12.9670136041422,-52.0078509283934,24.2));
#25584=CARTESIAN_POINT('',(-13.269106166151,-51.3763922330071,14.5));
#25585=CARTESIAN_POINT('Origin',(-15.6835336610931,-50.9192356256703,14.5));
#25586=CARTESIAN_POINT('',(-15.97249974917,-50.6012065971863,11.0622545443402));
#25587=CARTESIAN_POINT('',(-15.3945675730164,-51.2372646541541,11.5));
#25588=CARTESIAN_POINT('Ctrl Pts',(-15.97249974917,-50.6012065971863,11.0622545443402));
#25589=CARTESIAN_POINT('Ctrl Pts',(-15.6847207004672,-50.9179291990878,
11.2776618075209));
#25590=CARTESIAN_POINT('Ctrl Pts',(-15.3945675730164,-51.2372646541541,
11.5));
#25591=CARTESIAN_POINT('',(-15.3945675730164,-51.2372646541541,24.2));
#25592=CARTESIAN_POINT('',(-15.3945675730164,-51.2372646541541,14.5));
#25593=CARTESIAN_POINT('',(-15.9724997491699,-50.6012065971864,24.2));
#25594=CARTESIAN_POINT('',(-15.8681814918784,-50.7160167267776,24.2));
#25595=CARTESIAN_POINT('',(-15.9724997491699,-50.6012065971864,14.5));
#25596=CARTESIAN_POINT('Origin',(0.,0.,14.5));
#25597=CARTESIAN_POINT('',(-14.0962798654037,-51.6095426636995,11.5));
#25598=CARTESIAN_POINT('Origin',(0.,0.,11.5));
#25599=CARTESIAN_POINT('',(-14.0962798654037,-51.6095426636995,24.2));
#25600=CARTESIAN_POINT('',(-14.0962798654037,-51.6095426636995,14.5));
#25601=CARTESIAN_POINT('Origin',(0.,0.,24.2));
#25602=CARTESIAN_POINT('Origin',(0.,0.,11.25));
#25603=CARTESIAN_POINT('Ctrl Pts',(-16.0365442723228,-50.5156336969243,
11.));
#25604=CARTESIAN_POINT('Ctrl Pts',(-16.0120367597354,-50.5436377394353,
11.0192759649605));
#25605=CARTESIAN_POINT('Ctrl Pts',(-15.9906779647135,-50.5725991285972,
11.0404458048696));
#25606=CARTESIAN_POINT('Ctrl Pts',(-15.97249974917,-50.6012065971862,11.0622545443403));
#25607=CARTESIAN_POINT('Ctrl Pts',(-14.0962798654037,-51.6095426636995,
11.5));
#25608=CARTESIAN_POINT('Ctrl Pts',(-13.9053251952808,-51.5557194296894,
11.3977655520823));
#25609=CARTESIAN_POINT('Ctrl Pts',(-13.7150950830682,-51.5021004224203,
11.2969997378715));
#25610=CARTESIAN_POINT('Origin',(-13.6826930157773,-51.4929674483533,14.5));
#25611=CARTESIAN_POINT('',(-13.4184131650408,-51.4184764906763,24.2));
#25612=CARTESIAN_POINT('Origin',(19.1972756843392,-49.7011709228329,14.5));
#25613=CARTESIAN_POINT('',(18.9311980867048,-50.0385825039234,24.2));
#25614=CARTESIAN_POINT('',(19.4633532819736,-49.3637593417425,24.2));
#25615=CARTESIAN_POINT('',(19.3672978885042,-49.485566673404,24.2));
#25616=CARTESIAN_POINT('',(18.9311980867048,-50.0385825039234,11.5));
#25617=CARTESIAN_POINT('',(18.9311980867048,-50.0385825039234,14.5));
#25618=CARTESIAN_POINT('',(19.4633532819737,-49.3637593417424,11.0622545443403));
#25619=CARTESIAN_POINT('Ctrl Pts',(18.9311980867048,-50.0385825039234,11.5));
#25620=CARTESIAN_POINT('Ctrl Pts',(19.1983687004362,-49.6997848749554,11.2776618075187));
#25621=CARTESIAN_POINT('Ctrl Pts',(19.4633532819737,-49.3637593417424,11.0622545443403));
#25622=CARTESIAN_POINT('',(19.4633532819736,-49.3637593417425,14.5));
#25623=CARTESIAN_POINT('Origin',(0.,0.,11.25));
#25624=CARTESIAN_POINT('',(17.6620417438945,-50.5005176353365,11.5));
#25625=CARTESIAN_POINT('Origin',(0.,0.,11.5));
#25626=CARTESIAN_POINT('',(17.274290716648,-50.4199272242177,11.2969997378715));
#25627=CARTESIAN_POINT('Ctrl Pts',(17.274290716648,-50.4199272242177,11.2969997378715));
#25628=CARTESIAN_POINT('Ctrl Pts',(17.4677977107421,-50.4601458364523,11.397765552083));
#25629=CARTESIAN_POINT('Ctrl Pts',(17.6620417438945,-50.5005176353365,11.5));
#25630=CARTESIAN_POINT('Ctrl Pts',(17.274290716648,-50.4199272242177,11.2969997378715));
#25631=CARTESIAN_POINT('Ctrl Pts',(17.3085684561035,-50.3043072742572,11.1987310576087));
#25632=CARTESIAN_POINT('Ctrl Pts',(17.3357703360584,-50.1875136980569,11.0971961933879));
#25633=CARTESIAN_POINT('Ctrl Pts',(17.3575602159693,-50.0770916023385,11.));
#25634=CARTESIAN_POINT('Ctrl Pts',(19.4633532819737,-49.3637593417423,11.0622545443403));
#25635=CARTESIAN_POINT('Ctrl Pts',(19.4794916601662,-49.3339535112937,11.0404458048696));
#25636=CARTESIAN_POINT('Ctrl Pts',(19.4987781818543,-49.3035727563959,11.0192759649605));
#25637=CARTESIAN_POINT('Ctrl Pts',(19.5212725321166,-49.2739273726667,11.));
#25638=CARTESIAN_POINT('Origin',(0.,0.,14.5));
#25639=CARTESIAN_POINT('',(17.6620417438945,-50.5005176353365,24.2));
#25640=CARTESIAN_POINT('Origin',(0.,0.,24.2));
#25641=CARTESIAN_POINT('',(17.6620417438945,-50.5005176353365,14.5));
#25642=CARTESIAN_POINT('Origin',(17.2413304950986,-50.4130767515726,14.5));
#25643=CARTESIAN_POINT('',(16.8206192463027,-50.3256358678088,24.2));
#25644=CARTESIAN_POINT('',(16.9724981902626,-50.3572024805937,24.2));
#25645=CARTESIAN_POINT('',(16.8206192463027,-50.3256358678088,11.5));
#25646=CARTESIAN_POINT('',(16.8206192463027,-50.3256358678088,14.5));
#25647=CARTESIAN_POINT('Ctrl Pts',(16.8206192463027,-50.3256358678088,11.5));
#25648=CARTESIAN_POINT('Ctrl Pts',(17.0187290262849,-50.366811125883,11.4654707447276));
#25649=CARTESIAN_POINT('Ctrl Pts',(17.274290716648,-50.4199272242177,11.2969997378715));
#25650=CARTESIAN_POINT('Origin',(15.6835336610932,-50.9192356256702,14.5));
#25651=CARTESIAN_POINT('',(15.3945675730165,-51.2372646541541,24.2));
#25652=CARTESIAN_POINT('',(15.9724997491699,-50.6012065971864,24.2));
#25653=CARTESIAN_POINT('',(15.8681814918784,-50.7160167267776,24.2));
#25654=CARTESIAN_POINT('',(15.3945675730165,-51.2372646541541,11.5));
#25655=CARTESIAN_POINT('',(15.3945675730165,-51.2372646541541,14.5));
#25656=CARTESIAN_POINT('',(15.6608948885133,-50.9441513065986,11.2969997378716));
#25657=CARTESIAN_POINT('Ctrl Pts',(15.3945675730165,-51.2372646541541,11.5));
#25658=CARTESIAN_POINT('Ctrl Pts',(15.527984348901,-51.0904294047295,11.3977655520823));
#25659=CARTESIAN_POINT('Ctrl Pts',(15.6608948885133,-50.9441513065986,11.2969997378716));
#25660=CARTESIAN_POINT('',(15.9724997491699,-50.6012065971864,11.5));
#25661=CARTESIAN_POINT('Ctrl Pts',(15.6608948885133,-50.9441513065986,11.2969997378716));
#25662=CARTESIAN_POINT('Ctrl Pts',(15.8364277798678,-50.7509640877247,11.4654707447277));
#25663=CARTESIAN_POINT('Ctrl Pts',(15.9724997491699,-50.6012065971864,11.5));
#25664=CARTESIAN_POINT('',(15.9724997491699,-50.6012065971864,14.5));
#25665=CARTESIAN_POINT('Origin',(0.,0.,11.25));
#25666=CARTESIAN_POINT('',(14.0962798654032,-51.6095426636996,11.5));
#25667=CARTESIAN_POINT('Origin',(0.,0.,11.5));
#25668=CARTESIAN_POINT('',(13.7150950830682,-51.5021004224204,11.2969997378716));
#25669=CARTESIAN_POINT('Ctrl Pts',(13.7150950830682,-51.5021004224204,11.2969997378716));
#25670=CARTESIAN_POINT('Ctrl Pts',(13.9053251952827,-51.5557194296901,11.3977655520835));
#25671=CARTESIAN_POINT('Ctrl Pts',(14.0962798654032,-51.6095426636996,11.5));
#25672=CARTESIAN_POINT('Ctrl Pts',(13.7150950830682,-51.5021004224204,11.2969997378716));
#25673=CARTESIAN_POINT('Ctrl Pts',(13.7573545636769,-51.3891532110794,11.1987310576087));
#25674=CARTESIAN_POINT('Ctrl Pts',(13.792637289251,-51.2745416453855,11.0971961933879));
#25675=CARTESIAN_POINT('Ctrl Pts',(13.8220767461304,-51.1659085175284,11.));
#25676=CARTESIAN_POINT('Ctrl Pts',(15.6608948885133,-50.9441513065987,11.2969997378716));
#25677=CARTESIAN_POINT('Ctrl Pts',(15.5652039133075,-50.8707607519257,11.1987310576087));
#25678=CARTESIAN_POINT('Ctrl Pts',(15.474547588492,-50.7922616278179,11.0971961933879));
#25679=CARTESIAN_POINT('Ctrl Pts',(15.3920147259482,-50.7157360458881,11.));
#25680=CARTESIAN_POINT('Origin',(0.,0.,14.5));
#25681=CARTESIAN_POINT('',(14.0962798654032,-51.6095426636996,24.2));
#25682=CARTESIAN_POINT('Origin',(0.,0.,24.2));
#25683=CARTESIAN_POINT('',(14.0962798654032,-51.6095426636996,14.5));
#25684=CARTESIAN_POINT('Origin',(13.682693015777,-51.4929674483533,14.5));
#25685=CARTESIAN_POINT('',(13.2691061661508,-51.3763922330071,24.2));
#25686=CARTESIAN_POINT('',(13.4184131650408,-51.4184764906764,24.2));
#25687=CARTESIAN_POINT('',(13.2691061661508,-51.3763922330071,11.5));
#25688=CARTESIAN_POINT('',(13.2691061661508,-51.3763922330071,14.5));
#25689=CARTESIAN_POINT('Ctrl Pts',(13.2691061661508,-51.3763922330071,11.5));
#25690=CARTESIAN_POINT('Ctrl Pts',(13.4638611198572,-51.4312866298879,11.4654707447276));
#25691=CARTESIAN_POINT('Ctrl Pts',(13.7150950830682,-51.5021004224204,11.2969997378716));
#25692=CARTESIAN_POINT('Origin',(12.0933830383532,-51.8892269309232,14.5));
#25693=CARTESIAN_POINT('',(11.7829362735681,-52.1863240013419,24.2));
#25694=CARTESIAN_POINT('',(12.4038298031382,-51.5921298605045,24.2));
#25695=CARTESIAN_POINT('',(12.2917569100881,-51.6993834446145,24.2));
#25696=CARTESIAN_POINT('',(11.7829362735681,-52.1863240013419,11.5));
#25697=CARTESIAN_POINT('',(11.7829362735681,-52.1863240013419,14.5));
#25698=CARTESIAN_POINT('',(12.0690613826431,-51.9125027175599,11.2969997378715));
#25699=CARTESIAN_POINT('Ctrl Pts',(11.7829362735681,-52.1863240013419,11.5));
#25700=CARTESIAN_POINT('Ctrl Pts',(11.9262707621134,-52.049153119029,11.3977655520823));
#25701=CARTESIAN_POINT('Ctrl Pts',(12.0690613826431,-51.9125027175599,11.2969997378715));
#25702=CARTESIAN_POINT('',(12.4038298031382,-51.5921298605045,11.5));
#25703=CARTESIAN_POINT('Ctrl Pts',(12.0690613826431,-51.9125027175599,11.2969997378715));
#25704=CARTESIAN_POINT('Ctrl Pts',(12.2576427438576,-51.7320306485686,11.4654707447276));
#25705=CARTESIAN_POINT('Ctrl Pts',(12.4038298031382,-51.5921298605045,11.5));
#25706=CARTESIAN_POINT('',(12.4038298031382,-51.5921298605045,14.5));
#25707=CARTESIAN_POINT('Origin',(0.,0.,11.25));
#25708=CARTESIAN_POINT('',(10.4618423283611,-52.4671311879782,11.5));
#25709=CARTESIAN_POINT('Origin',(0.,0.,11.5));
#25710=CARTESIAN_POINT('',(10.0890808848802,-52.3333605643381,11.2969997378715));
#25711=CARTESIAN_POINT('Ctrl Pts',(10.0890808848802,-52.3333605643381,11.2969997378715));
#25712=CARTESIAN_POINT('Ctrl Pts',(10.2751073332268,-52.400118740228,11.3977655520819));
#25713=CARTESIAN_POINT('Ctrl Pts',(10.4618423283611,-52.4671311879782,11.5));
#25714=CARTESIAN_POINT('Ctrl Pts',(10.0890808848802,-52.3333605643381,11.2969997378715));
#25715=CARTESIAN_POINT('Ctrl Pts',(10.1391162227005,-52.2236363590767,11.1987310576087));
#25716=CARTESIAN_POINT('Ctrl Pts',(10.1823079000016,-52.1117651799167,11.0971961933879));
#25717=CARTESIAN_POINT('Ctrl Pts',(10.2192535077747,-52.0054502696,11.));
#25718=CARTESIAN_POINT('Ctrl Pts',(12.0690613826431,-51.9125027175599,11.2969997378715));
#25719=CARTESIAN_POINT('Ctrl Pts',(11.9787229721437,-51.8326158735901,11.1987310576086));
#25720=CARTESIAN_POINT('Ctrl Pts',(11.8937633036688,-51.7479841038615,11.0971961933879));
#25721=CARTESIAN_POINT('Ctrl Pts',(11.8167696417768,-51.6658877329441,11.));
#25722=CARTESIAN_POINT('Origin',(0.,0.,14.5));
#25723=CARTESIAN_POINT('',(10.4618423283611,-52.4671311879782,24.2));
#25724=CARTESIAN_POINT('Origin',(0.,0.,24.2));
#25725=CARTESIAN_POINT('',(10.4618423283611,-52.4671311879782,14.5));
#25726=CARTESIAN_POINT('Origin',(10.0573948314623,-52.3219895837806,14.5));
#25727=CARTESIAN_POINT('',(9.65294733456344,-52.176847979583,24.2));
#25728=CARTESIAN_POINT('',(9.79895497969302,-52.2292448518636,24.2));
#25729=CARTESIAN_POINT('',(9.65294733456344,-52.176847979583,11.5));
#25730=CARTESIAN_POINT('',(9.65294733456345,-52.176847979583,14.5));
#25731=CARTESIAN_POINT('Ctrl Pts',(9.65294733456344,-52.176847979583,11.5));
#25732=CARTESIAN_POINT('Ctrl Pts',(9.84339863543623,-52.2451940752868,11.4654707447276));
#25733=CARTESIAN_POINT('Ctrl Pts',(10.0890808848802,-52.3333605643381,11.2969997378715));
#25734=CARTESIAN_POINT('Origin',(8.44431466907313,-52.6064191384554,14.5));
#25735=CARTESIAN_POINT('',(8.11389969301201,-52.8811368237459,24.2));
#25736=CARTESIAN_POINT('',(8.77472964513425,-52.3317014531649,24.2));
#25737=CARTESIAN_POINT('',(8.65544812419492,-52.430875963113,24.2));
#25738=CARTESIAN_POINT('',(8.11389969301201,-52.8811368237459,11.5));
#25739=CARTESIAN_POINT('',(8.11389969301201,-52.8811368237459,14.5));
#25740=CARTESIAN_POINT('',(8.41842862289461,-52.6279416335077,11.2969997378715));
#25741=CARTESIAN_POINT('Ctrl Pts',(8.11389969301201,-52.8811368237459,11.5));
#25742=CARTESIAN_POINT('Ctrl Pts',(8.2664535829971,-52.7542985912954,11.3977655520826));
#25743=CARTESIAN_POINT('Ctrl Pts',(8.41842862289461,-52.6279416335077,11.2969997378715));
#25744=CARTESIAN_POINT('',(8.77472964513425,-52.3317014531649,11.5));
#25745=CARTESIAN_POINT('Ctrl Pts',(8.41842862289461,-52.6279416335077,11.2969997378715));
#25746=CARTESIAN_POINT('Ctrl Pts',(8.61913970453333,-52.4610639561783,11.4654707447276));
#25747=CARTESIAN_POINT('Ctrl Pts',(8.77472964513425,-52.3317014531649,11.5));
#25748=CARTESIAN_POINT('',(8.77472964513425,-52.3317014531649,14.5));
#25749=CARTESIAN_POINT('Origin',(0.,0.,11.25));
#25750=CARTESIAN_POINT('',(6.77643574711564,-53.0691051230866,11.5));
#25751=CARTESIAN_POINT('Origin',(0.,0.,11.5));
#25752=CARTESIAN_POINT('',(6.41391369877197,-52.9096578341174,11.2969997378716));
#25753=CARTESIAN_POINT('Ctrl Pts',(6.41391369877197,-52.9096578341174,11.2969997378716));
#25754=CARTESIAN_POINT('Ctrl Pts',(6.59483018109746,-52.9892299395064,11.3977655520826));
#25755=CARTESIAN_POINT('Ctrl Pts',(6.77643574711564,-53.0691051230866,11.5));
#25756=CARTESIAN_POINT('Ctrl Pts',(6.41391369877197,-52.9096578341174,11.2969997378715));
#25757=CARTESIAN_POINT('Ctrl Pts',(6.47148112666749,-52.8036912002343,11.1987310576087));
#25758=CARTESIAN_POINT('Ctrl Pts',(6.52237133018527,-52.6951054327476,11.0971961933879));
#25759=CARTESIAN_POINT('Ctrl Pts',(6.56664309356484,-52.5916266955277,11.));
#25760=CARTESIAN_POINT('Ctrl Pts',(8.41842862289462,-52.6279416335077,11.2969997378715));
#25761=CARTESIAN_POINT('Ctrl Pts',(8.3338828967566,-52.5419477009146,11.1987310576086));
#25762=CARTESIAN_POINT('Ctrl Pts',(8.2550337995871,-52.4515956030403,11.0971961933879));
#25763=CARTESIAN_POINT('Ctrl Pts',(8.18395444372811,-52.3643284084021,11.));
#25764=CARTESIAN_POINT('Origin',(0.,0.,14.5));
#25765=CARTESIAN_POINT('',(6.77643574711564,-53.0691051230866,24.2));
#25766=CARTESIAN_POINT('Origin',(0.,0.,24.2));
#25767=CARTESIAN_POINT('',(6.77643574711564,-53.0691051230866,14.5));
#25768=CARTESIAN_POINT('Origin',(6.38309803049424,-52.8961042453437,14.5));
#25769=CARTESIAN_POINT('',(5.98976031387283,-52.7231033676009,24.2));
#25770=CARTESIAN_POINT('',(6.13175727067171,-52.785557582198,24.2));
#25771=CARTESIAN_POINT('',(5.98976031387283,-52.7231033676009,11.5));
#25772=CARTESIAN_POINT('',(5.98976031387283,-52.7231033676009,14.5));
#25773=CARTESIAN_POINT('Ctrl Pts',(5.98976031387283,-52.7231033676009,11.5));
#25774=CARTESIAN_POINT('Ctrl Pts',(6.17498010231827,-52.8045681868194,11.4654707447276));
#25775=CARTESIAN_POINT('Ctrl Pts',(6.41391369877197,-52.9096578341174,11.2969997378716));
#25776=CARTESIAN_POINT('Origin',(4.7541064475452,-53.0673181599238,14.5));
#25777=CARTESIAN_POINT('',(4.40533300875834,-53.318318063138,24.2));
#25778=CARTESIAN_POINT('',(5.10287988633206,-52.8163182567096,24.2));
#25779=CARTESIAN_POINT('',(4.97697086508333,-52.9069305242526,24.2));
#25780=CARTESIAN_POINT('',(4.40533300875834,-53.318318063138,11.5));
#25781=CARTESIAN_POINT('',(4.40533300875834,-53.318318063138,14.5));
#25782=CARTESIAN_POINT('',(4.72678212511292,-53.0869825079595,11.2969997378716));
#25783=CARTESIAN_POINT('Ctrl Pts',(4.40533300875834,-53.318318063138,11.5));
#25784=CARTESIAN_POINT('Ctrl Pts',(4.5663630729665,-53.202430423668,11.3977655520825));
#25785=CARTESIAN_POINT('Ctrl Pts',(4.72678212511292,-53.0869825079595,11.2969997378716));
#25786=CARTESIAN_POINT('',(5.10287988633206,-52.8163182567096,11.5));
#25787=CARTESIAN_POINT('Ctrl Pts',(4.72678212511292,-53.0869825079595,11.2969997378716));
#25788=CARTESIAN_POINT('Ctrl Pts',(4.93864508296159,-52.9345122335611,11.4654707447277));
#25789=CARTESIAN_POINT('Ctrl Pts',(5.10287988633206,-52.8163182567096,11.5));
#25790=CARTESIAN_POINT('',(5.10287988633206,-52.8163182567096,14.5));
#25791=CARTESIAN_POINT('Origin',(0.,0.,11.25));
#25792=CARTESIAN_POINT('',(3.05801505207583,-53.412531712523,11.5));
#25793=CARTESIAN_POINT('Origin',(0.,0.,11.5));
#25794=CARTESIAN_POINT('',(2.29739178302173,-53.0124970957196,11.0622545443403));
#25795=CARTESIAN_POINT('Ctrl Pts',(2.29739178302173,-53.0124970957196,11.0622545443403));
#25796=CARTESIAN_POINT('Ctrl Pts',(2.67614114119987,-53.2116927560781,11.27766180752));
#25797=CARTESIAN_POINT('Ctrl Pts',(3.05801505207583,-53.412531712523,11.5));
#25798=CARTESIAN_POINT('Ctrl Pts',(2.2079419616008,-52.953989389792,11.));
#25799=CARTESIAN_POINT('Ctrl Pts',(2.2405494369663,-52.9719225189241,11.0192759649605));
#25800=CARTESIAN_POINT('Ctrl Pts',(2.2705255175094,-52.9918321844726,11.0404458048696));
#25801=CARTESIAN_POINT('Ctrl Pts',(2.2973917830217,-53.0124970957195,11.0622545443404));
#25802=CARTESIAN_POINT('Ctrl Pts',(4.51126784227785,-52.8076553394982,11.));
#25803=CARTESIAN_POINT('Ctrl Pts',(4.57608660062692,-52.8996682008571,11.0971961933879));
#25804=CARTESIAN_POINT('Ctrl Pts',(4.64844098161559,-52.9953004405386,11.1987310576087));
#25805=CARTESIAN_POINT('Ctrl Pts',(4.72678212511292,-53.0869825079595,11.2969997378716));
#25806=CARTESIAN_POINT('Origin',(0.,0.,14.5));
#25807=CARTESIAN_POINT('',(3.05801505207583,-53.412531712523,24.2));
#25808=CARTESIAN_POINT('Origin',(0.,0.,24.2));
#25809=CARTESIAN_POINT('',(3.05801505207583,-53.412531712523,14.5));
#25810=CARTESIAN_POINT('Origin',(1.04073669728542,-53.2696785416253,14.5));
#25811=CARTESIAN_POINT('',(1.4061694096632,-53.0436192667856,11.0622545443405));
#25812=CARTESIAN_POINT('',(1.4061694096632,-53.0436192667856,24.2));
#25813=CARTESIAN_POINT('',(1.4061694096632,-53.0436192667856,14.5));
#25814=CARTESIAN_POINT('',(0.675303984907634,-53.495737816465,24.2));
#25815=CARTESIAN_POINT('',(1.27424630420039,-53.1252278380639,24.2));
#25816=CARTESIAN_POINT('',(0.675303984907639,-53.495737816465,11.5));
#25817=CARTESIAN_POINT('',(0.675303984907634,-53.495737816465,14.5));
#25818=CARTESIAN_POINT('Ctrl Pts',(0.675303984907627,-53.495737816465,11.5));
#25819=CARTESIAN_POINT('Ctrl Pts',(0.918332026570836,-53.3453989414732,
11.3527407245756));
#25820=CARTESIAN_POINT('Ctrl Pts',(1.16196424828666,-53.1946863164038,11.2067970124651));
#25821=CARTESIAN_POINT('Ctrl Pts',(1.4061694096632,-53.0436192667856,11.0622545443405));
#25822=CARTESIAN_POINT('Origin',(0.,0.,11.25));
#25823=CARTESIAN_POINT('Ctrl Pts',(1.49132004456263,-52.9790143785696,11.));
#25824=CARTESIAN_POINT('Ctrl Pts',(1.46004329008757,-52.999178187535,11.0192757561174));
#25825=CARTESIAN_POINT('Ctrl Pts',(1.43152846249062,-53.0211308257202,11.0404460254343));
#25826=CARTESIAN_POINT('Ctrl Pts',(1.4061694096632,-53.0436192667856,11.0622545443405));
#25827=CARTESIAN_POINT('Origin',(0.,0.,11.5));
#25828=CARTESIAN_POINT('Origin',(0.,0.,11.25));
#25829=CARTESIAN_POINT('Origin',(0.,0.,11.5));
#25830=CARTESIAN_POINT('Origin',(0.,0.,11.25));
#25831=CARTESIAN_POINT('Origin',(0.,0.,11.5));
#25832=CARTESIAN_POINT('Origin',(0.,0.,14.5));
#25833=CARTESIAN_POINT('Origin',(0.,0.,24.2));
#25834=CARTESIAN_POINT('Origin',(0.,0.,14.5));
#25835=CARTESIAN_POINT('Origin',(0.,0.,24.2));
#25836=CARTESIAN_POINT('Origin',(0.,0.,14.5));
#25837=CARTESIAN_POINT('Origin',(0.,0.,24.2));
#25838=CARTESIAN_POINT('Origin',(0.,0.,14.5));
#25839=CARTESIAN_POINT('Origin',(0.,0.,24.2));
#25840=CARTESIAN_POINT('Origin',(2.67770341754884,-53.2125144041213,14.5));
#25841=CARTESIAN_POINT('',(2.29739178302185,-53.0124970957197,24.2));
#25842=CARTESIAN_POINT('',(2.43468625658986,-53.0847043819776,24.2));
#25843=CARTESIAN_POINT('',(2.29739178302185,-53.0124970957197,14.5));
#25844=CARTESIAN_POINT('Origin',(16.5633108984972,-50.9766292734202,11.25));
#25845=CARTESIAN_POINT('Origin',(16.5633108984972,-50.9766292734202,11.5));
#25846=CARTESIAN_POINT('Origin',(12.9670136041422,-52.0078509283934,11.25));
#25847=CARTESIAN_POINT('Origin',(12.9670136041422,-52.0078509283934,11.5));
#25848=CARTESIAN_POINT('Origin',(9.30754232294745,-52.7856955614544,11.25));
#25849=CARTESIAN_POINT('Origin',(9.30754232294745,-52.7856955614544,11.5));
#25850=CARTESIAN_POINT('Origin',(5.6027256311462,-53.3063735917395,11.25));
#25851=CARTESIAN_POINT('Origin',(5.6027256311462,-53.3063735917395,11.5));
#25852=CARTESIAN_POINT('Origin',(1.87061302325407,-53.5673483282235,11.));
#25853=CARTESIAN_POINT('Origin',(1.87061302325407,-53.5673483282235,24.2));
#25854=CARTESIAN_POINT('Origin',(5.6027256311462,-53.3063735917395,11.));
#25855=CARTESIAN_POINT('Origin',(5.6027256311462,-53.3063735917395,24.2));
#25856=CARTESIAN_POINT('Origin',(9.30754232294745,-52.7856955614544,11.));
#25857=CARTESIAN_POINT('Origin',(9.30754232294745,-52.7856955614544,24.2));
#25858=CARTESIAN_POINT('Origin',(12.9670136041422,-52.0078509283934,11.));
#25859=CARTESIAN_POINT('Origin',(12.9670136041422,-52.0078509283934,24.2));
#25860=CARTESIAN_POINT('Origin',(16.5633108984972,-50.9766292734202,11.));
#25861=CARTESIAN_POINT('Origin',(16.5633108984972,-50.9766292734202,24.2));
#25862=CARTESIAN_POINT('Origin',(36.2555847625696,-39.0419563844501,14.5));
#25863=CARTESIAN_POINT('',(36.2884817614959,-39.0348084727496,11.2969997378715));
#25864=CARTESIAN_POINT('',(36.675489024416,-38.9507189255852,11.5));
#25865=CARTESIAN_POINT('Ctrl Pts',(36.2884817614959,-39.0348084727496,11.2969997378715));
#25866=CARTESIAN_POINT('Ctrl Pts',(36.4816175803015,-38.9928436180799,11.3977655520826));
#25867=CARTESIAN_POINT('Ctrl Pts',(36.675489024416,-38.9507189255852,11.5));
#25868=CARTESIAN_POINT('',(36.675489024416,-38.9507189255852,24.2));
#25869=CARTESIAN_POINT('',(36.675489024416,-38.9507189255852,14.5));
#25870=CARTESIAN_POINT('',(35.8356805007233,-39.1331938433149,24.2));
#25871=CARTESIAN_POINT('',(35.9872681182067,-39.1002566472175,24.2));
#25872=CARTESIAN_POINT('',(35.8356805007233,-39.1331938433149,11.5));
#25873=CARTESIAN_POINT('',(35.8356805007233,-39.1331938433149,14.5));
#25874=CARTESIAN_POINT('Ctrl Pts',(35.8356805007233,-39.1331938433149,11.5));
#25875=CARTESIAN_POINT('Ctrl Pts',(36.0334102765875,-39.0902308064254,11.4654707447276));
#25876=CARTESIAN_POINT('Ctrl Pts',(36.2884817614959,-39.0348084727496,11.2969997378715));
#25877=CARTESIAN_POINT('Origin',(35.8654005008348,-39.8325626455884,11.25));
#25878=CARTESIAN_POINT('',(35.1729694999763,-39.7299015085881,11.5));
#25879=CARTESIAN_POINT('Origin',(35.8654005008348,-39.8325626455884,11.5));
#25880=CARTESIAN_POINT('',(35.027792474811,-40.1699382050837,11.2969997378715));
#25881=CARTESIAN_POINT('Ctrl Pts',(35.027792474811,-40.1699382050837,11.2969997378715));
#25882=CARTESIAN_POINT('Ctrl Pts',(35.1095734294849,-39.922057239828,11.4654707447276));
#25883=CARTESIAN_POINT('Ctrl Pts',(35.1729694999763,-39.7299015085881,11.5));
#25884=CARTESIAN_POINT('Ctrl Pts',(35.027792474811,-40.1699382050837,11.2969997378715));
#25885=CARTESIAN_POINT('Ctrl Pts',(34.9105237912332,-40.1418136232562,11.1987310576086));
#25886=CARTESIAN_POINT('Ctrl Pts',(34.7957766472675,-40.1069743542277,11.0971961933879));
#25887=CARTESIAN_POINT('Ctrl Pts',(34.6892533672809,-40.0706338959167,11.));
#25888=CARTESIAN_POINT('Ctrl Pts',(36.2884817614959,-39.0348084727496,11.2969997378715));
#25889=CARTESIAN_POINT('Ctrl Pts',(36.2727691643543,-38.9152423799721,11.1987310576086));
#25890=CARTESIAN_POINT('Ctrl Pts',(36.2501150911098,-38.7974821376142,11.0971961933879));
#25891=CARTESIAN_POINT('Ctrl Pts',(36.2251084243911,-38.6877437910394,11.));
#25892=CARTESIAN_POINT('Origin',(35.8654005008348,-39.8325626455884,11.));
#25893=CARTESIAN_POINT('',(35.1729694999763,-39.7299015085881,24.2));
#25894=CARTESIAN_POINT('Origin',(35.8654005008348,-39.8325626455884,24.2));
#25895=CARTESIAN_POINT('',(35.1729694999763,-39.7299015085881,14.5));
#25896=CARTESIAN_POINT('Origin',(35.0383399022471,-40.1379685795852,14.5));
#25897=CARTESIAN_POINT('',(34.9037103045179,-40.5460356505823,24.2));
#25898=CARTESIAN_POINT('',(35.1243675165795,-39.8772158387497,24.2));
#25899=CARTESIAN_POINT('',(34.9037103045179,-40.5460356505823,11.5));
#25900=CARTESIAN_POINT('',(34.9037103045179,-40.5460356505823,14.5));
#25901=CARTESIAN_POINT('Ctrl Pts',(34.9037103045179,-40.5460356505823,11.5));
#25902=CARTESIAN_POINT('Ctrl Pts',(34.9658693176641,-40.3576294838963,11.3977655520828));
#25903=CARTESIAN_POINT('Ctrl Pts',(35.027792474811,-40.1699382050837,11.2969997378715));
#25904=CARTESIAN_POINT('Origin',(33.443838774836,-41.4759138875076,14.5));
#25905=CARTESIAN_POINT('',(33.4771542514414,-41.4710781664026,11.2969997378715));
#25906=CARTESIAN_POINT('',(33.8690845744086,-41.4141897191236,11.5));
#25907=CARTESIAN_POINT('Ctrl Pts',(33.4771542514414,-41.4710781664026,11.2969997378715));
#25908=CARTESIAN_POINT('Ctrl Pts',(33.6727469213824,-41.4426880096833,11.3977655520828));
#25909=CARTESIAN_POINT('Ctrl Pts',(33.8690845744086,-41.4141897191236,11.5));
#25910=CARTESIAN_POINT('',(33.8690845744086,-41.4141897191236,24.2));
#25911=CARTESIAN_POINT('',(33.8690845744086,-41.4141897191236,14.5));
#25912=CARTESIAN_POINT('',(33.0185929752635,-41.5376380558916,24.2));
#25913=CARTESIAN_POINT('',(33.1721089155843,-41.5153553108074,24.2));
#25914=CARTESIAN_POINT('',(33.0185929752635,-41.5376380558916,11.5));
#25915=CARTESIAN_POINT('',(33.0185929752635,-41.5376380558916,14.5));
#25916=CARTESIAN_POINT('Ctrl Pts',(33.0185929752635,-41.5376380558916,11.5));
#25917=CARTESIAN_POINT('Ctrl Pts',(33.2188380412863,-41.5085726067192,11.4654707447276));
#25918=CARTESIAN_POINT('Ctrl Pts',(33.4771542514414,-41.4710781664026,11.2969997378715));
#25919=CARTESIAN_POINT('Origin',(32.9994550774553,-42.2373763933203,11.25));
#25920=CARTESIAN_POINT('',(32.3158720826212,-42.0866637887591,11.5));
#25921=CARTESIAN_POINT('Origin',(32.9994550774553,-42.2373763933203,11.5));
#25922=CARTESIAN_POINT('',(32.140353293127,-42.5155015406339,11.2969997378715));
#25923=CARTESIAN_POINT('Ctrl Pts',(32.140353293127,-42.5155015406339,11.2969997378715));
#25924=CARTESIAN_POINT('Ctrl Pts',(32.2392263355501,-42.2739291519686,11.4654707447276));
#25925=CARTESIAN_POINT('Ctrl Pts',(32.3158720826212,-42.0866637887591,11.5));
#25926=CARTESIAN_POINT('Ctrl Pts',(32.140353293127,-42.5155015406339,11.2969997378715));
#25927=CARTESIAN_POINT('Ctrl Pts',(32.0253321418224,-42.4792652190273,11.1987310576086));
#25928=CARTESIAN_POINT('Ctrl Pts',(31.9132947806875,-42.4365064605718,11.0971961933879));
#25929=CARTESIAN_POINT('Ctrl Pts',(31.809565968283,-42.3928238374073,11.));
#25930=CARTESIAN_POINT('Ctrl Pts',(33.4771542514414,-41.4710781664026,11.2969997378715));
#25931=CARTESIAN_POINT('Ctrl Pts',(33.4698204384081,-41.3507072752477,11.1987310576086));
#25932=CARTESIAN_POINT('Ctrl Pts',(33.4554360886017,-41.2316536226561,11.0971961933879));
#25933=CARTESIAN_POINT('Ctrl Pts',(33.4381452969578,-41.1204382162877,11.));
#25934=CARTESIAN_POINT('Origin',(32.9994550774553,-42.2373763933203,11.));
#25935=CARTESIAN_POINT('',(32.3158720826212,-42.0866637887591,24.2));
#25936=CARTESIAN_POINT('Origin',(32.9994550774553,-42.2373763933203,24.2));
#25937=CARTESIAN_POINT('',(32.3158720826212,-42.0866637887591,14.5));
#25938=CARTESIAN_POINT('Origin',(32.1531051159017,-42.4843455428814,14.5));
#25939=CARTESIAN_POINT('',(31.9903381491823,-42.8820272970037,24.2));
#25940=CARTESIAN_POINT('',(32.2571123630091,-42.2302289656376,24.2));
#25941=CARTESIAN_POINT('',(31.9903381491823,-42.8820272970037,11.5));
#25942=CARTESIAN_POINT('',(31.9903381491823,-42.8820272970037,14.5));
#25943=CARTESIAN_POINT('Ctrl Pts',(31.9903381491823,-42.8820272970037,11.5));
#25944=CARTESIAN_POINT('Ctrl Pts',(32.0654882959157,-42.6984160718402,11.3977655520835));
#25945=CARTESIAN_POINT('Ctrl Pts',(32.140353293127,-42.5155015406339,11.2969997378715));
#25946=CARTESIAN_POINT('Origin',(30.4691577663546,-43.7078049072493,14.5));
#25947=CARTESIAN_POINT('',(30.5027294109855,-43.705304935887,11.2969997378715));
#25948=CARTESIAN_POINT('',(30.8976733488635,-43.6758947432898,11.5));
#25949=CARTESIAN_POINT('Ctrl Pts',(30.5027294109855,-43.705304935887,11.2969997378715));
#25950=CARTESIAN_POINT('Ctrl Pts',(30.699826024235,-43.6906277911077,11.3977655520828));
#25951=CARTESIAN_POINT('Ctrl Pts',(30.8976733488635,-43.6758947432898,11.5));
#25952=CARTESIAN_POINT('',(30.8976733488635,-43.6758947432898,24.2));
#25953=CARTESIAN_POINT('',(30.8976733488635,-43.6758947432898,14.5));
#25954=CARTESIAN_POINT('',(30.0406421838458,-43.7397150712088,24.2));
#25955=CARTESIAN_POINT('',(30.195338532774,-43.728195336432,24.2));
#25956=CARTESIAN_POINT('',(30.0406421838458,-43.7397150712088,11.5));
#25957=CARTESIAN_POINT('',(30.0406421838458,-43.7397150712088,14.5));
#25958=CARTESIAN_POINT('Ctrl Pts',(30.0406421838458,-43.7397150712088,11.5));
#25959=CARTESIAN_POINT('Ctrl Pts',(30.242426966194,-43.7246888137001,11.4654707447276));
#25960=CARTESIAN_POINT('Ctrl Pts',(30.5027294109855,-43.705304935887,11.2969997378715));
#25961=CARTESIAN_POINT('Origin',(29.972739626032,-44.4364138889502,11.25));
#25962=CARTESIAN_POINT('',(29.3013349848596,-44.2383840734879,11.5));
#25963=CARTESIAN_POINT('Origin',(29.972739626032,-44.4364138889502,11.5));
#25964=CARTESIAN_POINT('',(29.0963295409359,-44.6539336263215,11.2969997378715));
#25965=CARTESIAN_POINT('Ctrl Pts',(29.0963295409359,-44.6539336263215,11.2969997378715));
#25966=CARTESIAN_POINT('Ctrl Pts',(29.2118129715843,-44.4198467306414,11.4654707447276));
#25967=CARTESIAN_POINT('Ctrl Pts',(29.3013349848596,-44.2383840734879,11.5));
#25968=CARTESIAN_POINT('Ctrl Pts',(29.0963295409359,-44.6539336263215,11.2969997378715));
#25969=CARTESIAN_POINT('Ctrl Pts',(28.9841162933917,-44.609762104652,11.1987310576086));
#25970=CARTESIAN_POINT('Ctrl Pts',(28.875334549849,-44.5592921731428,11.0971961933879));
#25971=CARTESIAN_POINT('Ctrl Pts',(28.774905561374,-44.5084802024738,11.));
#25972=CARTESIAN_POINT('Ctrl Pts',(30.5027294109855,-43.705304935887,11.2969997378715));
#25973=CARTESIAN_POINT('Ctrl Pts',(30.5038101116606,-43.5847156812369,11.1987310576087));
#25974=CARTESIAN_POINT('Ctrl Pts',(30.4977655643985,-43.4649486358399,11.0971961933879));
#25975=CARTESIAN_POINT('Ctrl Pts',(30.4882748868283,-43.3527979999583,11.));
#25976=CARTESIAN_POINT('Origin',(29.972739626032,-44.4364138889502,11.));
#25977=CARTESIAN_POINT('',(29.3013349848596,-44.2383840734879,24.2));
#25978=CARTESIAN_POINT('Origin',(29.972739626032,-44.4364138889502,24.2));
#25979=CARTESIAN_POINT('',(29.3013349848596,-44.2383840734879,14.5));
#25980=CARTESIAN_POINT('Origin',(29.1112236334505,-44.6237430452042,14.5));
#25981=CARTESIAN_POINT('',(28.9211122820414,-45.0091020169205,24.2));
#25982=CARTESIAN_POINT('',(29.2327038004797,-44.3775006619728,24.2));
#25983=CARTESIAN_POINT('',(28.9211122820414,-45.0091020169205,11.5));
#25984=CARTESIAN_POINT('',(28.9211122820413,-45.0091020169205,14.5));
#25985=CARTESIAN_POINT('Ctrl Pts',(28.9211122820414,-45.0091020169205,11.5));
#25986=CARTESIAN_POINT('Ctrl Pts',(29.0088874384019,-44.8311802687101,11.3977655520831));
#25987=CARTESIAN_POINT('Ctrl Pts',(29.0963295409359,-44.6539336263215,11.2969997378715));
#25988=CARTESIAN_POINT('Origin',(27.3460340839842,-45.7267558949762,14.5));
#25989=CARTESIAN_POINT('',(27.379698338963,-45.7266038529658,11.2969997378715));
#25990=CARTESIAN_POINT('',(27.7757317645856,-45.7248151985527,11.5));
#25991=CARTESIAN_POINT('Ctrl Pts',(27.379698338963,-45.7266038529658,11.2969997378715));
#25992=CARTESIAN_POINT('Ctrl Pts',(27.5773386606333,-45.7257112257007,11.397765552083));
#25993=CARTESIAN_POINT('Ctrl Pts',(27.7757317645856,-45.7248151985527,11.5));
#25994=CARTESIAN_POINT('',(27.7757317645856,-45.7248151985527,24.2));
#25995=CARTESIAN_POINT('',(27.7757317645856,-45.7248151985527,14.5));
#25996=CARTESIAN_POINT('',(26.9163364033829,-45.7286965913998,24.2));
#25997=CARTESIAN_POINT('',(27.0714594958567,-45.7279959899203,24.2));
#25998=CARTESIAN_POINT('',(26.9163364033829,-45.7286965913998,11.5));
#25999=CARTESIAN_POINT('',(26.9163364033829,-45.7286965913998,14.5));
#26000=CARTESIAN_POINT('Ctrl Pts',(26.9163364033829,-45.7286965913998,11.5));
#26001=CARTESIAN_POINT('Ctrl Pts',(27.1186778268805,-45.727782731971,11.4654707447276));
#26002=CARTESIAN_POINT('Ctrl Pts',(27.379698338963,-45.7266038529658,11.2969997378715));
#26003=CARTESIAN_POINT('Origin',(26.8,-46.4189616428459,11.25));
#26004=CARTESIAN_POINT('',(26.1440447284116,-46.1745793978374,11.5));
#26005=CARTESIAN_POINT('Origin',(26.8,-46.4189616428459,11.5));
#26006=CARTESIAN_POINT('',(25.9105513959743,-46.5748162359794,11.2969997378715));
#26007=CARTESIAN_POINT('Ctrl Pts',(25.9105513959743,-46.5748162359794,11.2969997378715));
#26008=CARTESIAN_POINT('Ctrl Pts',(26.042082591182,-46.3493552811098,11.4654707447276));
#26009=CARTESIAN_POINT('Ctrl Pts',(26.1440447284116,-46.1745793978374,11.5));
#26010=CARTESIAN_POINT('Ctrl Pts',(25.9105513959743,-46.5748162359794,11.2969997378715));
#26011=CARTESIAN_POINT('Ctrl Pts',(25.8016927438527,-46.5229247134606,11.1987310576087));
#26012=CARTESIAN_POINT('Ctrl Pts',(25.6966965916221,-46.4649894933306,11.0971961933879));
#26013=CARTESIAN_POINT('Ctrl Pts',(25.6000567070134,-46.4072957259707,11.));
#26014=CARTESIAN_POINT('Ctrl Pts',(27.379698338963,-45.7266038529658,11.2969997378715));
#26015=CARTESIAN_POINT('Ctrl Pts',(27.3891882882814,-45.6063837335474,11.1987310576087));
#26016=CARTESIAN_POINT('Ctrl Pts',(27.3915129919902,-45.4864867883511,11.0971961933879));
#26017=CARTESIAN_POINT('Ctrl Pts',(27.3898686661209,-45.3739473095812,11.));
#26018=CARTESIAN_POINT('Origin',(26.8,-46.4189616428459,11.));
#26019=CARTESIAN_POINT('',(26.1440447284116,-46.1745793978374,24.2));
#26020=CARTESIAN_POINT('Origin',(26.8,-46.4189616428459,24.2));
#26021=CARTESIAN_POINT('',(26.1440447284116,-46.1745793978374,14.5));
#26022=CARTESIAN_POINT('Origin',(25.9275151957071,-46.5457381569736,14.5));
#26023=CARTESIAN_POINT('',(25.7109856630026,-46.9168969161098,24.2));
#26024=CARTESIAN_POINT('',(26.0658764434955,-46.3085696358935,24.2));
#26025=CARTESIAN_POINT('',(25.7109856630026,-46.9168969161098,11.5));
#26026=CARTESIAN_POINT('',(25.7109856630026,-46.9168969161098,14.5));
#26027=CARTESIAN_POINT('Ctrl Pts',(25.7109856630026,-46.9168969161098,11.5));
#26028=CARTESIAN_POINT('Ctrl Pts',(25.8109581972526,-46.7455314617236,11.3977655520818));
#26029=CARTESIAN_POINT('Ctrl Pts',(25.9105513959743,-46.5748162359794,11.2969997378715));
#26030=CARTESIAN_POINT('Origin',(24.0896832723706,-47.5229307244202,14.5));
#26031=CARTESIAN_POINT('',(24.1232761288306,-47.525127352495,11.2969997378715));
#26032=CARTESIAN_POINT('',(24.5184696071576,-47.5509689504103,11.5));
#26033=CARTESIAN_POINT('Ctrl Pts',(24.1232761288306,-47.525127352495,11.2969997378715));
#26034=CARTESIAN_POINT('Ctrl Pts',(24.3204972751414,-47.5380235915345,11.3977655520831));
#26035=CARTESIAN_POINT('Ctrl Pts',(24.5184696071576,-47.5509689504103,11.5));
#26036=CARTESIAN_POINT('',(24.5184696071576,-47.5509689504103,24.2));
#26037=CARTESIAN_POINT('',(24.5184696071576,-47.5509689504103,14.5));
#26038=CARTESIAN_POINT('',(23.6608969375836,-47.49489249843,24.2));
#26039=CARTESIAN_POINT('',(23.8156910294893,-47.5050144435077,24.2));
#26040=CARTESIAN_POINT('',(23.6608969375836,-47.49489249843,11.5));
#26041=CARTESIAN_POINT('',(23.6608969375836,-47.49489249843,14.5));
#26042=CARTESIAN_POINT('Ctrl Pts',(23.6608969375836,-47.49489249843,11.5));
#26043=CARTESIAN_POINT('Ctrl Pts',(23.8628092151544,-47.5080954893125,11.4654707447276));
#26044=CARTESIAN_POINT('Ctrl Pts',(24.1232761288306,-47.525127352495,11.2969997378715));
#26045=CARTESIAN_POINT('Origin',(23.4966934678945,-48.1753608816354,11.25));
#26046=CARTESIAN_POINT('',(22.859383314037,-47.8858168128132,11.5));
#26047=CARTESIAN_POINT('Origin',(23.4966934678945,-48.1753608816354,11.5));
#26048=CARTESIAN_POINT('',(22.5985396491308,-48.2687910226197,11.2969997378715));
#26049=CARTESIAN_POINT('Ctrl Pts',(22.5985396491308,-48.2687910226197,11.2969997378715));
#26050=CARTESIAN_POINT('Ctrl Pts',(22.7454778021365,-48.0530544316696,11.4654707447276));
#26051=CARTESIAN_POINT('Ctrl Pts',(22.859383314037,-47.8858168128132,11.5));
#26052=CARTESIAN_POINT('Ctrl Pts',(22.5985396491308,-48.2687910226197,11.2969997378715));
#26053=CARTESIAN_POINT('Ctrl Pts',(22.4935659408428,-48.2094323095332,11.1987310576086));
#26054=CARTESIAN_POINT('Ctrl Pts',(22.3928669106238,-48.1443140553513,11.0971961933879));
#26055=CARTESIAN_POINT('Ctrl Pts',(22.300486949685,-48.0800195695356,11.));
#26056=CARTESIAN_POINT('Ctrl Pts',(24.1232761288306,-47.525127352495,11.2969997378715));
#26057=CARTESIAN_POINT('Ctrl Pts',(24.1411290927132,-47.4058620686457,11.1987310576087));
#26058=CARTESIAN_POINT('Ctrl Pts',(24.1518117216703,-47.2864193495151,11.0971961933879));
#26059=CARTESIAN_POINT('Ctrl Pts',(24.1580217584921,-47.174039308885,11.));
#26060=CARTESIAN_POINT('Origin',(23.4966934678945,-48.1753608816354,11.));
#26061=CARTESIAN_POINT('',(22.859383314037,-47.8858168128132,24.2));
#26062=CARTESIAN_POINT('Origin',(23.4966934678945,-48.1753608816354,24.2));
#26063=CARTESIAN_POINT('',(22.859383314037,-47.8858168128132,14.5));
#26064=CARTESIAN_POINT('Origin',(20.7159699453406,-49.087578612363,14.5));
#26065=CARTESIAN_POINT('',(20.2901839602893,-49.0296980633778,11.0622545443403));
#26066=CARTESIAN_POINT('',(21.1417559303918,-49.1454591613482,11.5));
#26067=CARTESIAN_POINT('Ctrl Pts',(20.2901839602893,-49.0296980633778,11.0622545443403));
#26068=CARTESIAN_POINT('Ctrl Pts',(20.7142208656047,-49.0873408457411,11.2776618075212));
#26069=CARTESIAN_POINT('Ctrl Pts',(21.1417559303918,-49.1454591613482,11.5));
#26070=CARTESIAN_POINT('',(21.1417559303918,-49.1454591613482,24.2));
#26071=CARTESIAN_POINT('',(21.1417559303918,-49.1454591613482,14.5));
#26072=CARTESIAN_POINT('',(20.2901839602894,-49.0296980633778,24.2));
#26073=CARTESIAN_POINT('',(20.4438949103711,-49.0505932419138,24.2));
#26074=CARTESIAN_POINT('',(20.2901839602894,-49.0296980633778,14.5));
#26075=CARTESIAN_POINT('Origin',(0.,0.,14.5));
#26076=CARTESIAN_POINT('',(22.3755977062724,-48.5961174095941,11.5));
#26077=CARTESIAN_POINT('Origin',(0.,0.,11.5));
#26078=CARTESIAN_POINT('',(22.3755977062724,-48.5961174095941,24.2));
#26079=CARTESIAN_POINT('',(22.3755977062724,-48.5961174095941,14.5));
#26080=CARTESIAN_POINT('Origin',(0.,0.,24.2));
#26081=CARTESIAN_POINT('Origin',(0.,0.,11.25));
#26082=CARTESIAN_POINT('Ctrl Pts',(20.1861178092024,-49.0053124446014,11.));
#26083=CARTESIAN_POINT('Ctrl Pts',(20.2228923045819,-49.0110116603164,11.0192759649605));
#26084=CARTESIAN_POINT('Ctrl Pts',(20.2578701129328,-49.019468202751,11.0404458048696));
#26085=CARTESIAN_POINT('Ctrl Pts',(20.2901839602893,-49.0296980633778,11.0622545443404));
#26086=CARTESIAN_POINT('Ctrl Pts',(22.3755977062724,-48.5961174095941,11.5));
#26087=CARTESIAN_POINT('Ctrl Pts',(22.4872805622719,-48.4321431243045,11.397765552083));
#26088=CARTESIAN_POINT('Ctrl Pts',(22.5985396491308,-48.2687910226197,11.2969997378715));
#26089=CARTESIAN_POINT('Origin',(22.6174905101547,-48.2409671112037,14.5));
#26090=CARTESIAN_POINT('',(22.7720587566113,-48.0140279134694,24.2));
#26091=CARTESIAN_POINT('Origin',(46.653263217121,-25.7335348523128,14.5));
#26092=CARTESIAN_POINT('',(46.6663199357044,-26.1630385020257,24.2));
#26093=CARTESIAN_POINT('',(46.6402064985376,-25.3040312025999,24.2));
#26094=CARTESIAN_POINT('',(46.6449200416998,-25.459084248916,24.2));
#26095=CARTESIAN_POINT('',(46.6663199357044,-26.1630385020257,11.5));
#26096=CARTESIAN_POINT('',(46.6663199357044,-26.1630385020257,14.5));
#26097=CARTESIAN_POINT('',(46.6402064985376,-25.3040312025998,11.0622545443403));
#26098=CARTESIAN_POINT('Ctrl Pts',(46.6663199357044,-26.1630385020257,11.5));
#26099=CARTESIAN_POINT('Ctrl Pts',(46.6532095816264,-25.7317705008368,11.2776618075201));
#26100=CARTESIAN_POINT('Ctrl Pts',(46.6402064985376,-25.3040312025998,11.0622545443403));
#26101=CARTESIAN_POINT('',(46.6402064985376,-25.3040312025999,14.5));
#26102=CARTESIAN_POINT('Origin',(0.,0.,11.25));
#26103=CARTESIAN_POINT('',(45.9910159507966,-27.3326993144397,11.5));
#26104=CARTESIAN_POINT('Origin',(0.,0.,11.5));
#26105=CARTESIAN_POINT('',(45.6421789133341,-27.5202050337907,11.2969997378715));
#26106=CARTESIAN_POINT('Ctrl Pts',(45.6421789133341,-27.5202050337907,11.2969997378715));
#26107=CARTESIAN_POINT('Ctrl Pts',(45.8162658964866,-27.4266303800122,11.3977655520824));
#26108=CARTESIAN_POINT('Ctrl Pts',(45.9910159507966,-27.3326993144397,11.5));
#26109=CARTESIAN_POINT('Ctrl Pts',(45.6421789133341,-27.5202050337907,11.2969997378715));
#26110=CARTESIAN_POINT('Ctrl Pts',(45.5941181138995,-27.4096017073998,11.1987310576087));
#26111=CARTESIAN_POINT('Ctrl Pts',(45.5398824992088,-27.3026476059644,11.097196193388));
#26112=CARTESIAN_POINT('Ctrl Pts',(45.4855965606673,-27.2040531083184,11.));
#26113=CARTESIAN_POINT('Ctrl Pts',(46.6402064985376,-25.3040312025997,11.0622545443404));
#26114=CARTESIAN_POINT('Ctrl Pts',(46.6334103949641,-25.2708250622694,11.0404458048696));
#26115=CARTESIAN_POINT('Ctrl Pts',(46.6286563549092,-25.2351549166271,11.0192759649605));
#26116=CARTESIAN_POINT('Ctrl Pts',(46.6268323415836,-25.1979861455206,11.));
#26117=CARTESIAN_POINT('Origin',(0.,0.,14.5));
#26118=CARTESIAN_POINT('',(45.9910159507966,-27.3326993144397,24.2));
#26119=CARTESIAN_POINT('Origin',(0.,0.,24.2));
#26120=CARTESIAN_POINT('',(45.9910159507966,-27.3326993144397,14.5));
#26121=CARTESIAN_POINT('Origin',(45.6125265198355,-27.5361436893127,14.5));
#26122=CARTESIAN_POINT('',(45.2340370888743,-27.7395880641857,24.2));
#26123=CARTESIAN_POINT('',(45.3706737374994,-27.666143589148,24.2));
#26124=CARTESIAN_POINT('',(45.2340370888743,-27.7395880641857,11.5));
#26125=CARTESIAN_POINT('',(45.2340370888743,-27.7395880641857,14.5));
#26126=CARTESIAN_POINT('Ctrl Pts',(45.2340370888743,-27.7395880641857,11.5));
#26127=CARTESIAN_POINT('Ctrl Pts',(45.412264930673,-27.6437876298972,11.4654707447276));
#26128=CARTESIAN_POINT('Ctrl Pts',(45.6421789133341,-27.5202050337907,11.2969997378715));
#26129=CARTESIAN_POINT('Origin',(44.74453756444,-28.9252163854584,14.5));
#26130=CARTESIAN_POINT('',(44.727601817449,-29.3545845765144,24.2));
#26131=CARTESIAN_POINT('',(44.7614733114311,-28.4958481944024,24.2));
#26132=CARTESIAN_POINT('',(44.7553594188847,-28.6508523394404,24.2));
#26133=CARTESIAN_POINT('',(44.727601817449,-29.3545845765144,11.5));
#26134=CARTESIAN_POINT('',(44.727601817449,-29.3545845765144,14.5));
#26135=CARTESIAN_POINT('',(44.7432107494939,-28.9588548268927,11.2969997378715));
#26136=CARTESIAN_POINT('Ctrl Pts',(44.727601817449,-29.3545845765144,11.5));
#26137=CARTESIAN_POINT('Ctrl Pts',(44.7354211182388,-29.156343599178,11.3977655520834));
#26138=CARTESIAN_POINT('Ctrl Pts',(44.7432107494939,-28.9588548268927,11.2969997378715));
#26139=CARTESIAN_POINT('',(44.7614733114311,-28.4958481944024,11.5));
#26140=CARTESIAN_POINT('Ctrl Pts',(44.7432107494939,-28.9588548268927,11.2969997378715));
#26141=CARTESIAN_POINT('Ctrl Pts',(44.7534983948587,-28.6980344637377,11.4654707447276));
#26142=CARTESIAN_POINT('Ctrl Pts',(44.7614733114311,-28.4958481944024,11.5));
#26143=CARTESIAN_POINT('',(44.7614733114311,-28.4958481944024,14.5));
#26144=CARTESIAN_POINT('Origin',(0.,0.,11.25));
#26145=CARTESIAN_POINT('',(43.9723514253573,-30.4742893292835,11.5));
#26146=CARTESIAN_POINT('Origin',(0.,0.,11.5));
#26147=CARTESIAN_POINT('',(43.6112843995965,-30.6370046524816,11.2969997378715));
#26148=CARTESIAN_POINT('Ctrl Pts',(43.6112843995965,-30.6370046524816,11.2969997378715));
#26149=CARTESIAN_POINT('Ctrl Pts',(43.7914747534875,-30.5558016359259,11.3977655520825));
#26150=CARTESIAN_POINT('Ctrl Pts',(43.9723514253573,-30.4742893292835,11.5));
#26151=CARTESIAN_POINT('Ctrl Pts',(43.6112843995965,-30.6370046524816,11.2969997378715));
#26152=CARTESIAN_POINT('Ctrl Pts',(43.5710559718872,-30.523318198341,11.1987310576086));
#26153=CARTESIAN_POINT('Ctrl Pts',(43.5244132133966,-30.412841346489,11.0971961933879));
#26154=CARTESIAN_POINT('Ctrl Pts',(43.4771371171594,-30.3107002244375,11.));
#26155=CARTESIAN_POINT('Ctrl Pts',(44.7432107494939,-28.9588548268927,11.2969997378715));
#26156=CARTESIAN_POINT('Ctrl Pts',(44.6227326704691,-28.9641433735292,11.1987310576086));
#26157=CARTESIAN_POINT('Ctrl Pts',(44.5028276322628,-28.9622823180478,11.0971961933879));
#26158=CARTESIAN_POINT('Ctrl Pts',(44.390414095648,-28.9567114226892,11.));
#26159=CARTESIAN_POINT('Origin',(0.,0.,14.5));
#26160=CARTESIAN_POINT('',(43.9723514253573,-30.4742893292835,24.2));
#26161=CARTESIAN_POINT('Origin',(0.,0.,24.2));
#26162=CARTESIAN_POINT('',(43.9723514253573,-30.4742893292835,14.5));
#26163=CARTESIAN_POINT('Origin',(43.5805924134329,-30.6508360358313,14.5));
#26164=CARTESIAN_POINT('',(43.1888334015085,-30.827382742379,24.2));
#26165=CARTESIAN_POINT('',(43.3302604377194,-30.7636484651835,24.2));
#26166=CARTESIAN_POINT('',(43.1888334015085,-30.827382742379,11.5));
#26167=CARTESIAN_POINT('',(43.1888334015085,-30.827382742379,14.5));
#26168=CARTESIAN_POINT('Ctrl Pts',(43.1888334015085,-30.827382742379,11.5));
#26169=CARTESIAN_POINT('Ctrl Pts',(43.3733097897213,-30.7442482189004,11.4654707447276));
#26170=CARTESIAN_POINT('Ctrl Pts',(43.6112843995965,-30.6370046524816,11.2969997378715));
#26171=CARTESIAN_POINT('Origin',(42.6178210224503,-31.9759771719266,14.5));
#26172=CARTESIAN_POINT('',(42.5709753191417,-32.4031180656588,24.2));
#26173=CARTESIAN_POINT('',(42.6646667257588,-31.5488362781943,24.2));
#26174=CARTESIAN_POINT('',(42.6477551837738,-31.7030363573407,24.2));
#26175=CARTESIAN_POINT('',(42.5709753191417,-32.4031180656588,11.5));
#26176=CARTESIAN_POINT('',(42.5709753191417,-32.4031180656588,14.5));
#26177=CARTESIAN_POINT('',(42.6141509405019,-32.0094411178763,11.2969997378715));
#26178=CARTESIAN_POINT('Ctrl Pts',(42.5709753191417,-32.4031180656588,11.5));
#26179=CARTESIAN_POINT('Ctrl Pts',(42.5926041640384,-32.2059054402292,11.3977655520831));
#26180=CARTESIAN_POINT('Ctrl Pts',(42.6141509405019,-32.0094411178763,11.2969997378715));
#26181=CARTESIAN_POINT('',(42.6646667257588,-31.5488362781943,11.5));
#26182=CARTESIAN_POINT('Ctrl Pts',(42.6141509405019,-32.0094411178763,11.2969997378715));
#26183=CARTESIAN_POINT('Ctrl Pts',(42.642607434494,-31.7499737298809,11.4654707447276));
#26184=CARTESIAN_POINT('Ctrl Pts',(42.6646667257588,-31.5488362781943,11.5));
#26185=CARTESIAN_POINT('',(42.6646667257588,-31.5488362781943,14.5));
#26186=CARTESIAN_POINT('Origin',(0.,0.,11.25));
#26187=CARTESIAN_POINT('',(41.7394580238585,-33.4674116697804,11.5));
#26188=CARTESIAN_POINT('Origin',(0.,0.,11.5));
#26189=CARTESIAN_POINT('',(41.3679200920551,-33.6045438641268,11.2969997378715));
#26190=CARTESIAN_POINT('Ctrl Pts',(41.3679200920551,-33.6045438641268,11.2969997378715));
#26191=CARTESIAN_POINT('Ctrl Pts',(41.5533359473939,-33.5361080977279,11.3977655520833));
#26192=CARTESIAN_POINT('Ctrl Pts',(41.7394580238585,-33.4674116697804,11.5));
#26193=CARTESIAN_POINT('Ctrl Pts',(41.3679200920551,-33.6045438641268,11.2969997378715));
#26194=CARTESIAN_POINT('Ctrl Pts',(41.3357200249272,-33.4883281512133,11.1987310576087));
#26195=CARTESIAN_POINT('Ctrl Pts',(41.2968973614675,-33.3748667810618,11.0971961933879));
#26196=CARTESIAN_POINT('Ctrl Pts',(41.2568614319233,-33.2696766558842,11.));
#26197=CARTESIAN_POINT('Ctrl Pts',(42.6141509405019,-32.0094411178763,11.2969997378715));
#26198=CARTESIAN_POINT('Ctrl Pts',(42.4935974296578,-32.0063126559227,11.1987310576086));
#26199=CARTESIAN_POINT('Ctrl Pts',(42.3741142947661,-31.9960919812296,11.0971961933879));
#26200=CARTESIAN_POINT('Ctrl Pts',(42.2623631978924,-31.9826930843766,11.));
#26201=CARTESIAN_POINT('Origin',(0.,0.,14.5));
#26202=CARTESIAN_POINT('',(41.7394580238585,-33.4674116697804,24.2));
#26203=CARTESIAN_POINT('Origin',(0.,0.,24.2));
#26204=CARTESIAN_POINT('',(41.7394580238585,-33.4674116697804,14.5));
#26205=CARTESIAN_POINT('Origin',(41.3363380414975,-33.6162005901948,14.5));
#26206=CARTESIAN_POINT('',(40.9332180591366,-33.7649895106092,24.2));
#26207=CARTESIAN_POINT('',(41.0787464646293,-33.7112759382477,24.2));
#26208=CARTESIAN_POINT('',(40.9332180591366,-33.7649895106092,11.5));
#26209=CARTESIAN_POINT('',(40.9332180591366,-33.7649895106092,14.5));
#26210=CARTESIAN_POINT('Ctrl Pts',(40.9332180591366,-33.7649895106092,11.5));
#26211=CARTESIAN_POINT('Ctrl Pts',(41.1230442433438,-33.6949259209822,11.4654707447276));
#26212=CARTESIAN_POINT('Ctrl Pts',(41.3679200920551,-33.6045438641268,11.2969997378715));
#26213=CARTESIAN_POINT('Origin',(40.2834747403676,-34.870954211827,14.5));
#26214=CARTESIAN_POINT('',(40.2069473082993,-35.2937868207372,24.2));
#26215=CARTESIAN_POINT('',(40.3600021724359,-34.4481216029168,24.2));
#26216=CARTESIAN_POINT('',(40.332375372345,-34.600766368886,24.2));
#26217=CARTESIAN_POINT('',(40.2069473082993,-35.2937868207372,11.5));
#26218=CARTESIAN_POINT('',(40.2069473082993,-35.2937868207372,14.5));
#26219=CARTESIAN_POINT('',(40.2774792716874,-34.9040806293114,11.2969997378715));
#26220=CARTESIAN_POINT('Ctrl Pts',(40.2069473082993,-35.2937868207372,11.5));
#26221=CARTESIAN_POINT('Ctrl Pts',(40.2422803237448,-35.0985633473018,11.3977655520828));
#26222=CARTESIAN_POINT('Ctrl Pts',(40.2774792716874,-34.9040806293114,11.2969997378715));
#26223=CARTESIAN_POINT('',(40.3600021724359,-34.4481216029168,11.5));
#26224=CARTESIAN_POINT('Ctrl Pts',(40.2774792716874,-34.9040806293114,11.2969997378715));
#26225=CARTESIAN_POINT('Ctrl Pts',(40.3239659771285,-34.6472303155083,11.4654707447276));
#26226=CARTESIAN_POINT('Ctrl Pts',(40.3600021724359,-34.4481216029168,11.5));
#26227=CARTESIAN_POINT('',(40.3600021724359,-34.4481216029168,14.5));
#26228=CARTESIAN_POINT('Origin',(0.,0.,11.25));
#26229=CARTESIAN_POINT('',(39.3032141785033,-36.2974841447544,11.5));
#26230=CARTESIAN_POINT('Origin',(0.,0.,11.5));
#26231=CARTESIAN_POINT('',(38.4781801929733,-36.5380966439885,11.0622545443402));
#26232=CARTESIAN_POINT('Ctrl Pts',(38.4781801929733,-36.5380966439885,11.0622545443402));
#26233=CARTESIAN_POINT('Ctrl Pts',(38.8890026134927,-36.4182845985743,11.277661807521));
#26234=CARTESIAN_POINT('Ctrl Pts',(39.3032141785033,-36.2974841447544,11.5));
#26235=CARTESIAN_POINT('Ctrl Pts',(38.3731925086332,-36.5581467896744,11.));
#26236=CARTESIAN_POINT('Ctrl Pts',(38.4091057617122,-36.5483957475015,11.0192759649605));
#26237=CARTESIAN_POINT('Ctrl Pts',(38.4444991653313,-36.5418944270792,11.0404458048696));
#26238=CARTESIAN_POINT('Ctrl Pts',(38.4781801929732,-36.5380966439885,11.0622545443403));
#26239=CARTESIAN_POINT('Ctrl Pts',(40.2774792716874,-34.9040806293114,11.2969997378715));
#26240=CARTESIAN_POINT('Ctrl Pts',(40.1574376536108,-34.8925504003199,11.1987310576087));
#26241=CARTESIAN_POINT('Ctrl Pts',(40.0389585318564,-34.8740199005147,11.0971961933879));
#26242=CARTESIAN_POINT('Ctrl Pts',(39.9284143148345,-34.8528582802461,11.));
#26243=CARTESIAN_POINT('Origin',(0.,0.,14.5));
#26244=CARTESIAN_POINT('',(39.3032141785033,-36.2974841447544,24.2));
#26245=CARTESIAN_POINT('Origin',(0.,0.,24.2));
#26246=CARTESIAN_POINT('',(39.3032141785033,-36.2974841447544,14.5));
#26247=CARTESIAN_POINT('Origin',(37.7528714186304,-37.5960434680237,14.5));
#26248=CARTESIAN_POINT('',(37.8587077455022,-37.1795791419031,11.0622545443405));
#26249=CARTESIAN_POINT('',(37.8587077455022,-37.1795791419031,24.2));
#26250=CARTESIAN_POINT('',(37.8587077455022,-37.1795791419031,14.5));
#26251=CARTESIAN_POINT('',(37.6470350917587,-38.0125077941444,24.2));
#26252=CARTESIAN_POINT('',(37.8205002822982,-37.3299249247391,24.2));
#26253=CARTESIAN_POINT('',(37.6470350917587,-38.0125077941444,11.5));
#26254=CARTESIAN_POINT('',(37.6470350917587,-38.0125077941444,14.5));
#26255=CARTESIAN_POINT('Ctrl Pts',(37.6470350917587,-38.0125077941444,11.5));
#26256=CARTESIAN_POINT('Ctrl Pts',(37.7174206768073,-37.7355415944255,11.3527407245747));
#26257=CARTESIAN_POINT('Ctrl Pts',(37.787981243994,-37.4578868426719,11.2067970124647));
#26258=CARTESIAN_POINT('Ctrl Pts',(37.8587077455022,-37.1795791419031,11.0622545443405));
#26259=CARTESIAN_POINT('Origin',(0.,0.,11.25));
#26260=CARTESIAN_POINT('Ctrl Pts',(37.8750816598376,-37.0739556732301,11.));
#26261=CARTESIAN_POINT('Ctrl Pts',(37.8665900041964,-37.1101869628422,11.0192757561174));
#26262=CARTESIAN_POINT('Ctrl Pts',(37.8613277376751,-37.1457864328837,11.0404460254343));
#26263=CARTESIAN_POINT('Ctrl Pts',(37.8587077455022,-37.1795791419031,11.0622545443405));
#26264=CARTESIAN_POINT('Origin',(0.,0.,11.5));
#26265=CARTESIAN_POINT('Origin',(0.,0.,11.25));
#26266=CARTESIAN_POINT('Origin',(0.,0.,11.5));
#26267=CARTESIAN_POINT('Origin',(0.,0.,11.25));
#26268=CARTESIAN_POINT('Origin',(0.,0.,11.5));
#26269=CARTESIAN_POINT('Origin',(0.,0.,11.25));
#26270=CARTESIAN_POINT('Origin',(0.,0.,11.5));
#26271=CARTESIAN_POINT('Origin',(0.,0.,11.25));
#26272=CARTESIAN_POINT('Origin',(0.,0.,11.5));
#26273=CARTESIAN_POINT('Origin',(0.,0.,14.5));
#26274=CARTESIAN_POINT('Origin',(0.,0.,24.2));
#26275=CARTESIAN_POINT('Origin',(0.,0.,14.5));
#26276=CARTESIAN_POINT('Origin',(0.,0.,24.2));
#26277=CARTESIAN_POINT('Origin',(0.,0.,14.5));
#26278=CARTESIAN_POINT('Origin',(0.,0.,24.2));
#26279=CARTESIAN_POINT('Origin',(0.,0.,14.5));
#26280=CARTESIAN_POINT('Origin',(0.,0.,24.2));
#26281=CARTESIAN_POINT('Origin',(0.,0.,14.5));
#26282=CARTESIAN_POINT('Origin',(0.,0.,24.2));
#26283=CARTESIAN_POINT('Origin',(38.8906971857384,-36.4177903943714,14.5));
#26284=CARTESIAN_POINT('',(38.4781801929734,-36.5380966439885,24.2));
#26285=CARTESIAN_POINT('',(38.6271009679847,-36.4946654635865,24.2));
#26286=CARTESIAN_POINT('',(38.4781801929734,-36.5380966439885,14.5));
#26287=CARTESIAN_POINT('Origin',(45.4553779539844,-28.4036725628998,11.25));
#26288=CARTESIAN_POINT('Origin',(45.4553779539844,-28.4036725628998,11.5));
#26289=CARTESIAN_POINT('Origin',(43.3633108984972,-31.5052895228766,11.25));
#26290=CARTESIAN_POINT('Origin',(43.3633108984972,-31.5052895228766,11.5));
#26291=CARTESIAN_POINT('Origin',(41.0599821511772,-34.4534158791985,11.25));
#26292=CARTESIAN_POINT('Origin',(41.0599821511772,-34.4534158791985,11.5));
#26293=CARTESIAN_POINT('Origin',(38.5566132981517,-37.2336886566023,11.));
#26294=CARTESIAN_POINT('Origin',(38.5566132981517,-37.2336886566023,24.2));
#26295=CARTESIAN_POINT('Origin',(41.0599821511772,-34.4534158791985,11.));
#26296=CARTESIAN_POINT('Origin',(41.0599821511772,-34.4534158791985,24.2));
#26297=CARTESIAN_POINT('Origin',(43.3633108984972,-31.5052895228766,11.));
#26298=CARTESIAN_POINT('Origin',(43.3633108984972,-31.5052895228766,24.2));
#26299=CARTESIAN_POINT('Origin',(45.4553779539844,-28.4036725628998,11.));
#26300=CARTESIAN_POINT('Origin',(45.4553779539844,-28.4036725628998,24.2));
#26301=CARTESIAN_POINT('Origin',(53.2009069058212,-2.89918767921613,14.5));
#26302=CARTESIAN_POINT('',(53.2196056697667,-2.87119372617343,11.2969997378715));
#26303=CARTESIAN_POINT('',(53.4395818891992,-2.54186693349002,11.5));
#26304=CARTESIAN_POINT('Ctrl Pts',(53.2196056697666,-2.87119372617343,11.2969997378715));
#26305=CARTESIAN_POINT('Ctrl Pts',(53.3293847135435,-2.70684332282478,11.397765552083));
#26306=CARTESIAN_POINT('Ctrl Pts',(53.4395818891992,-2.54186693349002,11.5));
#26307=CARTESIAN_POINT('',(53.4395818891992,-2.54186693349002,24.2));
#26308=CARTESIAN_POINT('',(53.4395818891992,-2.54186693349002,14.5));
#26309=CARTESIAN_POINT('',(52.9622319224431,-3.25650842494224,24.2));
#26310=CARTESIAN_POINT('',(53.048394829969,-3.127513781535,24.2));
#26311=CARTESIAN_POINT('',(52.9622319224431,-3.25650842494224,11.5));
#26312=CARTESIAN_POINT('',(52.9622319224431,-3.25650842494223,14.5));
#26313=CARTESIAN_POINT('Ctrl Pts',(52.9622319224431,-3.25650842494224,11.5));
#26314=CARTESIAN_POINT('Ctrl Pts',(53.0746221867387,-3.08824875867116,11.4654707447276));
#26315=CARTESIAN_POINT('Ctrl Pts',(53.2196056697667,-2.87119372617343,11.2969997378715));
#26316=CARTESIAN_POINT('Origin',(53.4694330939266,-3.73894699268513,11.25));
#26317=CARTESIAN_POINT('',(52.9000254978827,-4.14610174160441,11.5));
#26318=CARTESIAN_POINT('Origin',(53.4694330939266,-3.73894699268513,11.5));
#26319=CARTESIAN_POINT('',(53.1012690601164,-4.56348608673266,11.2969997378715));
#26320=CARTESIAN_POINT('Ctrl Pts',(53.1012690601164,-4.56348608673266,11.2969997378715));
#26321=CARTESIAN_POINT('Ctrl Pts',(52.9879047683306,-4.32836561796952,11.4654707447276));
#26322=CARTESIAN_POINT('Ctrl Pts',(52.9000254978827,-4.14610174160441,11.5));
#26323=CARTESIAN_POINT('Ctrl Pts',(52.7887618365133,-4.72722156957732,11.));
#26324=CARTESIAN_POINT('Ctrl Pts',(52.8906324750224,-4.67936541951144,11.0971961933879));
#26325=CARTESIAN_POINT('Ctrl Pts',(52.9973760525035,-4.6247166282963,11.1987310576087));
#26326=CARTESIAN_POINT('Ctrl Pts',(53.1012690601164,-4.56348608673266,11.2969997378715));
#26327=CARTESIAN_POINT('Ctrl Pts',(53.2196056697666,-2.87119372617344,11.2969997378715));
#26328=CARTESIAN_POINT('Ctrl Pts',(53.1252453861049,-2.79609996399364,11.1987310576087));
#26329=CARTESIAN_POINT('Ctrl Pts',(53.0271462715192,-2.72712717637234,11.0971961933879));
#26330=CARTESIAN_POINT('Ctrl Pts',(52.9329273198661,-2.66555910641112,11.));
#26331=CARTESIAN_POINT('Origin',(53.4694330939266,-3.73894699268513,11.));
#26332=CARTESIAN_POINT('',(52.9000254978827,-4.14610174160441,24.2));
#26333=CARTESIAN_POINT('Origin',(53.4694330939266,-3.73894699268513,24.2));
#26334=CARTESIAN_POINT('',(52.9000254978827,-4.14610174160441,14.5));
#26335=CARTESIAN_POINT('Origin',(53.0866482765093,-4.53316220395422,14.5));
#26336=CARTESIAN_POINT('',(53.273271055136,-4.92022266630402,24.2));
#26337=CARTESIAN_POINT('',(52.9673972893853,-4.28583257703742,24.2));
#26338=CARTESIAN_POINT('',(53.273271055136,-4.92022266630402,11.5));
#26339=CARTESIAN_POINT('',(53.273271055136,-4.92022266630402,14.5));
#26340=CARTESIAN_POINT('Ctrl Pts',(53.273271055136,-4.92022266630402,11.5));
#26341=CARTESIAN_POINT('Ctrl Pts',(53.1871065865071,-4.74151533319572,11.3977655520826));
#26342=CARTESIAN_POINT('Ctrl Pts',(53.1012690601164,-4.56348608673266,11.2969997378715));
#26343=CARTESIAN_POINT('Origin',(0.,0.,11.25));
#26344=CARTESIAN_POINT('',(53.1320940795741,-6.26343186434448,11.5));
#26345=CARTESIAN_POINT('Origin',(0.,0.,11.5));
#26346=CARTESIAN_POINT('',(52.889681035389,-6.5766116681379,11.2969997378715));
#26347=CARTESIAN_POINT('Ctrl Pts',(52.889681035389,-6.5766116681379,11.2969997378715));
#26348=CARTESIAN_POINT('Ctrl Pts',(53.0106571675296,-6.42031941309508,11.3977655520838));
#26349=CARTESIAN_POINT('Ctrl Pts',(53.1320940795741,-6.26343186434448,11.5));
#26350=CARTESIAN_POINT('Ctrl Pts',(52.889681035389,-6.5766116681379,11.2969997378715));
#26351=CARTESIAN_POINT('Ctrl Pts',(52.8007888846856,-6.49511858993886,11.1987310576086));
#26352=CARTESIAN_POINT('Ctrl Pts',(52.7077400330614,-6.41947076825076,11.0971961933879));
#26353=CARTESIAN_POINT('Ctrl Pts',(52.6180453654948,-6.35148029318637,11.));
#26354=CARTESIAN_POINT('Origin',(52.8690750612423,-6.60323306948161,14.5));
#26355=CARTESIAN_POINT('',(53.1320940795741,-6.26343186434448,24.2));
#26356=CARTESIAN_POINT('',(53.1320940795741,-6.26343186434448,14.5));
#26357=CARTESIAN_POINT('',(52.6060560429106,-6.94303427461875,24.2));
#26358=CARTESIAN_POINT('',(52.7010072733802,-6.82036427627618,24.2));
#26359=CARTESIAN_POINT('',(52.6060560429106,-6.94303427461875,11.5));
#26360=CARTESIAN_POINT('',(52.6060560429106,-6.94303427461874,14.5));
#26361=CARTESIAN_POINT('Ctrl Pts',(52.6060560429106,-6.94303427461875,11.5));
#26362=CARTESIAN_POINT('Ctrl Pts',(52.7299097311634,-6.78302442895846,11.4654707447276));
#26363=CARTESIAN_POINT('Ctrl Pts',(52.889681035389,-6.5766116681379,11.2969997378715));
#26364=CARTESIAN_POINT('Origin',(53.0783684845482,-7.45967821145953,11.25));
#26365=CARTESIAN_POINT('',(52.4819462572371,-7.82612128585083,11.5));
#26366=CARTESIAN_POINT('Origin',(53.0783684845482,-7.45967821145953,11.5));
#26367=CARTESIAN_POINT('',(52.6535843401555,-8.25652694495714,11.2969997378715));
#26368=CARTESIAN_POINT('Ctrl Pts',(52.6535843401555,-8.25652694495714,11.2969997378715));
#26369=CARTESIAN_POINT('Ctrl Pts',(52.5568973728928,-8.01407132459532,11.4654707447276));
#26370=CARTESIAN_POINT('Ctrl Pts',(52.4819462572371,-7.82612128585083,11.5));
#26371=CARTESIAN_POINT('Ctrl Pts',(52.6535843401555,-8.25652694495714,11.2969997378715));
#26372=CARTESIAN_POINT('Ctrl Pts',(52.5456731840226,-8.31036112214121,11.1987310576087));
#26373=CARTESIAN_POINT('Ctrl Pts',(52.4353775215618,-8.35743073608767,11.0971961933879));
#26374=CARTESIAN_POINT('Ctrl Pts',(52.3304167585326,-8.39806417445679,11.));
#26375=CARTESIAN_POINT('Origin',(53.0783684845482,-7.45967821145953,11.));
#26376=CARTESIAN_POINT('',(52.4819462572371,-7.82612128585083,24.2));
#26377=CARTESIAN_POINT('Origin',(53.0783684845482,-7.45967821145953,24.2));
#26378=CARTESIAN_POINT('',(52.4819462572371,-7.82612128585083,14.5));
#26379=CARTESIAN_POINT('Origin',(52.6411144591754,-8.22525703532526,14.5));
#26380=CARTESIAN_POINT('',(52.8002826611136,-8.6243927847997,24.2));
#26381=CARTESIAN_POINT('',(52.5394068040886,-7.97021136259661,24.2));
#26382=CARTESIAN_POINT('',(52.8002826611136,-8.6243927847997,11.5));
#26383=CARTESIAN_POINT('',(52.8002826611136,-8.6243927847997,14.5));
#26384=CARTESIAN_POINT('Ctrl Pts',(52.8002826611136,-8.6243927847997,11.5));
#26385=CARTESIAN_POINT('Ctrl Pts',(52.7267940781898,-8.44011024428003,11.3977655520829));
#26386=CARTESIAN_POINT('Ctrl Pts',(52.6535843401555,-8.25652694495714,11.2969997378715));
#26387=CARTESIAN_POINT('Origin',(52.2796703973459,-10.2751081719874,14.5));
#26388=CARTESIAN_POINT('',(52.302083191459,-10.2499890191339,11.2969997378715));
#26389=CARTESIAN_POINT('',(52.5657520484127,-9.95448198475414,11.5));
#26390=CARTESIAN_POINT('Ctrl Pts',(52.302083191459,-10.2499890191339,11.2969997378715));
#26391=CARTESIAN_POINT('Ctrl Pts',(52.4336670284067,-10.1025163525552,11.3977655520833));
#26392=CARTESIAN_POINT('Ctrl Pts',(52.5657520484127,-9.95448198475414,11.5));
#26393=CARTESIAN_POINT('',(52.5657520484127,-9.95448198475414,24.2));
#26394=CARTESIAN_POINT('',(52.5657520484127,-9.95448198475413,14.5));
#26395=CARTESIAN_POINT('',(51.9935887462792,-10.5957343592207,24.2));
#26396=CARTESIAN_POINT('',(52.0968657068422,-10.479986641844,24.2));
#26397=CARTESIAN_POINT('',(51.9935887462792,-10.5957343592207,11.5));
#26398=CARTESIAN_POINT('',(51.9935887462792,-10.5957343592207,14.5));
#26399=CARTESIAN_POINT('Ctrl Pts',(51.9935887462792,-10.5957343592207,11.5));
#26400=CARTESIAN_POINT('Ctrl Pts',(52.1283024557699,-10.4447538860551,11.4654707447276));
#26401=CARTESIAN_POINT('Ctrl Pts',(52.302083191459,-10.2499890191339,11.2969997378715));
#26402=CARTESIAN_POINT('Origin',(52.428711399332,-11.1440666278319,11.25));
#26403=CARTESIAN_POINT('',(51.8081802498931,-11.4680127538716,11.5));
#26404=CARTESIAN_POINT('Origin',(52.428711399332,-11.1440666278319,11.5));
#26405=CARTESIAN_POINT('',(51.9493766500092,-11.909342833849,11.2969997378715));
#26406=CARTESIAN_POINT('Ctrl Pts',(51.9493766500092,-11.909342833849,11.2969997378715));
#26407=CARTESIAN_POINT('Ctrl Pts',(51.8698380564552,-11.6607332812994,11.4654707447276));
#26408=CARTESIAN_POINT('Ctrl Pts',(51.8081802498931,-11.4680127538716,11.5));
#26409=CARTESIAN_POINT('Ctrl Pts',(51.9493766500092,-11.909342833849,11.2969997378715));
#26410=CARTESIAN_POINT('Ctrl Pts',(51.8379730776617,-11.9555183719537,11.1987310576086));
#26411=CARTESIAN_POINT('Ctrl Pts',(51.7246626796018,-11.9947794902037,11.0971961933879));
#26412=CARTESIAN_POINT('Ctrl Pts',(51.6171231503394,-12.0279922548488,11.));
#26413=CARTESIAN_POINT('Ctrl Pts',(52.3020831914591,-10.2499890191339,11.2969997378715));
#26414=CARTESIAN_POINT('Ctrl Pts',(52.2190922473368,-10.162493651001,11.1987310576086));
#26415=CARTESIAN_POINT('Ctrl Pts',(52.1315469833259,-10.0805393438292,11.0971961933879));
#26416=CARTESIAN_POINT('Ctrl Pts',(52.0468135832502,-10.0064577064218,11.));
#26417=CARTESIAN_POINT('Origin',(52.428711399332,-11.1440666278319,11.));
#26418=CARTESIAN_POINT('',(51.8081802498931,-11.4680127538716,24.2));
#26419=CARTESIAN_POINT('Origin',(52.428711399332,-11.1440666278319,24.2));
#26420=CARTESIAN_POINT('',(51.8081802498931,-11.4680127538716,14.5));
#26421=CARTESIAN_POINT('Origin',(51.9391184236626,-11.8772792412203,14.5));
#26422=CARTESIAN_POINT('',(52.0700565974321,-12.2865457285691,24.2));
#26423=CARTESIAN_POINT('',(51.8554496100851,-11.6157600795601,24.2));
#26424=CARTESIAN_POINT('',(52.0700565974321,-12.2865457285691,11.5));
#26425=CARTESIAN_POINT('',(52.0700565974321,-12.2865457285691,14.5));
#26426=CARTESIAN_POINT('Ctrl Pts',(52.0700565974321,-12.2865457285691,11.5));
#26427=CARTESIAN_POINT('Ctrl Pts',(52.0096019292023,-12.0975857866519,11.3977655520834));
#26428=CARTESIAN_POINT('Ctrl Pts',(51.9493766500092,-11.909342833849,11.2969997378715));
#26429=CARTESIAN_POINT('Origin',(51.4355644344077,-13.8969239803298,14.5));
#26430=CARTESIAN_POINT('',(51.4596748556075,-13.8734294539541,11.2969997378716));
#26431=CARTESIAN_POINT('',(51.7433149571623,-13.5970348695555,11.5));
#26432=CARTESIAN_POINT('Ctrl Pts',(51.4596748556075,-13.8734294539541,11.2969997378716));
#26433=CARTESIAN_POINT('Ctrl Pts',(51.6012253341357,-13.7354948478467,11.3977655520833));
#26434=CARTESIAN_POINT('Ctrl Pts',(51.7433149571623,-13.5970348695555,11.5));
#26435=CARTESIAN_POINT('',(51.7433149571623,-13.5970348695555,24.2));
#26436=CARTESIAN_POINT('',(51.7433149571622,-13.5970348695555,14.5));
#26437=CARTESIAN_POINT('',(51.1278139116531,-14.1968130911041,24.2));
#26438=CARTESIAN_POINT('',(51.238913447339,-14.0885515659373,24.2));
#26439=CARTESIAN_POINT('',(51.1278139116531,-14.1968130911041,11.5));
#26440=CARTESIAN_POINT('',(51.1278139116531,-14.1968130911041,14.5));
#26441=CARTESIAN_POINT('Ctrl Pts',(51.1278139116531,-14.1968130911041,11.5));
#26442=CARTESIAN_POINT('Ctrl Pts',(51.2727313307305,-14.055597552122,11.4654707447276));
#26443=CARTESIAN_POINT('Ctrl Pts',(51.4596748556075,-13.8734294539541,11.2969997378716));
#26444=CARTESIAN_POINT('Origin',(51.5236269022939,-14.7741622717911,11.25));
#26445=CARTESIAN_POINT('',(50.8820099961117,-15.054033216516,11.5));
#26446=CARTESIAN_POINT('Origin',(51.5236269022939,-14.7741622717911,11.5));
#26447=CARTESIAN_POINT('',(50.9920768187571,-15.5041376015772,11.2969997378715));
#26448=CARTESIAN_POINT('Ctrl Pts',(50.9920768187571,-15.5041376015772,11.2969997378715));
#26449=CARTESIAN_POINT('Ctrl Pts',(50.9300741029444,-15.2505853175897,11.4654707447276));
#26450=CARTESIAN_POINT('Ctrl Pts',(50.8820099961117,-15.054033216516,11.5));
#26451=CARTESIAN_POINT('Ctrl Pts',(50.9920768187571,-15.5041376015772,11.2969997378715));
#26452=CARTESIAN_POINT('Ctrl Pts',(50.8777235772014,-15.5424295380224,11.1987310576086));
#26453=CARTESIAN_POINT('Ctrl Pts',(50.7619504804118,-15.5736908843544,11.0971961933879));
#26454=CARTESIAN_POINT('Ctrl Pts',(50.6523561066928,-15.5993211660246,11.));
#26455=CARTESIAN_POINT('Ctrl Pts',(51.4596748556075,-13.8734294539541,11.2969997378716));
#26456=CARTESIAN_POINT('Ctrl Pts',(51.3829894416039,-13.7803580645257,11.1987310576087));
#26457=CARTESIAN_POINT('Ctrl Pts',(51.3013742769325,-13.6924965450168,11.097196193388));
#26458=CARTESIAN_POINT('Ctrl Pts',(51.2220149569554,-13.6126846635571,11.));
#26459=CARTESIAN_POINT('Origin',(51.5236269022939,-14.7741622717911,11.));
#26460=CARTESIAN_POINT('',(50.8820099961117,-15.054033216516,24.2));
#26461=CARTESIAN_POINT('Origin',(51.5236269022939,-14.7741622717911,24.2));
#26462=CARTESIAN_POINT('',(50.8820099961117,-15.054033216516,14.5));
#26463=CARTESIAN_POINT('Origin',(50.9840802240917,-15.4714365365519,14.5));
#26464=CARTESIAN_POINT('',(51.0861504520717,-15.8888398565878,24.2));
#26465=CARTESIAN_POINT('',(50.9188578780728,-15.204717981028,24.2));
#26466=CARTESIAN_POINT('',(51.0861504520717,-15.8888398565878,11.5));
#26467=CARTESIAN_POINT('',(51.0861504520717,-15.8888398565878,14.5));
#26468=CARTESIAN_POINT('Ctrl Pts',(51.0861504520717,-15.8888398565878,11.5));
#26469=CARTESIAN_POINT('Ctrl Pts',(51.039024227602,-15.6961231071132,11.3977655520826));
#26470=CARTESIAN_POINT('Ctrl Pts',(50.9920768187571,-15.5041376015772,11.2969997378715));
#26471=CARTESIAN_POINT('Origin',(50.34086957183,-17.4510353719535,14.5));
#26472=CARTESIAN_POINT('',(50.3665601565676,-17.4292799350267,11.2969997378715));
#26473=CARTESIAN_POINT('',(50.6687896366606,-17.1733443672407,11.5));
#26474=CARTESIAN_POINT('Ctrl Pts',(50.3665601565676,-17.4292799350267,11.2969997378715));
#26475=CARTESIAN_POINT('Ctrl Pts',(50.5173876569724,-17.3015553929273,11.3977655520822));
#26476=CARTESIAN_POINT('Ctrl Pts',(50.6687896366606,-17.1733443672407,11.5));
#26477=CARTESIAN_POINT('',(50.6687896366606,-17.1733443672407,24.2));
#26478=CARTESIAN_POINT('',(50.6687896366606,-17.1733443672407,14.5));
#26479=CARTESIAN_POINT('',(50.0129495069995,-17.7287263766662,24.2));
#26480=CARTESIAN_POINT('',(50.131330352038,-17.6284784829776,24.2));
#26481=CARTESIAN_POINT('',(50.0129495069995,-17.7287263766662,11.5));
#26482=CARTESIAN_POINT('',(50.0129495069995,-17.7287263766662,14.5));
#26483=CARTESIAN_POINT('Ctrl Pts',(50.0129495069995,-17.7287263766662,11.5));
#26484=CARTESIAN_POINT('Ctrl Pts',(50.1673646125647,-17.5979637597785,11.4654707447276));
#26485=CARTESIAN_POINT('Ctrl Pts',(50.3665601565676,-17.4292799350267,11.2969997378715));
#26486=CARTESIAN_POINT('Origin',(50.3675244741247,-18.3322796822558,11.25));
#26487=CARTESIAN_POINT('',(49.7079477042709,-18.5667119425557,11.5));
#26488=CARTESIAN_POINT('Origin',(50.3675244741247,-18.3322796822558,11.5));
#26489=CARTESIAN_POINT('',(49.7863487149498,-19.023397769381,11.2969997378715));
#26490=CARTESIAN_POINT('Ctrl Pts',(49.7863487149498,-19.023397769381,11.2969997378715));
#26491=CARTESIAN_POINT('Ctrl Pts',(49.7421839478773,-18.7661380351961,11.4654707447276));
#26492=CARTESIAN_POINT('Ctrl Pts',(49.7079477042709,-18.5667119425557,11.5));
#26493=CARTESIAN_POINT('Ctrl Pts',(49.7863487149498,-19.023397769381,11.2969997378715));
#26494=CARTESIAN_POINT('Ctrl Pts',(49.6696029216838,-19.0536195497014,11.1987310576087));
#26495=CARTESIAN_POINT('Ctrl Pts',(49.5519311610547,-19.0767288219785,11.0971961933879));
#26496=CARTESIAN_POINT('Ctrl Pts',(49.4408158756514,-19.0946517525179,11.));
#26497=CARTESIAN_POINT('Ctrl Pts',(50.3665601565676,-17.4292799350267,11.2969997378715));
#26498=CARTESIAN_POINT('Ctrl Pts',(50.2965538763113,-17.3310859587567,11.1987310576086));
#26499=CARTESIAN_POINT('Ctrl Pts',(50.2212664318579,-17.2377452794019,11.0971961933879));
#26500=CARTESIAN_POINT('Ctrl Pts',(50.1476678226092,-17.1525919893539,11.));
#26501=CARTESIAN_POINT('Origin',(50.3675244741247,-18.3322796822558,11.));
#26502=CARTESIAN_POINT('',(49.7079477042709,-18.5667119425557,24.2));
#26503=CARTESIAN_POINT('Origin',(50.3675244741247,-18.3322796822558,24.2));
#26504=CARTESIAN_POINT('',(49.7079477042709,-18.5667119425557,14.5));
#26505=CARTESIAN_POINT('Origin',(49.7806527105709,-18.9902185482606,14.5));
#26506=CARTESIAN_POINT('',(49.8533577168708,-19.4137251539655,24.2));
#26507=CARTESIAN_POINT('',(49.7341945888243,-18.7196000248653,24.2));
#26508=CARTESIAN_POINT('',(49.8533577168708,-19.4137251539655,11.5));
#26509=CARTESIAN_POINT('',(49.8533577168709,-19.4137251539655,14.5));
#26510=CARTESIAN_POINT('Ctrl Pts',(49.8533577168708,-19.4137251539655,11.5));
#26511=CARTESIAN_POINT('Ctrl Pts',(49.8197895303902,-19.2181904935674,11.3977655520828));
#26512=CARTESIAN_POINT('Ctrl Pts',(49.7863487149498,-19.023397769381,11.2969997378715));
#26513=CARTESIAN_POINT('Origin',(49.0009190529448,-20.9201270734171,14.5));
#26514=CARTESIAN_POINT('',(49.028064639274,-20.900216716241,11.2969997378715));
#26515=CARTESIAN_POINT('',(49.3474110662579,-20.6659870574277,11.5));
#26516=CARTESIAN_POINT('Ctrl Pts',(49.028064639274,-20.900216716241,11.2969997378715));
#26517=CARTESIAN_POINT('Ctrl Pts',(49.1874343451367,-20.7833244992779,11.3977655520828));
#26518=CARTESIAN_POINT('Ctrl Pts',(49.3474110662579,-20.6659870574277,11.5));
#26519=CARTESIAN_POINT('',(49.3474110662579,-20.6659870574277,24.2));
#26520=CARTESIAN_POINT('',(49.3474110662579,-20.6659870574277,14.5));
#26521=CARTESIAN_POINT('',(48.6544270396318,-21.1742670894066,24.2));
#26522=CARTESIAN_POINT('',(48.7795124544456,-21.0825212248573,24.2));
#26523=CARTESIAN_POINT('',(48.6544270396318,-21.1742670894066,11.5));
#26524=CARTESIAN_POINT('',(48.6544270396318,-21.1742670894066,14.5));
#26525=CARTESIAN_POINT('Ctrl Pts',(48.6544270396318,-21.1742670894066,11.5));
#26526=CARTESIAN_POINT('Ctrl Pts',(48.8175875368124,-21.0545944569386,11.4654707447276));
#26527=CARTESIAN_POINT('Ctrl Pts',(49.028064639274,-20.900216716241,11.2969997378715));
#26528=CARTESIAN_POINT('Origin',(48.9660365296434,-21.8010840688629,11.25));
#26529=CARTESIAN_POINT('',(48.2917132878404,-21.9889355143306,11.5));
#26530=CARTESIAN_POINT('Origin',(48.9660365296434,-21.8010840688629,11.5));
#26531=CARTESIAN_POINT('',(48.3380665247095,-22.4499778554777,11.2969997378716));
#26532=CARTESIAN_POINT('Ctrl Pts',(48.3380665247095,-22.4499778554777,11.2969997378716));
#26533=CARTESIAN_POINT('Ctrl Pts',(48.3119548726829,-22.1902640146607,11.4654707447277));
#26534=CARTESIAN_POINT('Ctrl Pts',(48.2917132878404,-21.9889355143306,11.5));
#26535=CARTESIAN_POINT('Ctrl Pts',(48.3380665247095,-22.4499778554777,11.2969997378716));
#26536=CARTESIAN_POINT('Ctrl Pts',(48.2194969535028,-22.4719822421975,11.1987310576087));
#26537=CARTESIAN_POINT('Ctrl Pts',(48.1004998140236,-22.486826854368,11.0971961933879));
#26538=CARTESIAN_POINT('Ctrl Pts',(47.9884049594373,-22.4969551150606,11.));
#26539=CARTESIAN_POINT('Ctrl Pts',(49.028064639274,-20.900216716241,11.2969997378714));
#26540=CARTESIAN_POINT('Ctrl Pts',(48.9650785563254,-20.7973785443114,11.1987310576086));
#26541=CARTESIAN_POINT('Ctrl Pts',(48.8964856249515,-20.699013451518,11.0971961933879));
#26542=CARTESIAN_POINT('Ctrl Pts',(48.8290062914572,-20.608933611151,11.));
#26543=CARTESIAN_POINT('Origin',(48.9660365296434,-21.8010840688629,11.));
#26544=CARTESIAN_POINT('',(48.2917132878404,-21.9889355143306,24.2));
#26545=CARTESIAN_POINT('Origin',(48.9660365296434,-21.8010840688629,24.2));
#26546=CARTESIAN_POINT('',(48.2917132878404,-21.9889355143306,14.5));
#26547=CARTESIAN_POINT('Origin',(47.4222409819888,-24.287298018663,14.5));
#26548=CARTESIAN_POINT('',(47.0588650944528,-24.5166489013173,11.0622545443403));
#26549=CARTESIAN_POINT('',(47.7856168695248,-24.0579471360087,11.5));
#26550=CARTESIAN_POINT('Ctrl Pts',(47.0588650944528,-24.5166489013173,11.0622545443403));
#26551=CARTESIAN_POINT('Ctrl Pts',(47.4207482757382,-24.2882401656459,11.2776618075213));
#26552=CARTESIAN_POINT('Ctrl Pts',(47.7856168695248,-24.0579471360087,11.5));
#26553=CARTESIAN_POINT('',(47.7856168695248,-24.0579471360087,24.2));
#26554=CARTESIAN_POINT('',(47.7856168695248,-24.0579471360087,14.5));
#26555=CARTESIAN_POINT('',(47.0588650944529,-24.5166489013173,24.2));
#26556=CARTESIAN_POINT('',(47.1900456754746,-24.4338520425371,24.2));
#26557=CARTESIAN_POINT('',(47.0588650944529,-24.5166489013173,14.5));
#26558=CARTESIAN_POINT('Origin',(0.,0.,14.5));
#26559=CARTESIAN_POINT('',(48.3776844341154,-22.8440287338541,11.5));
#26560=CARTESIAN_POINT('Origin',(0.,0.,11.5));
#26561=CARTESIAN_POINT('',(48.3776844341154,-22.8440287338541,24.2));
#26562=CARTESIAN_POINT('',(48.3776844341154,-22.8440287338541,14.5));
#26563=CARTESIAN_POINT('Origin',(0.,0.,24.2));
#26564=CARTESIAN_POINT('Origin',(0.,0.,11.25));
#26565=CARTESIAN_POINT('Ctrl Pts',(46.9634710240919,-24.5648608660681,11.));
#26566=CARTESIAN_POINT('Ctrl Pts',(46.9953053071723,-24.5455885286143,11.0192759649605));
#26567=CARTESIAN_POINT('Ctrl Pts',(47.0275356235898,-24.5295833141324,11.0404458048696));
#26568=CARTESIAN_POINT('Ctrl Pts',(47.0588650944527,-24.5166489013174,11.0622545443404));
#26569=CARTESIAN_POINT('Ctrl Pts',(48.3776844341154,-22.8440287338541,11.5));
#26570=CARTESIAN_POINT('Ctrl Pts',(48.3578378264539,-22.6466287877422,11.3977655520828));
#26571=CARTESIAN_POINT('Ctrl Pts',(48.3380665247095,-22.4499778554777,11.2969997378716));
#26572=CARTESIAN_POINT('Origin',(48.3346988609779,-22.4164821240923,14.5));
#26573=CARTESIAN_POINT('',(48.3072313028028,-22.1432820590691,24.2));
#26574=CARTESIAN_POINT('Origin',(52.2796703973459,10.2751081719876,14.5));
#26575=CARTESIAN_POINT('',(52.5657520484127,9.95448198475442,24.2));
#26576=CARTESIAN_POINT('',(51.9935887462791,10.5957343592208,24.2));
#26577=CARTESIAN_POINT('',(52.0968657068422,10.479986641844,24.2));
#26578=CARTESIAN_POINT('',(52.5657520484127,9.95448198475442,11.5));
#26579=CARTESIAN_POINT('',(52.5657520484127,9.95448198475442,14.5));
#26580=CARTESIAN_POINT('',(51.993588746279,10.5957343592209,11.0622545443402));
#26581=CARTESIAN_POINT('Ctrl Pts',(52.5657520484127,9.95448198475442,11.5));
#26582=CARTESIAN_POINT('Ctrl Pts',(52.278495206905,10.2764252674005,11.2776618075198));
#26583=CARTESIAN_POINT('Ctrl Pts',(51.993588746279,10.5957343592209,11.0622545443402));
#26584=CARTESIAN_POINT('',(51.9935887462791,10.5957343592208,14.5));
#26585=CARTESIAN_POINT('Origin',(0.,0.,11.25));
#26586=CARTESIAN_POINT('',(52.8002826611136,8.62439278479999,11.5));
#26587=CARTESIAN_POINT('Origin',(0.,0.,11.5));
#26588=CARTESIAN_POINT('',(52.6535843401555,8.25652694495716,11.2969997378715));
#26589=CARTESIAN_POINT('Ctrl Pts',(52.6535843401555,8.25652694495716,11.2969997378715));
#26590=CARTESIAN_POINT('Ctrl Pts',(52.7267940781897,8.4401102442802,11.3977655520829));
#26591=CARTESIAN_POINT('Ctrl Pts',(52.8002826611136,8.62439278479999,11.5));
#26592=CARTESIAN_POINT('Ctrl Pts',(52.6535843401555,8.25652694495715,11.2969997378715));
#26593=CARTESIAN_POINT('Ctrl Pts',(52.5456731840225,8.31036112214122,11.1987310576086));
#26594=CARTESIAN_POINT('Ctrl Pts',(52.4353775215617,8.35743073608767,11.0971961933879));
#26595=CARTESIAN_POINT('Ctrl Pts',(52.3304167585326,8.39806417445676,11.));
#26596=CARTESIAN_POINT('Ctrl Pts',(51.993588746279,10.5957343592209,11.0622545443403));
#26597=CARTESIAN_POINT('Ctrl Pts',(51.9670381333318,10.6168032873272,11.0404458048695));
#26598=CARTESIAN_POINT('Ctrl Pts',(51.9404679997109,10.6410723661384,11.0192759649605));
#26599=CARTESIAN_POINT('Ctrl Pts',(51.9151790989041,10.6683728435365,11.));
#26600=CARTESIAN_POINT('Origin',(0.,0.,14.5));
#26601=CARTESIAN_POINT('',(52.8002826611136,8.62439278479999,24.2));
#26602=CARTESIAN_POINT('Origin',(0.,0.,24.2));
#26603=CARTESIAN_POINT('',(52.8002826611136,8.62439278479999,14.5));
#26604=CARTESIAN_POINT('Origin',(52.6411144591754,8.22525703532543,14.5));
#26605=CARTESIAN_POINT('',(52.4819462572372,7.82612128585089,24.2));
#26606=CARTESIAN_POINT('',(52.5394068040886,7.97021136259661,24.2));
#26607=CARTESIAN_POINT('',(52.4819462572372,7.82612128585089,11.5));
#26608=CARTESIAN_POINT('',(52.4819462572372,7.82612128585088,14.5));
#26609=CARTESIAN_POINT('Ctrl Pts',(52.4819462572372,7.82612128585089,11.5));
#26610=CARTESIAN_POINT('Ctrl Pts',(52.5568973728928,8.01407132459532,11.4654707447276));
#26611=CARTESIAN_POINT('Ctrl Pts',(52.6535843401555,8.25652694495716,11.2969997378715));
#26612=CARTESIAN_POINT('Origin',(52.8690750612423,6.60323306948177,14.5));
#26613=CARTESIAN_POINT('',(53.1320940795741,6.26343186434477,24.2));
#26614=CARTESIAN_POINT('',(52.6060560429105,6.94303427461878,24.2));
#26615=CARTESIAN_POINT('',(52.7010072733802,6.82036427627619,24.2));
#26616=CARTESIAN_POINT('',(53.1320940795741,6.26343186434477,11.5));
#26617=CARTESIAN_POINT('',(53.1320940795741,6.26343186434477,14.5));
#26618=CARTESIAN_POINT('',(52.889681035389,6.57661166813793,11.2969997378715));
#26619=CARTESIAN_POINT('Ctrl Pts',(53.1320940795741,6.26343186434477,11.5));
#26620=CARTESIAN_POINT('Ctrl Pts',(53.0106571675283,6.42031941309698,11.3977655520827));
#26621=CARTESIAN_POINT('Ctrl Pts',(52.889681035389,6.57661166813793,11.2969997378715));
#26622=CARTESIAN_POINT('',(52.6060560429105,6.94303427461878,11.5));
#26623=CARTESIAN_POINT('Ctrl Pts',(52.889681035389,6.57661166813793,11.2969997378715));
#26624=CARTESIAN_POINT('Ctrl Pts',(52.7299097311634,6.78302442895845,11.4654707447276));
#26625=CARTESIAN_POINT('Ctrl Pts',(52.6060560429105,6.94303427461878,11.5));
#26626=CARTESIAN_POINT('',(52.6060560429105,6.94303427461878,14.5));
#26627=CARTESIAN_POINT('Origin',(0.,0.,11.25));
#26628=CARTESIAN_POINT('',(53.273271055136,4.920222666304,11.5));
#26629=CARTESIAN_POINT('Origin',(0.,0.,11.5));
#26630=CARTESIAN_POINT('',(53.1012690601164,4.56348608673264,11.2969997378715));
#26631=CARTESIAN_POINT('Ctrl Pts',(53.1012690601164,4.56348608673264,11.2969997378715));
#26632=CARTESIAN_POINT('Ctrl Pts',(53.1871065865071,4.74151533319583,11.3977655520826));
#26633=CARTESIAN_POINT('Ctrl Pts',(53.273271055136,4.920222666304,11.5));
#26634=CARTESIAN_POINT('Ctrl Pts',(53.1012690601164,4.56348608673263,11.2969997378715));
#26635=CARTESIAN_POINT('Ctrl Pts',(52.9973760525035,4.62471662829628,11.1987310576087));
#26636=CARTESIAN_POINT('Ctrl Pts',(52.8906324750223,4.67936541951142,11.0971961933879));
#26637=CARTESIAN_POINT('Ctrl Pts',(52.7887618365133,4.72722156957729,11.));
#26638=CARTESIAN_POINT('Ctrl Pts',(52.889681035389,6.57661166813793,11.2969997378715));
#26639=CARTESIAN_POINT('Ctrl Pts',(52.8007888846856,6.49511858993887,11.1987310576087));
#26640=CARTESIAN_POINT('Ctrl Pts',(52.7077400330614,6.41947076825075,11.0971961933879));
#26641=CARTESIAN_POINT('Ctrl Pts',(52.6180453654948,6.35148029318636,11.));
#26642=CARTESIAN_POINT('Origin',(0.,0.,14.5));
#26643=CARTESIAN_POINT('',(53.273271055136,4.920222666304,24.2));
#26644=CARTESIAN_POINT('Origin',(0.,0.,24.2));
#26645=CARTESIAN_POINT('',(53.273271055136,4.920222666304,14.5));
#26646=CARTESIAN_POINT('Origin',(53.0866482765093,4.5331622039542,14.5));
#26647=CARTESIAN_POINT('',(52.9000254978827,4.1461017416044,24.2));
#26648=CARTESIAN_POINT('',(52.9673972893853,4.2858325770374,24.2));
#26649=CARTESIAN_POINT('',(52.9000254978827,4.1461017416044,11.5));
#26650=CARTESIAN_POINT('',(52.9000254978827,4.1461017416044,14.5));
#26651=CARTESIAN_POINT('Ctrl Pts',(52.9000254978827,4.1461017416044,11.5));
#26652=CARTESIAN_POINT('Ctrl Pts',(52.9879047683306,4.32836561796949,11.4654707447276));
#26653=CARTESIAN_POINT('Ctrl Pts',(53.1012690601164,4.56348608673264,11.2969997378715));
#26654=CARTESIAN_POINT('Origin',(53.2009069058212,2.89918767921592,14.5));
#26655=CARTESIAN_POINT('',(53.4395818891992,2.54186693348969,24.2));
#26656=CARTESIAN_POINT('',(52.9622319224432,3.25650842494215,24.2));
#26657=CARTESIAN_POINT('',(53.048394829969,3.12751378153496,24.2));
#26658=CARTESIAN_POINT('',(53.4395818891992,2.54186693348969,11.5));
#26659=CARTESIAN_POINT('',(53.4395818891992,2.54186693348969,14.5));
#26660=CARTESIAN_POINT('',(53.2196056697666,2.87119372617337,11.2969997378715));
#26661=CARTESIAN_POINT('Ctrl Pts',(53.4395818891992,2.54186693348969,11.5));
#26662=CARTESIAN_POINT('Ctrl Pts',(53.3293847135434,2.70684332282464,11.3977655520829));
#26663=CARTESIAN_POINT('Ctrl Pts',(53.2196056697666,2.87119372617337,11.2969997378715));
#26664=CARTESIAN_POINT('',(52.9622319224432,3.25650842494215,11.5));
#26665=CARTESIAN_POINT('Ctrl Pts',(53.2196056697666,2.87119372617337,11.2969997378715));
#26666=CARTESIAN_POINT('Ctrl Pts',(53.0746221867387,3.08824875867107,11.4654707447276));
#26667=CARTESIAN_POINT('Ctrl Pts',(52.9622319224432,3.25650842494215,11.5));
#26668=CARTESIAN_POINT('',(52.9622319224432,3.25650842494215,14.5));
#26669=CARTESIAN_POINT('Origin',(0.,0.,11.25));
#26670=CARTESIAN_POINT('',(53.4867174275882,1.19208171755715,11.5));
#26671=CARTESIAN_POINT('Origin',(0.,0.,11.5));
#26672=CARTESIAN_POINT('',(53.0603811317944,0.445882806437465,11.0622545443402));
#26673=CARTESIAN_POINT('Ctrl Pts',(53.0603811317944,0.445882806437465,11.0622545443402));
#26674=CARTESIAN_POINT('Ctrl Pts',(53.2726736095176,0.817449612451526,11.277661807522));
#26675=CARTESIAN_POINT('Ctrl Pts',(53.4867174275882,1.19208171755715,11.5));
#26676=CARTESIAN_POINT('Ctrl Pts',(52.9987873134328,0.358529364921033,11.));
#26677=CARTESIAN_POINT('Ctrl Pts',(53.0178475026662,0.390491119512532,11.0192759649605));
#26678=CARTESIAN_POINT('Ctrl Pts',(53.0387911899085,0.419754102130115,11.0404458048696));
#26679=CARTESIAN_POINT('Ctrl Pts',(53.0603811317944,0.445882806437441,11.0622545443403));
#26680=CARTESIAN_POINT('Ctrl Pts',(52.9329273198661,2.66555910641111,11.));
#26681=CARTESIAN_POINT('Ctrl Pts',(53.0271462715192,2.7271271763723,11.0971961933878));
#26682=CARTESIAN_POINT('Ctrl Pts',(53.1252453861049,2.79609996399359,11.1987310576086));
#26683=CARTESIAN_POINT('Ctrl Pts',(53.2196056697666,2.87119372617338,11.2969997378715));
#26684=CARTESIAN_POINT('Origin',(0.,0.,14.5));
#26685=CARTESIAN_POINT('',(53.4867174275882,1.19208171755715,24.2));
#26686=CARTESIAN_POINT('Origin',(0.,0.,24.2));
#26687=CARTESIAN_POINT('',(53.4867174275882,1.19208171755715,14.5));
#26688=CARTESIAN_POINT('Origin',(53.2735492796914,-0.818982261997365,14.5));
#26689=CARTESIAN_POINT('',(53.0603811317945,-0.44588280643758,11.0622545443404));
#26690=CARTESIAN_POINT('',(53.0603811317945,-0.44588280643758,24.2));
#26691=CARTESIAN_POINT('',(53.0603811317945,-0.44588280643758,14.5));
#26692=CARTESIAN_POINT('',(53.4867174275882,-1.19208171755715,24.2));
#26693=CARTESIAN_POINT('',(53.1373359393522,-0.580573645973269,24.2));
#26694=CARTESIAN_POINT('',(53.4867174275882,-1.19208171755715,11.5));
#26695=CARTESIAN_POINT('',(53.4867174275882,-1.19208171755715,14.5));
#26696=CARTESIAN_POINT('Ctrl Pts',(53.4867174275882,-1.19208171755715,11.5));
#26697=CARTESIAN_POINT('Ctrl Pts',(53.3449516913153,-0.943954970938041,
11.3527407245752));
#26698=CARTESIAN_POINT('Ctrl Pts',(53.2028335182235,-0.695211368627667,
11.2067970124649));
#26699=CARTESIAN_POINT('Ctrl Pts',(53.0603811317945,-0.44588280643758,11.0622545443404));
#26700=CARTESIAN_POINT('Origin',(0.,0.,11.25));
#26701=CARTESIAN_POINT('Ctrl Pts',(52.9987873134328,-0.358529364921033,
11.));
#26702=CARTESIAN_POINT('Ctrl Pts',(53.0178472961609,-0.390490773226817,
11.0192757561174));
#26703=CARTESIAN_POINT('Ctrl Pts',(53.0387914082603,-0.419754366385171,
11.0404460254342));
#26704=CARTESIAN_POINT('Ctrl Pts',(53.0603811317945,-0.44588280643758,11.0622545443404));
#26705=CARTESIAN_POINT('Origin',(0.,0.,11.5));
#26706=CARTESIAN_POINT('Origin',(0.,0.,11.25));
#26707=CARTESIAN_POINT('Origin',(0.,0.,11.5));
#26708=CARTESIAN_POINT('Origin',(0.,0.,11.25));
#26709=CARTESIAN_POINT('Origin',(0.,0.,11.5));
#26710=CARTESIAN_POINT('Origin',(0.,0.,11.25));
#26711=CARTESIAN_POINT('Origin',(0.,0.,11.5));
#26712=CARTESIAN_POINT('Origin',(0.,0.,11.25));
#26713=CARTESIAN_POINT('Origin',(0.,0.,11.5));
#26714=CARTESIAN_POINT('Origin',(0.,0.,14.5));
#26715=CARTESIAN_POINT('Origin',(0.,0.,24.2));
#26716=CARTESIAN_POINT('Origin',(0.,0.,14.5));
#26717=CARTESIAN_POINT('Origin',(0.,0.,24.2));
#26718=CARTESIAN_POINT('Origin',(0.,0.,14.5));
#26719=CARTESIAN_POINT('Origin',(0.,0.,24.2));
#26720=CARTESIAN_POINT('Origin',(0.,0.,14.5));
#26721=CARTESIAN_POINT('Origin',(0.,0.,24.2));
#26722=CARTESIAN_POINT('Origin',(0.,0.,14.5));
#26723=CARTESIAN_POINT('Origin',(0.,0.,24.2));
#26724=CARTESIAN_POINT('Origin',(0.,0.,14.5));
#26725=CARTESIAN_POINT('Origin',(0.,0.,24.2));
#26726=CARTESIAN_POINT('Origin',(53.2735492796914,0.818982261997365,14.5));
#26727=CARTESIAN_POINT('',(53.0603811317945,0.44588280643758,24.2));
#26728=CARTESIAN_POINT('',(53.1373359393522,0.580573645973269,24.2));
#26729=CARTESIAN_POINT('',(53.0603811317945,0.44588280643758,14.5));
#26730=CARTESIAN_POINT('Origin',(53.0783684845482,7.45967821145951,11.25));
#26731=CARTESIAN_POINT('Origin',(53.0783684845482,7.45967821145951,11.5));
#26732=CARTESIAN_POINT('Origin',(53.4694330939266,3.73894699268512,11.25));
#26733=CARTESIAN_POINT('Origin',(53.4694330939266,3.73894699268512,11.5));
#26734=CARTESIAN_POINT('Origin',(53.6,0.,11.));
#26735=CARTESIAN_POINT('Origin',(53.6,0.,24.2));
#26736=CARTESIAN_POINT('Origin',(53.4694330939266,3.73894699268512,11.));
#26737=CARTESIAN_POINT('Origin',(53.4694330939266,3.73894699268512,24.2));
#26738=CARTESIAN_POINT('Origin',(53.0783684845482,7.45967821145951,11.));
#26739=CARTESIAN_POINT('Origin',(53.0783684845482,7.45967821145951,24.2));
#26740=CARTESIAN_POINT('Origin',(40.2834747403675,34.8709542118271,14.5));
#26741=CARTESIAN_POINT('',(40.2774792716873,34.9040806293113,11.2969997378715));
#26742=CARTESIAN_POINT('',(40.2069473082991,35.2937868207374,11.5));
#26743=CARTESIAN_POINT('Ctrl Pts',(40.2774792716873,34.9040806293113,11.2969997378715));
#26744=CARTESIAN_POINT('Ctrl Pts',(40.2422803237447,35.0985633473016,11.3977655520825));
#26745=CARTESIAN_POINT('Ctrl Pts',(40.2069473082991,35.2937868207374,11.5));
#26746=CARTESIAN_POINT('',(40.2069473082991,35.2937868207374,24.2));
#26747=CARTESIAN_POINT('',(40.2069473082991,35.2937868207374,14.5));
#26748=CARTESIAN_POINT('',(40.3600021724359,34.4481216029168,24.2));
#26749=CARTESIAN_POINT('',(40.332375372345,34.600766368886,24.2));
#26750=CARTESIAN_POINT('',(40.3600021724359,34.4481216029168,11.5));
#26751=CARTESIAN_POINT('',(40.3600021724359,34.4481216029168,14.5));
#26752=CARTESIAN_POINT('Ctrl Pts',(40.3600021724359,34.4481216029168,11.5));
#26753=CARTESIAN_POINT('Ctrl Pts',(40.3239659771285,34.6472303155083,11.4654707447276));
#26754=CARTESIAN_POINT('Ctrl Pts',(40.2774792716873,34.9040806293113,11.2969997378715));
#26755=CARTESIAN_POINT('Origin',(41.0599821511772,34.4534158791985,11.25));
#26756=CARTESIAN_POINT('',(40.9332180591367,33.7649895106091,11.5));
#26757=CARTESIAN_POINT('Origin',(41.0599821511772,34.4534158791985,11.5));
#26758=CARTESIAN_POINT('',(41.3679200920551,33.6045438641267,11.2969997378715));
#26759=CARTESIAN_POINT('Ctrl Pts',(41.3679200920551,33.6045438641267,11.2969997378715));
#26760=CARTESIAN_POINT('Ctrl Pts',(41.1230442433439,33.6949259209821,11.4654707447276));
#26761=CARTESIAN_POINT('Ctrl Pts',(40.9332180591367,33.7649895106091,11.5));
#26762=CARTESIAN_POINT('Ctrl Pts',(41.3679200920551,33.6045438641267,11.2969997378715));
#26763=CARTESIAN_POINT('Ctrl Pts',(41.3357200249272,33.4883281512132,11.1987310576086));
#26764=CARTESIAN_POINT('Ctrl Pts',(41.2968973614675,33.3748667810618,11.0971961933879));
#26765=CARTESIAN_POINT('Ctrl Pts',(41.2568614319233,33.2696766558841,11.));
#26766=CARTESIAN_POINT('Ctrl Pts',(40.2774792716873,34.9040806293113,11.2969997378715));
#26767=CARTESIAN_POINT('Ctrl Pts',(40.1574376536108,34.8925504003199,11.1987310576086));
#26768=CARTESIAN_POINT('Ctrl Pts',(40.0389585318563,34.8740199005147,11.0971961933879));
#26769=CARTESIAN_POINT('Ctrl Pts',(39.9284143148345,34.8528582802461,11.));
#26770=CARTESIAN_POINT('Origin',(41.0599821511772,34.4534158791985,11.));
#26771=CARTESIAN_POINT('',(40.9332180591367,33.7649895106091,24.2));
#26772=CARTESIAN_POINT('Origin',(41.0599821511772,34.4534158791985,24.2));
#26773=CARTESIAN_POINT('',(40.9332180591367,33.7649895106091,14.5));
#26774=CARTESIAN_POINT('Origin',(41.3363380414977,33.6162005901946,14.5));
#26775=CARTESIAN_POINT('',(41.7394580238587,33.4674116697801,24.2));
#26776=CARTESIAN_POINT('',(41.0787464646293,33.7112759382477,24.2));
#26777=CARTESIAN_POINT('',(41.7394580238587,33.4674116697801,11.5));
#26778=CARTESIAN_POINT('',(41.7394580238587,33.4674116697801,14.5));
#26779=CARTESIAN_POINT('Ctrl Pts',(41.7394580238587,33.4674116697801,11.5));
#26780=CARTESIAN_POINT('Ctrl Pts',(41.5533359473942,33.5361080977276,11.3977655520833));
#26781=CARTESIAN_POINT('Ctrl Pts',(41.3679200920551,33.6045438641267,11.2969997378715));
#26782=CARTESIAN_POINT('Origin',(42.6178210224504,31.9759771719264,14.5));
#26783=CARTESIAN_POINT('',(42.614150940502,32.0094411178763,11.2969997378715));
#26784=CARTESIAN_POINT('',(42.5709753191419,32.4031180656586,11.5));
#26785=CARTESIAN_POINT('Ctrl Pts',(42.614150940502,32.0094411178763,11.2969997378715));
#26786=CARTESIAN_POINT('Ctrl Pts',(42.5926041640387,32.2059054402286,11.3977655520829));
#26787=CARTESIAN_POINT('Ctrl Pts',(42.5709753191419,32.4031180656586,11.5));
#26788=CARTESIAN_POINT('',(42.5709753191419,32.4031180656586,24.2));
#26789=CARTESIAN_POINT('',(42.5709753191419,32.4031180656586,14.5));
#26790=CARTESIAN_POINT('',(42.6646667257588,31.5488362781942,24.2));
#26791=CARTESIAN_POINT('',(42.6477551837739,31.7030363573407,24.2));
#26792=CARTESIAN_POINT('',(42.6646667257588,31.5488362781942,11.5));
#26793=CARTESIAN_POINT('',(42.6646667257588,31.5488362781942,14.5));
#26794=CARTESIAN_POINT('Ctrl Pts',(42.6646667257588,31.5488362781942,11.5));
#26795=CARTESIAN_POINT('Ctrl Pts',(42.6426074344941,31.7499737298808,11.4654707447276));
#26796=CARTESIAN_POINT('Ctrl Pts',(42.614150940502,32.0094411178763,11.2969997378715));
#26797=CARTESIAN_POINT('Origin',(43.3633108984972,31.5052895228766,11.25));
#26798=CARTESIAN_POINT('',(43.1888334015084,30.827382742379,11.5));
#26799=CARTESIAN_POINT('Origin',(43.3633108984972,31.5052895228766,11.5));
#26800=CARTESIAN_POINT('',(43.6112843995965,30.6370046524817,11.2969997378715));
#26801=CARTESIAN_POINT('Ctrl Pts',(43.6112843995965,30.6370046524817,11.2969997378715));
#26802=CARTESIAN_POINT('Ctrl Pts',(43.3733097897213,30.7442482189004,11.4654707447276));
#26803=CARTESIAN_POINT('Ctrl Pts',(43.1888334015084,30.827382742379,11.5));
#26804=CARTESIAN_POINT('Ctrl Pts',(43.6112843995965,30.6370046524817,11.2969997378715));
#26805=CARTESIAN_POINT('Ctrl Pts',(43.5710559718872,30.523318198341,11.1987310576087));
#26806=CARTESIAN_POINT('Ctrl Pts',(43.5244132133966,30.412841346489,11.0971961933879));
#26807=CARTESIAN_POINT('Ctrl Pts',(43.4771371171594,30.3107002244375,11.));
#26808=CARTESIAN_POINT('Ctrl Pts',(42.614150940502,32.0094411178763,11.2969997378715));
#26809=CARTESIAN_POINT('Ctrl Pts',(42.4935974296579,32.0063126559227,11.1987310576087));
#26810=CARTESIAN_POINT('Ctrl Pts',(42.3741142947662,31.9960919812296,11.0971961933879));
#26811=CARTESIAN_POINT('Ctrl Pts',(42.2623631978924,31.9826930843766,11.));
#26812=CARTESIAN_POINT('Origin',(43.3633108984972,31.5052895228766,11.));
#26813=CARTESIAN_POINT('',(43.1888334015084,30.827382742379,24.2));
#26814=CARTESIAN_POINT('Origin',(43.3633108984972,31.5052895228766,24.2));
#26815=CARTESIAN_POINT('',(43.1888334015084,30.827382742379,14.5));
#26816=CARTESIAN_POINT('Origin',(43.5805924134327,30.6508360358314,14.5));
#26817=CARTESIAN_POINT('',(43.9723514253571,30.4742893292837,24.2));
#26818=CARTESIAN_POINT('',(43.3302604377194,30.7636484651835,24.2));
#26819=CARTESIAN_POINT('',(43.9723514253571,30.4742893292837,11.5));
#26820=CARTESIAN_POINT('',(43.9723514253571,30.4742893292837,14.5));
#26821=CARTESIAN_POINT('Ctrl Pts',(43.9723514253571,30.4742893292837,11.5));
#26822=CARTESIAN_POINT('Ctrl Pts',(43.7914747534882,30.5558016359257,11.397765552083));
#26823=CARTESIAN_POINT('Ctrl Pts',(43.6112843995965,30.6370046524817,11.2969997378715));
#26824=CARTESIAN_POINT('Origin',(44.74453756444,28.9252163854584,14.5));
#26825=CARTESIAN_POINT('',(44.7432107494939,28.9588548268927,11.2969997378715));
#26826=CARTESIAN_POINT('',(44.727601817449,29.3545845765144,11.5));
#26827=CARTESIAN_POINT('Ctrl Pts',(44.7432107494939,28.9588548268927,11.2969997378715));
#26828=CARTESIAN_POINT('Ctrl Pts',(44.7354211182387,29.156343599178,11.3977655520835));
#26829=CARTESIAN_POINT('Ctrl Pts',(44.727601817449,29.3545845765144,11.5));
#26830=CARTESIAN_POINT('',(44.727601817449,29.3545845765144,24.2));
#26831=CARTESIAN_POINT('',(44.727601817449,29.3545845765144,14.5));
#26832=CARTESIAN_POINT('',(44.7614733114311,28.4958481944023,24.2));
#26833=CARTESIAN_POINT('',(44.7553594188847,28.6508523394404,24.2));
#26834=CARTESIAN_POINT('',(44.7614733114311,28.4958481944023,11.5));
#26835=CARTESIAN_POINT('',(44.7614733114311,28.4958481944023,14.5));
#26836=CARTESIAN_POINT('Ctrl Pts',(44.7614733114311,28.4958481944023,11.5));
#26837=CARTESIAN_POINT('Ctrl Pts',(44.7534983948587,28.6980344637377,11.4654707447276));
#26838=CARTESIAN_POINT('Ctrl Pts',(44.7432107494939,28.9588548268927,11.2969997378715));
#26839=CARTESIAN_POINT('Origin',(45.4553779539844,28.4036725628998,11.25));
#26840=CARTESIAN_POINT('',(45.2340370888744,27.7395880641857,11.5));
#26841=CARTESIAN_POINT('Origin',(45.4553779539844,28.4036725628998,11.5));
#26842=CARTESIAN_POINT('',(45.6421789133341,27.5202050337906,11.2969997378715));
#26843=CARTESIAN_POINT('Ctrl Pts',(45.6421789133341,27.5202050337906,11.2969997378715));
#26844=CARTESIAN_POINT('Ctrl Pts',(45.4122649306731,27.6437876298971,11.4654707447276));
#26845=CARTESIAN_POINT('Ctrl Pts',(45.2340370888744,27.7395880641857,11.5));
#26846=CARTESIAN_POINT('Ctrl Pts',(45.6421789133341,27.5202050337906,11.2969997378715));
#26847=CARTESIAN_POINT('Ctrl Pts',(45.5941181138995,27.4096017073997,11.1987310576086));
#26848=CARTESIAN_POINT('Ctrl Pts',(45.5398824992087,27.3026476059642,11.0971961933879));
#26849=CARTESIAN_POINT('Ctrl Pts',(45.4855965606673,27.2040531083184,11.));
#26850=CARTESIAN_POINT('Ctrl Pts',(44.7432107494939,28.9588548268927,11.2969997378715));
#26851=CARTESIAN_POINT('Ctrl Pts',(44.6227326704691,28.9641433735292,11.1987310576086));
#26852=CARTESIAN_POINT('Ctrl Pts',(44.5028276322628,28.9622823180478,11.0971961933879));
#26853=CARTESIAN_POINT('Ctrl Pts',(44.390414095648,28.9567114226892,11.));
#26854=CARTESIAN_POINT('Origin',(45.4553779539844,28.4036725628998,11.));
#26855=CARTESIAN_POINT('',(45.2340370888744,27.7395880641857,24.2));
#26856=CARTESIAN_POINT('Origin',(45.4553779539844,28.4036725628998,24.2));
#26857=CARTESIAN_POINT('',(45.2340370888744,27.7395880641857,14.5));
#26858=CARTESIAN_POINT('Origin',(45.6125265198356,27.5361436893125,14.5));
#26859=CARTESIAN_POINT('',(45.9910159507968,27.3326993144394,24.2));
#26860=CARTESIAN_POINT('',(45.3706737374995,27.6661435891479,24.2));
#26861=CARTESIAN_POINT('',(45.9910159507968,27.3326993144394,11.5));
#26862=CARTESIAN_POINT('',(45.9910159507968,27.3326993144394,14.5));
#26863=CARTESIAN_POINT('Ctrl Pts',(45.9910159507968,27.3326993144394,11.5));
#26864=CARTESIAN_POINT('Ctrl Pts',(45.8162658964868,27.426630380012,11.3977655520824));
#26865=CARTESIAN_POINT('Ctrl Pts',(45.6421789133341,27.5202050337906,11.2969997378715));
#26866=CARTESIAN_POINT('Origin',(46.653263217121,25.7335348523128,14.5));
#26867=CARTESIAN_POINT('',(46.6542861332861,25.7671839061264,11.2969997378715));
#26868=CARTESIAN_POINT('',(46.6663199357044,26.1630385020257,11.5));
#26869=CARTESIAN_POINT('Ctrl Pts',(46.6542861332861,25.7671839061264,11.2969997378715));
#26870=CARTESIAN_POINT('Ctrl Pts',(46.6602915975398,25.964734982895,11.3977655520828));
#26871=CARTESIAN_POINT('Ctrl Pts',(46.6663199357044,26.1630385020257,11.5));
#26872=CARTESIAN_POINT('',(46.6663199357044,26.1630385020257,24.2));
#26873=CARTESIAN_POINT('',(46.6663199357044,26.1630385020257,14.5));
#26874=CARTESIAN_POINT('',(46.6402064985376,25.3040312025999,24.2));
#26875=CARTESIAN_POINT('',(46.6449200416998,25.459084248916,24.2));
#26876=CARTESIAN_POINT('',(46.6402064985376,25.3040312025999,11.5));
#26877=CARTESIAN_POINT('',(46.6402064985376,25.3040312025999,14.5));
#26878=CARTESIAN_POINT('Ctrl Pts',(46.6402064985376,25.3040312025999,11.5));
#26879=CARTESIAN_POINT('Ctrl Pts',(46.6463548096495,25.5062812584034,11.4654707447275));
#26880=CARTESIAN_POINT('Ctrl Pts',(46.6542861332861,25.7671839061264,11.2969997378715));
#26881=CARTESIAN_POINT('Origin',(47.3259909772385,25.1636757653237,11.25));
#26882=CARTESIAN_POINT('',(47.0588650944529,24.5166489013173,11.5));
#26883=CARTESIAN_POINT('Origin',(47.3259909772385,25.1636757653237,11.5));
#26884=CARTESIAN_POINT('',(47.4507093193416,24.2693297424963,11.2969997378715));
#26885=CARTESIAN_POINT('Ctrl Pts',(47.4507093193416,24.2693297424963,11.2969997378715));
#26886=CARTESIAN_POINT('Ctrl Pts',(47.2299760817075,24.4086492863048,11.4654707447276));
#26887=CARTESIAN_POINT('Ctrl Pts',(47.0588650944529,24.5166489013173,11.5));
#26888=CARTESIAN_POINT('Ctrl Pts',(47.4507093193416,24.2693297424963,11.2969997378714));
#26889=CARTESIAN_POINT('Ctrl Pts',(47.3950502955655,24.1623483921434,11.1987310576086));
#26890=CARTESIAN_POINT('Ctrl Pts',(47.3334860551377,24.0594381107558,11.0971961933879));
#26891=CARTESIAN_POINT('Ctrl Pts',(47.2724547499278,23.9648705799974,11.));
#26892=CARTESIAN_POINT('Ctrl Pts',(46.6542861332861,25.7671839061264,11.2969997378715));
#26893=CARTESIAN_POINT('Ctrl Pts',(46.5344704431712,25.7808636960853,11.1987310576086));
#26894=CARTESIAN_POINT('Ctrl Pts',(46.4147276669439,25.787371326691,11.0971961933879));
#26895=CARTESIAN_POINT('Ctrl Pts',(46.3021993580384,25.7896555736688,11.));
#26896=CARTESIAN_POINT('Origin',(47.3259909772385,25.1636757653237,11.));
#26897=CARTESIAN_POINT('',(47.0588650944529,24.5166489013173,24.2));
#26898=CARTESIAN_POINT('Origin',(47.3259909772385,25.1636757653237,24.2));
#26899=CARTESIAN_POINT('',(47.0588650944529,24.5166489013173,14.5));
#26900=CARTESIAN_POINT('Origin',(47.4222409819888,24.287298018663,14.5));
#26901=CARTESIAN_POINT('',(47.7856168695248,24.0579471360087,24.2));
#26902=CARTESIAN_POINT('',(47.1900456754746,24.4338520425371,24.2));
#26903=CARTESIAN_POINT('',(47.7856168695248,24.0579471360087,11.5));
#26904=CARTESIAN_POINT('',(47.7856168695248,24.0579471360087,14.5));
#26905=CARTESIAN_POINT('Ctrl Pts',(47.7856168695248,24.0579471360087,11.5));
#26906=CARTESIAN_POINT('Ctrl Pts',(47.6178447974735,24.1638393378018,11.3977655520823));
#26907=CARTESIAN_POINT('Ctrl Pts',(47.4507093193416,24.2693297424963,11.2969997378715));
#26908=CARTESIAN_POINT('Origin',(48.3346988609778,22.4164821240926,14.5));
#26909=CARTESIAN_POINT('',(48.3380665247094,22.4499778554777,11.2969997378715));
#26910=CARTESIAN_POINT('',(48.3776844341152,22.8440287338545,11.5));
#26911=CARTESIAN_POINT('Ctrl Pts',(48.3380665247094,22.4499778554777,11.2969997378715));
#26912=CARTESIAN_POINT('Ctrl Pts',(48.3578378264538,22.646628787743,11.397765552083));
#26913=CARTESIAN_POINT('Ctrl Pts',(48.3776844341152,22.8440287338545,11.5));
#26914=CARTESIAN_POINT('',(48.3776844341152,22.8440287338545,24.2));
#26915=CARTESIAN_POINT('',(48.3776844341152,22.8440287338545,14.5));
#26916=CARTESIAN_POINT('',(48.2917132878405,21.9889355143307,24.2));
#26917=CARTESIAN_POINT('',(48.3072313028027,22.1432820590691,24.2));
#26918=CARTESIAN_POINT('',(48.2917132878405,21.9889355143307,11.5));
#26919=CARTESIAN_POINT('',(48.2917132878405,21.9889355143307,14.5));
#26920=CARTESIAN_POINT('Ctrl Pts',(48.2917132878405,21.9889355143307,11.5));
#26921=CARTESIAN_POINT('Ctrl Pts',(48.3119548726829,22.1902640146607,11.4654707447276));
#26922=CARTESIAN_POINT('Ctrl Pts',(48.3380665247094,22.4499778554777,11.2969997378715));
#26923=CARTESIAN_POINT('Origin',(48.9660365296434,21.8010840688629,11.25));
#26924=CARTESIAN_POINT('',(48.6544270396318,21.1742670894066,11.5));
#26925=CARTESIAN_POINT('Origin',(48.9660365296434,21.8010840688629,11.5));
#26926=CARTESIAN_POINT('',(49.028064639274,20.9002167162411,11.2969997378715));
#26927=CARTESIAN_POINT('Ctrl Pts',(49.028064639274,20.9002167162411,11.2969997378715));
#26928=CARTESIAN_POINT('Ctrl Pts',(48.8175875368124,21.0545944569385,11.4654707447276));
#26929=CARTESIAN_POINT('Ctrl Pts',(48.6544270396318,21.1742670894066,11.5));
#26930=CARTESIAN_POINT('Ctrl Pts',(49.028064639274,20.9002167162411,11.2969997378715));
#26931=CARTESIAN_POINT('Ctrl Pts',(48.9650785563254,20.7973785443115,11.1987310576086));
#26932=CARTESIAN_POINT('Ctrl Pts',(48.8964856249514,20.699013451518,11.0971961933879));
#26933=CARTESIAN_POINT('Ctrl Pts',(48.8290062914572,20.608933611151,11.));
#26934=CARTESIAN_POINT('Ctrl Pts',(48.3380665247094,22.4499778554777,11.2969997378715));
#26935=CARTESIAN_POINT('Ctrl Pts',(48.2194969535028,22.4719822421975,11.1987310576086));
#26936=CARTESIAN_POINT('Ctrl Pts',(48.1004998140235,22.4868268543681,11.0971961933879));
#26937=CARTESIAN_POINT('Ctrl Pts',(47.9884049594373,22.4969551150606,11.));
#26938=CARTESIAN_POINT('Origin',(48.9660365296434,21.8010840688629,11.));
#26939=CARTESIAN_POINT('',(48.6544270396318,21.1742670894066,24.2));
#26940=CARTESIAN_POINT('Origin',(48.9660365296434,21.8010840688629,24.2));
#26941=CARTESIAN_POINT('',(48.6544270396318,21.1742670894066,14.5));
#26942=CARTESIAN_POINT('Origin',(49.0009190529448,20.9201270734172,14.5));
#26943=CARTESIAN_POINT('',(49.3474110662579,20.6659870574277,24.2));
#26944=CARTESIAN_POINT('',(48.7795124544456,21.0825212248573,24.2));
#26945=CARTESIAN_POINT('',(49.3474110662579,20.6659870574277,11.5));
#26946=CARTESIAN_POINT('',(49.3474110662579,20.6659870574277,14.5));
#26947=CARTESIAN_POINT('Ctrl Pts',(49.3474110662579,20.6659870574277,11.5));
#26948=CARTESIAN_POINT('Ctrl Pts',(49.1874343451369,20.7833244992778,11.3977655520829));
#26949=CARTESIAN_POINT('Ctrl Pts',(49.028064639274,20.9002167162411,11.2969997378715));
#26950=CARTESIAN_POINT('Origin',(49.7806527105708,18.9902185482608,14.5));
#26951=CARTESIAN_POINT('',(49.7863487149497,19.0233977693811,11.2969997378715));
#26952=CARTESIAN_POINT('',(49.8533577168707,19.4137251539658,11.5));
#26953=CARTESIAN_POINT('Ctrl Pts',(49.7863487149497,19.0233977693811,11.2969997378715));
#26954=CARTESIAN_POINT('Ctrl Pts',(49.8197895303901,19.2181904935678,11.3977655520829));
#26955=CARTESIAN_POINT('Ctrl Pts',(49.8533577168707,19.4137251539658,11.5));
#26956=CARTESIAN_POINT('',(49.8533577168707,19.4137251539658,24.2));
#26957=CARTESIAN_POINT('',(49.8533577168707,19.4137251539658,14.5));
#26958=CARTESIAN_POINT('',(49.707947704271,18.5667119425558,24.2));
#26959=CARTESIAN_POINT('',(49.7341945888243,18.7196000248653,24.2));
#26960=CARTESIAN_POINT('',(49.707947704271,18.5667119425558,11.5));
#26961=CARTESIAN_POINT('',(49.707947704271,18.5667119425558,14.5));
#26962=CARTESIAN_POINT('Ctrl Pts',(49.707947704271,18.5667119425558,11.5));
#26963=CARTESIAN_POINT('Ctrl Pts',(49.7421839478772,18.7661380351961,11.4654707447276));
#26964=CARTESIAN_POINT('Ctrl Pts',(49.7863487149497,19.0233977693811,11.2969997378715));
#26965=CARTESIAN_POINT('Origin',(50.3675244741247,18.3322796822558,11.25));
#26966=CARTESIAN_POINT('',(50.0129495069995,17.7287263766662,11.5));
#26967=CARTESIAN_POINT('Origin',(50.3675244741247,18.3322796822558,11.5));
#26968=CARTESIAN_POINT('',(50.3665601565676,17.4292799350267,11.2969997378715));
#26969=CARTESIAN_POINT('Ctrl Pts',(50.3665601565676,17.4292799350267,11.2969997378715));
#26970=CARTESIAN_POINT('Ctrl Pts',(50.1673646125648,17.5979637597785,11.4654707447276));
#26971=CARTESIAN_POINT('Ctrl Pts',(50.0129495069995,17.7287263766662,11.5));
#26972=CARTESIAN_POINT('Ctrl Pts',(50.3665601565676,17.4292799350267,11.2969997378715));
#26973=CARTESIAN_POINT('Ctrl Pts',(50.2965538763113,17.3310859587567,11.1987310576086));
#26974=CARTESIAN_POINT('Ctrl Pts',(50.2212664318579,17.2377452794019,11.0971961933879));
#26975=CARTESIAN_POINT('Ctrl Pts',(50.1476678226092,17.1525919893539,11.));
#26976=CARTESIAN_POINT('Ctrl Pts',(49.7863487149497,19.0233977693811,11.2969997378715));
#26977=CARTESIAN_POINT('Ctrl Pts',(49.6696029216838,19.0536195497014,11.1987310576086));
#26978=CARTESIAN_POINT('Ctrl Pts',(49.5519311610546,19.0767288219785,11.0971961933879));
#26979=CARTESIAN_POINT('Ctrl Pts',(49.4408158756514,19.0946517525179,11.));
#26980=CARTESIAN_POINT('Origin',(50.3675244741247,18.3322796822558,11.));
#26981=CARTESIAN_POINT('',(50.0129495069995,17.7287263766662,24.2));
#26982=CARTESIAN_POINT('Origin',(50.3675244741247,18.3322796822558,24.2));
#26983=CARTESIAN_POINT('',(50.0129495069995,17.7287263766662,14.5));
#26984=CARTESIAN_POINT('Origin',(50.34086957183,17.4510353719535,14.5));
#26985=CARTESIAN_POINT('',(50.6687896366606,17.1733443672407,24.2));
#26986=CARTESIAN_POINT('',(50.131330352038,17.6284784829776,24.2));
#26987=CARTESIAN_POINT('',(50.6687896366606,17.1733443672407,11.5));
#26988=CARTESIAN_POINT('',(50.6687896366606,17.1733443672407,14.5));
#26989=CARTESIAN_POINT('Ctrl Pts',(50.6687896366606,17.1733443672407,11.5));
#26990=CARTESIAN_POINT('Ctrl Pts',(50.5173876569737,17.3015553929261,11.3977655520831));
#26991=CARTESIAN_POINT('Ctrl Pts',(50.3665601565676,17.4292799350267,11.2969997378715));
#26992=CARTESIAN_POINT('Origin',(50.9840802240917,15.4714365365517,14.5));
#26993=CARTESIAN_POINT('',(50.9920768187572,15.5041376015772,11.2969997378715));
#26994=CARTESIAN_POINT('',(51.0861504520718,15.8888398565875,11.5));
#26995=CARTESIAN_POINT('Ctrl Pts',(50.9920768187572,15.5041376015772,11.2969997378715));
#26996=CARTESIAN_POINT('Ctrl Pts',(51.0390242276023,15.6961231071139,11.3977655520831));
#26997=CARTESIAN_POINT('Ctrl Pts',(51.0861504520718,15.8888398565875,11.5));
#26998=CARTESIAN_POINT('',(51.0861504520718,15.8888398565875,24.2));
#26999=CARTESIAN_POINT('',(51.0861504520718,15.8888398565875,14.5));
#27000=CARTESIAN_POINT('',(50.8820099961117,15.054033216516,24.2));
#27001=CARTESIAN_POINT('',(50.9188578780728,15.204717981028,24.2));
#27002=CARTESIAN_POINT('',(50.8820099961117,15.054033216516,11.5));
#27003=CARTESIAN_POINT('',(50.8820099961117,15.054033216516,14.5));
#27004=CARTESIAN_POINT('Ctrl Pts',(50.8820099961117,15.054033216516,11.5));
#27005=CARTESIAN_POINT('Ctrl Pts',(50.9300741029444,15.2505853175896,11.4654707447276));
#27006=CARTESIAN_POINT('Ctrl Pts',(50.9920768187572,15.5041376015772,11.2969997378715));
#27007=CARTESIAN_POINT('Origin',(51.5236269022939,14.7741622717912,11.25));
#27008=CARTESIAN_POINT('',(51.1278139116531,14.1968130911041,11.5));
#27009=CARTESIAN_POINT('Origin',(51.5236269022939,14.7741622717912,11.5));
#27010=CARTESIAN_POINT('',(51.4596748556074,13.8734294539541,11.2969997378715));
#27011=CARTESIAN_POINT('Ctrl Pts',(51.4596748556075,13.8734294539541,11.2969997378715));
#27012=CARTESIAN_POINT('Ctrl Pts',(51.2727313307305,14.0555975521219,11.4654707447276));
#27013=CARTESIAN_POINT('Ctrl Pts',(51.1278139116531,14.1968130911041,11.5));
#27014=CARTESIAN_POINT('Ctrl Pts',(51.4596748556074,13.8734294539541,11.2969997378715));
#27015=CARTESIAN_POINT('Ctrl Pts',(51.3829894416038,13.7803580645257,11.1987310576087));
#27016=CARTESIAN_POINT('Ctrl Pts',(51.3013742769325,13.6924965450168,11.0971961933879));
#27017=CARTESIAN_POINT('Ctrl Pts',(51.2220149569554,13.6126846635571,11.));
#27018=CARTESIAN_POINT('Ctrl Pts',(50.9920768187572,15.5041376015772,11.2969997378715));
#27019=CARTESIAN_POINT('Ctrl Pts',(50.8777235772014,15.5424295380224,11.1987310576087));
#27020=CARTESIAN_POINT('Ctrl Pts',(50.7619504804118,15.5736908843544,11.0971961933879));
#27021=CARTESIAN_POINT('Ctrl Pts',(50.6523561066928,15.5993211660246,11.));
#27022=CARTESIAN_POINT('Origin',(51.5236269022939,14.7741622717912,11.));
#27023=CARTESIAN_POINT('',(51.1278139116531,14.1968130911041,24.2));
#27024=CARTESIAN_POINT('Origin',(51.5236269022939,14.7741622717912,24.2));
#27025=CARTESIAN_POINT('',(51.1278139116531,14.1968130911041,14.5));
#27026=CARTESIAN_POINT('Origin',(51.9391184236626,11.8772792412203,14.5));
#27027=CARTESIAN_POINT('',(51.8081802498931,11.4680127538715,11.0622545443403));
#27028=CARTESIAN_POINT('',(52.0700565974321,12.286545728569,11.5));
#27029=CARTESIAN_POINT('Ctrl Pts',(51.8081802498931,11.4680127538715,11.0622545443403));
#27030=CARTESIAN_POINT('Ctrl Pts',(51.9385805447408,11.8755980216752,11.2776618075205));
#27031=CARTESIAN_POINT('Ctrl Pts',(52.0700565974321,12.286545728569,11.5));
#27032=CARTESIAN_POINT('',(52.0700565974321,12.286545728569,24.2));
#27033=CARTESIAN_POINT('',(52.0700565974321,12.286545728569,14.5));
#27034=CARTESIAN_POINT('',(51.8081802498931,11.4680127538716,24.2));
#27035=CARTESIAN_POINT('',(51.8554496100851,11.6157600795601,24.2));
#27036=CARTESIAN_POINT('',(51.8081802498931,11.4680127538716,14.5));
#27037=CARTESIAN_POINT('Origin',(0.,0.,14.5));
#27038=CARTESIAN_POINT('',(51.7433149571623,13.5970348695554,11.5));
#27039=CARTESIAN_POINT('Origin',(0.,0.,11.5));
#27040=CARTESIAN_POINT('',(51.7433149571623,13.5970348695554,24.2));
#27041=CARTESIAN_POINT('',(51.7433149571623,13.5970348695554,14.5));
#27042=CARTESIAN_POINT('Origin',(0.,0.,24.2));
#27043=CARTESIAN_POINT('Origin',(0.,0.,11.25));
#27044=CARTESIAN_POINT('Ctrl Pts',(51.766094205967,11.3697621197168,11.));
#27045=CARTESIAN_POINT('Ctrl Pts',(51.7780926618965,11.4049882694565,11.0192759649605));
#27046=CARTESIAN_POINT('Ctrl Pts',(51.7924945631287,11.4379662231208,11.0404458048696));
#27047=CARTESIAN_POINT('Ctrl Pts',(51.8081802498931,11.4680127538714,11.0622545443403));
#27048=CARTESIAN_POINT('Ctrl Pts',(51.7433149571623,13.5970348695554,11.5));
#27049=CARTESIAN_POINT('Ctrl Pts',(51.6012253341355,13.7354948478468,11.3977655520831));
#27050=CARTESIAN_POINT('Ctrl Pts',(51.4596748556074,13.8734294539541,11.2969997378715));
#27051=CARTESIAN_POINT('Origin',(51.4355644344077,13.8969239803297,14.5));
#27052=CARTESIAN_POINT('',(51.238913447339,14.0885515659373,24.2));
#27053=CARTESIAN_POINT('Origin',(33.443838774836,41.4759138875076,14.5));
#27054=CARTESIAN_POINT('',(33.8690845744085,41.4141897191236,24.2));
#27055=CARTESIAN_POINT('',(33.0185929752635,41.5376380558916,24.2));
#27056=CARTESIAN_POINT('',(33.1721089155843,41.5153553108074,24.2));
#27057=CARTESIAN_POINT('',(33.8690845744085,41.4141897191236,11.5));
#27058=CARTESIAN_POINT('',(33.8690845744085,41.4141897191236,14.5));
#27059=CARTESIAN_POINT('',(33.0185929752634,41.5376380558916,11.0622545443402));
#27060=CARTESIAN_POINT('Ctrl Pts',(33.8690845744085,41.4141897191236,11.5));
#27061=CARTESIAN_POINT('Ctrl Pts',(33.4420919141158,41.4761674432754,11.2776618075192));
#27062=CARTESIAN_POINT('Ctrl Pts',(33.0185929752634,41.5376380558916,11.0622545443402));
#27063=CARTESIAN_POINT('',(33.0185929752635,41.5376380558916,14.5));
#27064=CARTESIAN_POINT('Origin',(0.,0.,11.25));
#27065=CARTESIAN_POINT('',(34.9037103045182,40.546035650582,11.5));
#27066=CARTESIAN_POINT('Origin',(0.,0.,11.5));
#27067=CARTESIAN_POINT('',(35.0277924748111,40.1699382050837,11.2969997378715));
#27068=CARTESIAN_POINT('Ctrl Pts',(35.0277924748111,40.1699382050837,11.2969997378715));
#27069=CARTESIAN_POINT('Ctrl Pts',(34.9658693176643,40.3576294838962,11.3977655520829));
#27070=CARTESIAN_POINT('Ctrl Pts',(34.9037103045182,40.546035650582,11.5));
#27071=CARTESIAN_POINT('Ctrl Pts',(35.0277924748111,40.1699382050837,11.2969997378715));
#27072=CARTESIAN_POINT('Ctrl Pts',(34.9105237912333,40.1418136232562,11.1987310576086));
#27073=CARTESIAN_POINT('Ctrl Pts',(34.7957766472675,40.1069743542277,11.0971961933879));
#27074=CARTESIAN_POINT('Ctrl Pts',(34.6892533672809,40.0706338959167,11.));
#27075=CARTESIAN_POINT('Ctrl Pts',(33.0185929752633,41.5376380558916,11.0622545443403));
#27076=CARTESIAN_POINT('Ctrl Pts',(32.9847111798176,41.5367113861579,11.0404458048696));
#27077=CARTESIAN_POINT('Ctrl Pts',(32.948757413446,41.5382236264416,11.0192759649605));
#27078=CARTESIAN_POINT('Ctrl Pts',(32.9118365829004,41.5428816133457,11.));
#27079=CARTESIAN_POINT('Origin',(0.,0.,14.5));
#27080=CARTESIAN_POINT('',(34.9037103045182,40.546035650582,24.2));
#27081=CARTESIAN_POINT('Origin',(0.,0.,24.2));
#27082=CARTESIAN_POINT('',(34.9037103045182,40.546035650582,14.5));
#27083=CARTESIAN_POINT('Origin',(35.0383399022473,40.137968579585,14.5));
#27084=CARTESIAN_POINT('',(35.1729694999764,39.729901508588,24.2));
#27085=CARTESIAN_POINT('',(35.1243675165795,39.8772158387497,24.2));
#27086=CARTESIAN_POINT('',(35.1729694999764,39.729901508588,11.5));
#27087=CARTESIAN_POINT('',(35.1729694999764,39.729901508588,14.5));
#27088=CARTESIAN_POINT('Ctrl Pts',(35.1729694999764,39.729901508588,11.5));
#27089=CARTESIAN_POINT('Ctrl Pts',(35.1095734294849,39.9220572398279,11.4654707447276));
#27090=CARTESIAN_POINT('Ctrl Pts',(35.0277924748111,40.1699382050837,11.2969997378715));
#27091=CARTESIAN_POINT('Origin',(36.2555847625695,39.0419563844502,14.5));
#27092=CARTESIAN_POINT('',(36.6754890244158,38.9507189255854,24.2));
#27093=CARTESIAN_POINT('',(35.8356805007232,39.1331938433149,24.2));
#27094=CARTESIAN_POINT('',(35.9872681182067,39.1002566472175,24.2));
#27095=CARTESIAN_POINT('',(36.6754890244158,38.9507189255854,11.5));
#27096=CARTESIAN_POINT('',(36.6754890244158,38.9507189255854,14.5));
#27097=CARTESIAN_POINT('',(36.288481761496,39.0348084727497,11.2969997378715));
#27098=CARTESIAN_POINT('Ctrl Pts',(36.6754890244158,38.9507189255854,11.5));
#27099=CARTESIAN_POINT('Ctrl Pts',(36.4816175803026,38.9928436180797,11.3977655520832));
#27100=CARTESIAN_POINT('Ctrl Pts',(36.288481761496,39.0348084727497,11.2969997378715));
#27101=CARTESIAN_POINT('',(35.8356805007232,39.1331938433149,11.5));
#27102=CARTESIAN_POINT('Ctrl Pts',(36.288481761496,39.0348084727497,11.2969997378715));
#27103=CARTESIAN_POINT('Ctrl Pts',(36.0334102765875,39.0902308064254,11.4654707447276));
#27104=CARTESIAN_POINT('Ctrl Pts',(35.8356805007232,39.1331938433149,11.5));
#27105=CARTESIAN_POINT('',(35.8356805007232,39.1331938433149,14.5));
#27106=CARTESIAN_POINT('Origin',(0.,0.,11.25));
#27107=CARTESIAN_POINT('',(37.6470350917587,38.0125077941444,11.5));
#27108=CARTESIAN_POINT('Origin',(0.,0.,11.5));
#27109=CARTESIAN_POINT('',(37.8587077455022,37.1795791419029,11.0622545443403));
#27110=CARTESIAN_POINT('Ctrl Pts',(37.8587077455022,37.1795791419029,11.0622545443403));
#27111=CARTESIAN_POINT('Ctrl Pts',(37.753306182059,37.5943326805875,11.277661807521));
#27112=CARTESIAN_POINT('Ctrl Pts',(37.6470350917587,38.0125077941444,11.5));
#27113=CARTESIAN_POINT('Ctrl Pts',(37.8750816598377,37.0739556732301,11.));
#27114=CARTESIAN_POINT('Ctrl Pts',(37.8665899121936,37.1101873553899,11.0192759649605));
#27115=CARTESIAN_POINT('Ctrl Pts',(37.861327764173,37.1457860911145,11.0404458048696));
#27116=CARTESIAN_POINT('Ctrl Pts',(37.8587077455022,37.1795791419029,11.0622545443404));
#27117=CARTESIAN_POINT('Ctrl Pts',(36.288481761496,39.0348084727497,11.2969997378715));
#27118=CARTESIAN_POINT('Ctrl Pts',(36.2727691643543,38.9152423799721,11.1987310576087));
#27119=CARTESIAN_POINT('Ctrl Pts',(36.2501150911098,38.7974821376142,11.0971961933879));
#27120=CARTESIAN_POINT('Ctrl Pts',(36.2251084243911,38.6877437910394,11.));
#27121=CARTESIAN_POINT('Origin',(0.,0.,14.5));
#27122=CARTESIAN_POINT('',(37.6470350917587,38.0125077941444,24.2));
#27123=CARTESIAN_POINT('Origin',(0.,0.,24.2));
#27124=CARTESIAN_POINT('',(37.6470350917587,38.0125077941444,14.5));
#27125=CARTESIAN_POINT('Origin',(38.8906971857384,36.4177903943714,14.5));
#27126=CARTESIAN_POINT('',(38.4781801929734,36.5380966439885,11.0622545443404));
#27127=CARTESIAN_POINT('',(38.4781801929734,36.5380966439885,24.2));
#27128=CARTESIAN_POINT('',(38.4781801929734,36.5380966439885,14.5));
#27129=CARTESIAN_POINT('',(39.3032141785034,36.2974841447543,24.2));
#27130=CARTESIAN_POINT('',(38.6271009679847,36.4946654635865,24.2));
#27131=CARTESIAN_POINT('',(39.3032141785034,36.2974841447543,11.5));
#27132=CARTESIAN_POINT('',(39.3032141785034,36.2974841447543,14.5));
#27133=CARTESIAN_POINT('Ctrl Pts',(39.3032141785034,36.2974841447543,11.5));
#27134=CARTESIAN_POINT('Ctrl Pts',(39.0288731206038,36.3774928337799,11.352740724575));
#27135=CARTESIAN_POINT('Ctrl Pts',(38.7538500369047,36.4577004284687,11.2067970124648));
#27136=CARTESIAN_POINT('Ctrl Pts',(38.4781801929734,36.5380966439885,11.0622545443404));
#27137=CARTESIAN_POINT('Origin',(0.,0.,11.25));
#27138=CARTESIAN_POINT('Ctrl Pts',(38.3731925086332,36.5581467896744,11.));
#27139=CARTESIAN_POINT('Ctrl Pts',(38.4091053726145,36.548395853148,11.0192757561174));
#27140=CARTESIAN_POINT('Ctrl Pts',(38.4444995059675,36.54189438867,11.0404460254343));
#27141=CARTESIAN_POINT('Ctrl Pts',(38.4781801929734,36.5380966439885,11.0622545443404));
#27142=CARTESIAN_POINT('Origin',(0.,0.,11.5));
#27143=CARTESIAN_POINT('Origin',(0.,0.,11.25));
#27144=CARTESIAN_POINT('Origin',(0.,0.,11.5));
#27145=CARTESIAN_POINT('Origin',(0.,0.,11.25));
#27146=CARTESIAN_POINT('Origin',(0.,0.,11.5));
#27147=CARTESIAN_POINT('Origin',(0.,0.,11.25));
#27148=CARTESIAN_POINT('Origin',(0.,0.,11.5));
#27149=CARTESIAN_POINT('Origin',(0.,0.,11.25));
#27150=CARTESIAN_POINT('Origin',(0.,0.,11.5));
#27151=CARTESIAN_POINT('Origin',(0.,0.,11.25));
#27152=CARTESIAN_POINT('Origin',(0.,0.,11.5));
#27153=CARTESIAN_POINT('Origin',(0.,0.,11.25));
#27154=CARTESIAN_POINT('Origin',(0.,0.,11.5));
#27155=CARTESIAN_POINT('Origin',(0.,0.,14.5));
#27156=CARTESIAN_POINT('Origin',(0.,0.,24.2));
#27157=CARTESIAN_POINT('Origin',(0.,0.,14.5));
#27158=CARTESIAN_POINT('Origin',(0.,0.,24.2));
#27159=CARTESIAN_POINT('Origin',(0.,0.,14.5));
#27160=CARTESIAN_POINT('Origin',(0.,0.,24.2));
#27161=CARTESIAN_POINT('Origin',(0.,0.,14.5));
#27162=CARTESIAN_POINT('Origin',(0.,0.,24.2));
#27163=CARTESIAN_POINT('Origin',(0.,0.,14.5));
#27164=CARTESIAN_POINT('Origin',(0.,0.,24.2));
#27165=CARTESIAN_POINT('Origin',(0.,0.,14.5));
#27166=CARTESIAN_POINT('Origin',(0.,0.,24.2));
#27167=CARTESIAN_POINT('Origin',(0.,0.,14.5));
#27168=CARTESIAN_POINT('Origin',(0.,0.,24.2));
#27169=CARTESIAN_POINT('Origin',(37.7528714186305,37.5960434680237,14.5));
#27170=CARTESIAN_POINT('',(37.8587077455022,37.1795791419031,24.2));
#27171=CARTESIAN_POINT('',(37.8205002822982,37.3299249247391,24.2));
#27172=CARTESIAN_POINT('',(37.8587077455022,37.1795791419031,14.5));
#27173=CARTESIAN_POINT('Origin',(35.8654005008348,39.8325626455883,11.25));
#27174=CARTESIAN_POINT('Origin',(35.8654005008348,39.8325626455883,11.5));
#27175=CARTESIAN_POINT('Origin',(38.5566132981517,37.2336886566023,11.));
#27176=CARTESIAN_POINT('Origin',(38.5566132981517,37.2336886566023,24.2));
#27177=CARTESIAN_POINT('Origin',(35.8654005008348,39.8325626455883,11.));
#27178=CARTESIAN_POINT('Origin',(35.8654005008348,39.8325626455883,24.2));
#27179=CARTESIAN_POINT('Origin',(4.75410644754494,53.0673181599239,14.5));
#27180=CARTESIAN_POINT('',(4.72678212511286,53.0869825079594,11.2969997378715));
#27181=CARTESIAN_POINT('',(4.4053330087579,53.318318063138,11.5));
#27182=CARTESIAN_POINT('Ctrl Pts',(4.72678212511286,53.0869825079594,11.2969997378715));
#27183=CARTESIAN_POINT('Ctrl Pts',(4.56636307296556,53.2024304236685,11.3977655520829));
#27184=CARTESIAN_POINT('Ctrl Pts',(4.4053330087579,53.318318063138,11.5));
#27185=CARTESIAN_POINT('',(4.4053330087579,53.318318063138,24.2));
#27186=CARTESIAN_POINT('',(4.40533300875789,53.318318063138,14.5));
#27187=CARTESIAN_POINT('',(5.102879886332,52.8163182567097,24.2));
#27188=CARTESIAN_POINT('',(4.97697086508332,52.9069305242525,24.2));
#27189=CARTESIAN_POINT('',(5.102879886332,52.8163182567097,11.5));
#27190=CARTESIAN_POINT('',(5.10287988633199,52.8163182567097,14.5));
#27191=CARTESIAN_POINT('Ctrl Pts',(5.102879886332,52.8163182567097,11.5));
#27192=CARTESIAN_POINT('Ctrl Pts',(4.93864508296158,52.9345122335611,11.4654707447275));
#27193=CARTESIAN_POINT('Ctrl Pts',(4.72678212511286,53.0869825079594,11.2969997378715));
#27194=CARTESIAN_POINT('Origin',(5.60272563114623,53.3063735917395,11.25));
#27195=CARTESIAN_POINT('',(5.98976031387286,52.7231033676009,11.5));
#27196=CARTESIAN_POINT('Origin',(5.60272563114623,53.3063735917395,11.5));
#27197=CARTESIAN_POINT('',(6.413913698772,52.9096578341174,11.2969997378715));
#27198=CARTESIAN_POINT('Ctrl Pts',(6.413913698772,52.9096578341174,11.2969997378715));
#27199=CARTESIAN_POINT('Ctrl Pts',(6.17498010231834,52.8045681868194,11.4654707447277));
#27200=CARTESIAN_POINT('Ctrl Pts',(5.98976031387286,52.7231033676009,11.5));
#27201=CARTESIAN_POINT('Ctrl Pts',(6.413913698772,52.9096578341174,11.2969997378716));
#27202=CARTESIAN_POINT('Ctrl Pts',(6.47148112666752,52.8036912002343,11.1987310576087));
#27203=CARTESIAN_POINT('Ctrl Pts',(6.5223713301853,52.6951054327476,11.0971961933879));
#27204=CARTESIAN_POINT('Ctrl Pts',(6.56664309356487,52.5916266955277,11.));
#27205=CARTESIAN_POINT('Ctrl Pts',(4.72678212511286,53.0869825079594,11.2969997378714));
#27206=CARTESIAN_POINT('Ctrl Pts',(4.64844098161554,52.9953004405385,11.1987310576086));
#27207=CARTESIAN_POINT('Ctrl Pts',(4.57608660062689,52.899668200857,11.0971961933879));
#27208=CARTESIAN_POINT('Ctrl Pts',(4.51126784227787,52.8076553394982,11.));
#27209=CARTESIAN_POINT('Origin',(5.60272563114623,53.3063735917395,11.));
#27210=CARTESIAN_POINT('',(5.98976031387286,52.7231033676009,24.2));
#27211=CARTESIAN_POINT('Origin',(5.60272563114623,53.3063735917395,24.2));
#27212=CARTESIAN_POINT('',(5.98976031387286,52.7231033676009,14.5));
#27213=CARTESIAN_POINT('Origin',(6.38309803049426,52.8961042453437,14.5));
#27214=CARTESIAN_POINT('',(6.77643574711566,53.0691051230866,24.2));
#27215=CARTESIAN_POINT('',(6.13175727067173,52.785557582198,24.2));
#27216=CARTESIAN_POINT('',(6.77643574711566,53.0691051230866,11.5));
#27217=CARTESIAN_POINT('',(6.77643574711566,53.0691051230866,14.5));
#27218=CARTESIAN_POINT('Ctrl Pts',(6.77643574711566,53.0691051230866,11.5));
#27219=CARTESIAN_POINT('Ctrl Pts',(6.59483018109884,52.989229939507,11.3977655520833));
#27220=CARTESIAN_POINT('Ctrl Pts',(6.413913698772,52.9096578341174,11.2969997378715));
#27221=CARTESIAN_POINT('Origin',(8.44431466907315,52.6064191384554,14.5));
#27222=CARTESIAN_POINT('',(8.41842862289464,52.6279416335077,11.2969997378715));
#27223=CARTESIAN_POINT('',(8.11389969301204,52.8811368237459,11.5));
#27224=CARTESIAN_POINT('Ctrl Pts',(8.41842862289464,52.6279416335077,11.2969997378715));
#27225=CARTESIAN_POINT('Ctrl Pts',(8.26645358299653,52.7542985912959,11.397765552083));
#27226=CARTESIAN_POINT('Ctrl Pts',(8.11389969301204,52.8811368237459,11.5));
#27227=CARTESIAN_POINT('',(8.11389969301204,52.8811368237459,24.2));
#27228=CARTESIAN_POINT('',(8.11389969301204,52.8811368237459,14.5));
#27229=CARTESIAN_POINT('',(8.77472964513427,52.3317014531649,24.2));
#27230=CARTESIAN_POINT('',(8.65544812419494,52.430875963113,24.2));
#27231=CARTESIAN_POINT('',(8.77472964513427,52.3317014531649,11.5));
#27232=CARTESIAN_POINT('',(8.77472964513427,52.3317014531649,14.5));
#27233=CARTESIAN_POINT('Ctrl Pts',(8.77472964513427,52.3317014531649,11.5));
#27234=CARTESIAN_POINT('Ctrl Pts',(8.6191397045334,52.4610639561783,11.4654707447276));
#27235=CARTESIAN_POINT('Ctrl Pts',(8.41842862289464,52.6279416335077,11.2969997378715));
#27236=CARTESIAN_POINT('Origin',(9.30754232294747,52.7856955614544,11.25));
#27237=CARTESIAN_POINT('',(9.65294733456355,52.1768479795831,11.5));
#27238=CARTESIAN_POINT('Origin',(9.30754232294747,52.7856955614544,11.5));
#27239=CARTESIAN_POINT('',(10.0890808848803,52.3333605643381,11.2969997378715));
#27240=CARTESIAN_POINT('Ctrl Pts',(10.0890808848803,52.3333605643381,11.2969997378715));
#27241=CARTESIAN_POINT('Ctrl Pts',(9.84339863543633,52.2451940752868,11.4654707447276));
#27242=CARTESIAN_POINT('Ctrl Pts',(9.65294733456355,52.1768479795831,11.5));
#27243=CARTESIAN_POINT('Ctrl Pts',(10.0890808848803,52.3333605643381,11.2969997378715));
#27244=CARTESIAN_POINT('Ctrl Pts',(10.1391162227005,52.2236363590767,11.1987310576086));
#27245=CARTESIAN_POINT('Ctrl Pts',(10.1823079000016,52.1117651799167,11.0971961933879));
#27246=CARTESIAN_POINT('Ctrl Pts',(10.2192535077747,52.0054502696,11.));
#27247=CARTESIAN_POINT('Ctrl Pts',(8.41842862289465,52.6279416335078,11.2969997378715));
#27248=CARTESIAN_POINT('Ctrl Pts',(8.33388289675663,52.5419477009147,11.1987310576086));
#27249=CARTESIAN_POINT('Ctrl Pts',(8.25503379958712,52.4515956030403,11.0971961933879));
#27250=CARTESIAN_POINT('Ctrl Pts',(8.18395444372813,52.3643284084021,11.));
#27251=CARTESIAN_POINT('Origin',(9.30754232294747,52.7856955614544,11.));
#27252=CARTESIAN_POINT('',(9.65294733456355,52.1768479795831,24.2));
#27253=CARTESIAN_POINT('Origin',(9.30754232294747,52.7856955614544,24.2));
#27254=CARTESIAN_POINT('',(9.65294733456355,52.1768479795831,14.5));
#27255=CARTESIAN_POINT('Origin',(10.0573948314625,52.3219895837806,14.5));
#27256=CARTESIAN_POINT('',(10.4618423283614,52.4671311879781,24.2));
#27257=CARTESIAN_POINT('',(9.79895497969307,52.2292448518636,24.2));
#27258=CARTESIAN_POINT('',(10.4618423283614,52.4671311879781,11.5));
#27259=CARTESIAN_POINT('',(10.4618423283614,52.4671311879781,14.5));
#27260=CARTESIAN_POINT('Ctrl Pts',(10.4618423283614,52.4671311879781,11.5));
#27261=CARTESIAN_POINT('Ctrl Pts',(10.2751073332288,52.4001187402286,11.3977655520829));
#27262=CARTESIAN_POINT('Ctrl Pts',(10.0890808848803,52.3333605643381,11.2969997378715));
#27263=CARTESIAN_POINT('Origin',(12.0933830383533,51.8892269309231,14.5));
#27264=CARTESIAN_POINT('',(12.0690613826432,51.9125027175599,11.2969997378715));
#27265=CARTESIAN_POINT('',(11.7829362735685,52.1863240013418,11.5));
#27266=CARTESIAN_POINT('Ctrl Pts',(12.0690613826432,51.9125027175599,11.2969997378715));
#27267=CARTESIAN_POINT('Ctrl Pts',(11.926270762113,52.0491531190295,11.3977655520827));
#27268=CARTESIAN_POINT('Ctrl Pts',(11.7829362735685,52.1863240013418,11.5));
#27269=CARTESIAN_POINT('',(11.7829362735685,52.1863240013418,24.2));
#27270=CARTESIAN_POINT('',(11.7829362735685,52.1863240013418,14.5));
#27271=CARTESIAN_POINT('',(12.4038298031382,51.5921298605044,24.2));
#27272=CARTESIAN_POINT('',(12.2917569100881,51.6993834446145,24.2));
#27273=CARTESIAN_POINT('',(12.4038298031382,51.5921298605044,11.5));
#27274=CARTESIAN_POINT('',(12.4038298031382,51.5921298605044,14.5));
#27275=CARTESIAN_POINT('Ctrl Pts',(12.4038298031382,51.5921298605044,11.5));
#27276=CARTESIAN_POINT('Ctrl Pts',(12.2576427438577,51.7320306485686,11.4654707447276));
#27277=CARTESIAN_POINT('Ctrl Pts',(12.0690613826432,51.9125027175599,11.2969997378715));
#27278=CARTESIAN_POINT('Origin',(12.9670136041422,52.0078509283934,11.25));
#27279=CARTESIAN_POINT('',(13.2691061661509,51.3763922330071,11.5));
#27280=CARTESIAN_POINT('Origin',(12.9670136041422,52.0078509283934,11.5));
#27281=CARTESIAN_POINT('',(13.7150950830682,51.5021004224204,11.2969997378715));
#27282=CARTESIAN_POINT('Ctrl Pts',(13.7150950830682,51.5021004224204,11.2969997378715));
#27283=CARTESIAN_POINT('Ctrl Pts',(13.4638611198573,51.4312866298879,11.4654707447276));
#27284=CARTESIAN_POINT('Ctrl Pts',(13.2691061661509,51.3763922330071,11.5));
#27285=CARTESIAN_POINT('Ctrl Pts',(13.7150950830682,51.5021004224204,11.2969997378715));
#27286=CARTESIAN_POINT('Ctrl Pts',(13.7573545636769,51.3891532110793,11.1987310576087));
#27287=CARTESIAN_POINT('Ctrl Pts',(13.7926372892511,51.2745416453855,11.0971961933879));
#27288=CARTESIAN_POINT('Ctrl Pts',(13.8220767461304,51.1659085175284,11.));
#27289=CARTESIAN_POINT('Ctrl Pts',(12.0690613826432,51.9125027175599,11.2969997378715));
#27290=CARTESIAN_POINT('Ctrl Pts',(11.9787229721437,51.8326158735901,11.1987310576087));
#27291=CARTESIAN_POINT('Ctrl Pts',(11.8937633036688,51.7479841038615,11.0971961933879));
#27292=CARTESIAN_POINT('Ctrl Pts',(11.8167696417768,51.6658877329441,11.));
#27293=CARTESIAN_POINT('Origin',(12.9670136041422,52.0078509283934,11.));
#27294=CARTESIAN_POINT('',(13.2691061661509,51.3763922330071,24.2));
#27295=CARTESIAN_POINT('Origin',(12.9670136041422,52.0078509283934,24.2));
#27296=CARTESIAN_POINT('',(13.2691061661509,51.3763922330071,14.5));
#27297=CARTESIAN_POINT('Origin',(13.6826930157771,51.4929674483533,14.5));
#27298=CARTESIAN_POINT('',(14.0962798654034,51.6095426636995,24.2));
#27299=CARTESIAN_POINT('',(13.4184131650408,51.4184764906763,24.2));
#27300=CARTESIAN_POINT('',(14.0962798654034,51.6095426636995,11.5));
#27301=CARTESIAN_POINT('',(14.0962798654034,51.6095426636995,14.5));
#27302=CARTESIAN_POINT('Ctrl Pts',(14.0962798654034,51.6095426636995,11.5));
#27303=CARTESIAN_POINT('Ctrl Pts',(13.9053251952812,51.5557194296896,11.3977655520826));
#27304=CARTESIAN_POINT('Ctrl Pts',(13.7150950830682,51.5021004224204,11.2969997378715));
#27305=CARTESIAN_POINT('Origin',(15.683533661093,50.9192356256704,14.5));
#27306=CARTESIAN_POINT('',(15.6608948885132,50.9441513065986,11.2969997378715));
#27307=CARTESIAN_POINT('',(15.3945675730161,51.2372646541542,11.5));
#27308=CARTESIAN_POINT('Ctrl Pts',(15.6608948885132,50.9441513065986,11.2969997378715));
#27309=CARTESIAN_POINT('Ctrl Pts',(15.5279843488991,51.0904294047314,11.3977655520835));
#27310=CARTESIAN_POINT('Ctrl Pts',(15.3945675730161,51.2372646541542,11.5));
#27311=CARTESIAN_POINT('',(15.3945675730161,51.2372646541542,24.2));
#27312=CARTESIAN_POINT('',(15.3945675730161,51.2372646541542,14.5));
#27313=CARTESIAN_POINT('',(15.9724997491698,50.6012065971865,24.2));
#27314=CARTESIAN_POINT('',(15.8681814918784,50.7160167267776,24.2));
#27315=CARTESIAN_POINT('',(15.9724997491698,50.6012065971865,11.5));
#27316=CARTESIAN_POINT('',(15.9724997491698,50.6012065971865,14.5));
#27317=CARTESIAN_POINT('Ctrl Pts',(15.9724997491698,50.6012065971865,11.5));
#27318=CARTESIAN_POINT('Ctrl Pts',(15.8364277798677,50.7509640877247,11.4654707447276));
#27319=CARTESIAN_POINT('Ctrl Pts',(15.6608948885132,50.9441513065986,11.2969997378715));
#27320=CARTESIAN_POINT('Origin',(16.5633108984972,50.9766292734202,11.25));
#27321=CARTESIAN_POINT('',(16.8206192463028,50.3256358678088,11.5));
#27322=CARTESIAN_POINT('Origin',(16.5633108984972,50.9766292734202,11.5));
#27323=CARTESIAN_POINT('',(17.274290716648,50.4199272242176,11.2969997378715));
#27324=CARTESIAN_POINT('Ctrl Pts',(17.274290716648,50.4199272242176,11.2969997378715));
#27325=CARTESIAN_POINT('Ctrl Pts',(17.018729026285,50.366811125883,11.4654707447276));
#27326=CARTESIAN_POINT('Ctrl Pts',(16.8206192463028,50.3256358678088,11.5));
#27327=CARTESIAN_POINT('Ctrl Pts',(17.274290716648,50.4199272242176,11.2969997378715));
#27328=CARTESIAN_POINT('Ctrl Pts',(17.3085684561035,50.3043072742572,11.1987310576086));
#27329=CARTESIAN_POINT('Ctrl Pts',(17.3357703360584,50.1875136980568,11.0971961933879));
#27330=CARTESIAN_POINT('Ctrl Pts',(17.3575602159692,50.0770916023385,11.));
#27331=CARTESIAN_POINT('Ctrl Pts',(15.6608948885132,50.9441513065986,11.2969997378715));
#27332=CARTESIAN_POINT('Ctrl Pts',(15.5652039133075,50.8707607519257,11.1987310576086));
#27333=CARTESIAN_POINT('Ctrl Pts',(15.474547588492,50.7922616278179,11.0971961933879));
#27334=CARTESIAN_POINT('Ctrl Pts',(15.3920147259482,50.7157360458881,11.));
#27335=CARTESIAN_POINT('Origin',(16.5633108984972,50.9766292734202,11.));
#27336=CARTESIAN_POINT('',(16.8206192463028,50.3256358678088,24.2));
#27337=CARTESIAN_POINT('Origin',(16.5633108984972,50.9766292734202,24.2));
#27338=CARTESIAN_POINT('',(16.8206192463028,50.3256358678088,14.5));
#27339=CARTESIAN_POINT('Origin',(17.2413304950988,50.4130767515726,14.5));
#27340=CARTESIAN_POINT('',(17.6620417438948,50.5005176353364,24.2));
#27341=CARTESIAN_POINT('',(16.9724981902626,50.3572024805936,24.2));
#27342=CARTESIAN_POINT('',(17.6620417438948,50.5005176353364,11.5));
#27343=CARTESIAN_POINT('',(17.6620417438948,50.5005176353364,14.5));
#27344=CARTESIAN_POINT('Ctrl Pts',(17.6620417438948,50.5005176353364,11.5));
#27345=CARTESIAN_POINT('Ctrl Pts',(17.4677977107416,50.4601458364521,11.3977655520826));
#27346=CARTESIAN_POINT('Ctrl Pts',(17.274290716648,50.4199272242176,11.2969997378715));
#27347=CARTESIAN_POINT('Origin',(19.1972756843392,49.7011709228329,14.5));
#27348=CARTESIAN_POINT('',(19.1764300887141,49.7276051113597,11.2969997378715));
#27349=CARTESIAN_POINT('',(18.9311980867048,50.0385825039234,11.5));
#27350=CARTESIAN_POINT('Ctrl Pts',(19.1764300887141,49.7276051113597,11.2969997378715));
#27351=CARTESIAN_POINT('Ctrl Pts',(19.0540471568071,49.8827982539631,11.3977655520827));
#27352=CARTESIAN_POINT('Ctrl Pts',(18.9311980867048,50.0385825039234,11.5));
#27353=CARTESIAN_POINT('',(18.9311980867048,50.0385825039234,24.2));
#27354=CARTESIAN_POINT('',(18.9311980867048,50.0385825039234,14.5));
#27355=CARTESIAN_POINT('',(19.4633532819736,49.3637593417425,24.2));
#27356=CARTESIAN_POINT('',(19.3672978885042,49.485566673404,24.2));
#27357=CARTESIAN_POINT('',(19.4633532819736,49.3637593417425,11.5));
#27358=CARTESIAN_POINT('',(19.4633532819736,49.3637593417425,14.5));
#27359=CARTESIAN_POINT('Ctrl Pts',(19.4633532819736,49.3637593417425,11.5));
#27360=CARTESIAN_POINT('Ctrl Pts',(19.3380593316065,49.5226439313145,11.4654707447276));
#27361=CARTESIAN_POINT('Ctrl Pts',(19.1764300887141,49.7276051113597,11.2969997378715));
#27362=CARTESIAN_POINT('Origin',(20.0789134070929,49.6970546047798,11.25));
#27363=CARTESIAN_POINT('',(20.2901839602894,49.0296980633778,11.5));
#27364=CARTESIAN_POINT('Origin',(20.0789134070929,49.6970546047798,11.5));
#27365=CARTESIAN_POINT('',(20.7493277422619,49.0921132087718,11.2969997378715));
#27366=CARTESIAN_POINT('Ctrl Pts',(20.7493277422619,49.0921132087718,11.2969997378715));
#27367=CARTESIAN_POINT('Ctrl Pts',(20.4906833956133,49.056953580927,11.4654707447276));
#27368=CARTESIAN_POINT('Ctrl Pts',(20.2901839602894,49.0296980633778,11.5));
#27369=CARTESIAN_POINT('Ctrl Pts',(20.7493277422619,49.0921132087718,11.2969997378715));
#27370=CARTESIAN_POINT('Ctrl Pts',(20.7754567428632,48.9743838089661,11.1987310576086));
#27371=CARTESIAN_POINT('Ctrl Pts',(20.7944452523739,48.8559772288225,11.0971961933879));
#27372=CARTESIAN_POINT('Ctrl Pts',(20.8084793972118,48.7443041305937,11.));
#27373=CARTESIAN_POINT('Ctrl Pts',(19.1764300887141,49.7276051113597,11.2969997378715));
#27374=CARTESIAN_POINT('Ctrl Pts',(19.0758527456144,49.6610683973889,11.1987310576086));
#27375=CARTESIAN_POINT('Ctrl Pts',(18.9799414329601,49.5890843587438,11.0971961933879));
#27376=CARTESIAN_POINT('Ctrl Pts',(18.8922714615747,49.5185023907445,11.));
#27377=CARTESIAN_POINT('Origin',(20.0789134070929,49.6970546047798,11.));
#27378=CARTESIAN_POINT('',(20.2901839602894,49.0296980633778,24.2));
#27379=CARTESIAN_POINT('Origin',(20.0789134070929,49.6970546047798,24.2));
#27380=CARTESIAN_POINT('',(20.2901839602894,49.0296980633778,14.5));
#27381=CARTESIAN_POINT('Origin',(20.7159699453406,49.087578612363,14.5));
#27382=CARTESIAN_POINT('',(21.1417559303918,49.1454591613482,24.2));
#27383=CARTESIAN_POINT('',(20.4438949103711,49.0505932419138,24.2));
#27384=CARTESIAN_POINT('',(21.1417559303918,49.1454591613482,11.5));
#27385=CARTESIAN_POINT('',(21.1417559303918,49.1454591613482,14.5));
#27386=CARTESIAN_POINT('Ctrl Pts',(21.1417559303918,49.1454591613482,11.5));
#27387=CARTESIAN_POINT('Ctrl Pts',(20.9451688716126,49.1187354849356,11.397765552083));
#27388=CARTESIAN_POINT('Ctrl Pts',(20.7493277422619,49.0921132087718,11.2969997378715));
#27389=CARTESIAN_POINT('Origin',(22.6174905101547,48.2409671112037,14.5));
#27390=CARTESIAN_POINT('',(22.5985396491308,48.2687910226197,11.2969997378715));
#27391=CARTESIAN_POINT('',(22.3755977062724,48.5961174095941,11.5));
#27392=CARTESIAN_POINT('Ctrl Pts',(22.5985396491308,48.2687910226197,11.2969997378715));
#27393=CARTESIAN_POINT('Ctrl Pts',(22.4872805622718,48.4321431243046,11.3977655520831));
#27394=CARTESIAN_POINT('Ctrl Pts',(22.3755977062724,48.5961174095941,11.5));
#27395=CARTESIAN_POINT('',(22.3755977062724,48.5961174095941,24.2));
#27396=CARTESIAN_POINT('',(22.3755977062724,48.5961174095941,14.5));
#27397=CARTESIAN_POINT('',(22.859383314037,47.8858168128132,24.2));
#27398=CARTESIAN_POINT('',(22.7720587566113,48.0140279134694,24.2));
#27399=CARTESIAN_POINT('',(22.859383314037,47.8858168128132,11.5));
#27400=CARTESIAN_POINT('',(22.859383314037,47.8858168128132,14.5));
#27401=CARTESIAN_POINT('Ctrl Pts',(22.859383314037,47.8858168128132,11.5));
#27402=CARTESIAN_POINT('Ctrl Pts',(22.7454778021365,48.0530544316696,11.4654707447276));
#27403=CARTESIAN_POINT('Ctrl Pts',(22.5985396491308,48.2687910226197,11.2969997378715));
#27404=CARTESIAN_POINT('Origin',(23.4966934678946,48.1753608816354,11.25));
#27405=CARTESIAN_POINT('',(23.6608969375836,47.49489249843,11.5));
#27406=CARTESIAN_POINT('Origin',(23.4966934678946,48.1753608816354,11.5));
#27407=CARTESIAN_POINT('',(24.1232761288306,47.525127352495,11.2969997378715));
#27408=CARTESIAN_POINT('Ctrl Pts',(24.1232761288306,47.525127352495,11.2969997378715));
#27409=CARTESIAN_POINT('Ctrl Pts',(23.8628092151544,47.5080954893125,11.4654707447277));
#27410=CARTESIAN_POINT('Ctrl Pts',(23.6608969375836,47.49489249843,11.5));
#27411=CARTESIAN_POINT('Ctrl Pts',(24.1232761288306,47.525127352495,11.2969997378715));
#27412=CARTESIAN_POINT('Ctrl Pts',(24.1411290927132,47.4058620686457,11.1987310576087));
#27413=CARTESIAN_POINT('Ctrl Pts',(24.1518117216703,47.2864193495151,11.0971961933879));
#27414=CARTESIAN_POINT('Ctrl Pts',(24.1580217584921,47.174039308885,11.));
#27415=CARTESIAN_POINT('Ctrl Pts',(22.5985396491308,48.2687910226197,11.2969997378715));
#27416=CARTESIAN_POINT('Ctrl Pts',(22.4935659408428,48.2094323095332,11.1987310576086));
#27417=CARTESIAN_POINT('Ctrl Pts',(22.3928669106239,48.1443140553513,11.0971961933879));
#27418=CARTESIAN_POINT('Ctrl Pts',(22.300486949685,48.0800195695356,11.));
#27419=CARTESIAN_POINT('Origin',(23.4966934678946,48.1753608816354,11.));
#27420=CARTESIAN_POINT('',(23.6608969375836,47.49489249843,24.2));
#27421=CARTESIAN_POINT('Origin',(23.4966934678946,48.1753608816354,24.2));
#27422=CARTESIAN_POINT('',(23.6608969375836,47.49489249843,14.5));
#27423=CARTESIAN_POINT('Origin',(24.0896832723706,47.5229307244202,14.5));
#27424=CARTESIAN_POINT('',(24.5184696071576,47.5509689504103,24.2));
#27425=CARTESIAN_POINT('',(23.8156910294893,47.5050144435077,24.2));
#27426=CARTESIAN_POINT('',(24.5184696071576,47.5509689504103,11.5));
#27427=CARTESIAN_POINT('',(24.5184696071576,47.5509689504103,14.5));
#27428=CARTESIAN_POINT('Ctrl Pts',(24.5184696071576,47.5509689504103,11.5));
#27429=CARTESIAN_POINT('Ctrl Pts',(24.3204972751397,47.5380235915344,11.3977655520822));
#27430=CARTESIAN_POINT('Ctrl Pts',(24.1232761288306,47.525127352495,11.2969997378715));
#27431=CARTESIAN_POINT('Origin',(25.9275151957071,46.5457381569736,14.5));
#27432=CARTESIAN_POINT('',(25.9105513959743,46.5748162359794,11.2969997378715));
#27433=CARTESIAN_POINT('',(25.7109856630026,46.9168969161098,11.5));
#27434=CARTESIAN_POINT('Ctrl Pts',(25.9105513959743,46.5748162359794,11.2969997378715));
#27435=CARTESIAN_POINT('Ctrl Pts',(25.8109581972508,46.7455314617268,11.3977655520837));
#27436=CARTESIAN_POINT('Ctrl Pts',(25.7109856630026,46.9168969161098,11.5));
#27437=CARTESIAN_POINT('',(25.7109856630026,46.9168969161098,24.2));
#27438=CARTESIAN_POINT('',(25.7109856630026,46.9168969161098,14.5));
#27439=CARTESIAN_POINT('',(26.1440447284116,46.1745793978374,24.2));
#27440=CARTESIAN_POINT('',(26.0658764434955,46.3085696358935,24.2));
#27441=CARTESIAN_POINT('',(26.1440447284116,46.1745793978374,11.5));
#27442=CARTESIAN_POINT('',(26.1440447284116,46.1745793978374,14.5));
#27443=CARTESIAN_POINT('Ctrl Pts',(26.1440447284116,46.1745793978374,11.5));
#27444=CARTESIAN_POINT('Ctrl Pts',(26.0420825911821,46.3493552811098,11.4654707447276));
#27445=CARTESIAN_POINT('Ctrl Pts',(25.9105513959743,46.5748162359794,11.2969997378715));
#27446=CARTESIAN_POINT('Origin',(26.8,46.4189616428459,11.25));
#27447=CARTESIAN_POINT('',(26.9163364033829,45.7286965913998,11.5));
#27448=CARTESIAN_POINT('Origin',(26.8,46.4189616428459,11.5));
#27449=CARTESIAN_POINT('',(27.379698338963,45.7266038529658,11.2969997378715));
#27450=CARTESIAN_POINT('Ctrl Pts',(27.379698338963,45.7266038529658,11.2969997378715));
#27451=CARTESIAN_POINT('Ctrl Pts',(27.1186778268805,45.7277827319711,11.4654707447276));
#27452=CARTESIAN_POINT('Ctrl Pts',(26.9163364033829,45.7286965913998,11.5));
#27453=CARTESIAN_POINT('Ctrl Pts',(27.379698338963,45.7266038529658,11.2969997378715));
#27454=CARTESIAN_POINT('Ctrl Pts',(27.3891882882814,45.6063837335474,11.1987310576087));
#27455=CARTESIAN_POINT('Ctrl Pts',(27.3915129919902,45.4864867883511,11.0971961933879));
#27456=CARTESIAN_POINT('Ctrl Pts',(27.3898686661209,45.3739473095812,11.));
#27457=CARTESIAN_POINT('Ctrl Pts',(25.9105513959743,46.5748162359794,11.2969997378715));
#27458=CARTESIAN_POINT('Ctrl Pts',(25.8016927438527,46.5229247134606,11.1987310576086));
#27459=CARTESIAN_POINT('Ctrl Pts',(25.6966965916221,46.4649894933305,11.0971961933879));
#27460=CARTESIAN_POINT('Ctrl Pts',(25.6000567070134,46.4072957259707,11.));
#27461=CARTESIAN_POINT('Origin',(26.8,46.4189616428459,11.));
#27462=CARTESIAN_POINT('',(26.9163364033829,45.7286965913998,24.2));
#27463=CARTESIAN_POINT('Origin',(26.8,46.4189616428459,24.2));
#27464=CARTESIAN_POINT('',(26.9163364033829,45.7286965913998,14.5));
#27465=CARTESIAN_POINT('Origin',(27.3460340839842,45.7267558949762,14.5));
#27466=CARTESIAN_POINT('',(27.7757317645856,45.7248151985527,24.2));
#27467=CARTESIAN_POINT('',(27.0714594958567,45.7279959899203,24.2));
#27468=CARTESIAN_POINT('',(27.7757317645856,45.7248151985527,11.5));
#27469=CARTESIAN_POINT('',(27.7757317645856,45.7248151985527,14.5));
#27470=CARTESIAN_POINT('Ctrl Pts',(27.7757317645856,45.7248151985527,11.5));
#27471=CARTESIAN_POINT('Ctrl Pts',(27.5773386606331,45.7257112257008,11.3977655520829));
#27472=CARTESIAN_POINT('Ctrl Pts',(27.379698338963,45.7266038529658,11.2969997378715));
#27473=CARTESIAN_POINT('Origin',(29.1112236334504,44.6237430452042,14.5));
#27474=CARTESIAN_POINT('',(29.0963295409359,44.6539336263215,11.2969997378715));
#27475=CARTESIAN_POINT('',(28.9211122820413,45.0091020169205,11.5));
#27476=CARTESIAN_POINT('Ctrl Pts',(29.0963295409359,44.6539336263215,11.2969997378715));
#27477=CARTESIAN_POINT('Ctrl Pts',(29.0088874384024,44.8311802687091,11.3977655520826));
#27478=CARTESIAN_POINT('Ctrl Pts',(28.9211122820413,45.0091020169205,11.5));
#27479=CARTESIAN_POINT('',(28.9211122820413,45.0091020169205,24.2));
#27480=CARTESIAN_POINT('',(28.9211122820413,45.0091020169205,14.5));
#27481=CARTESIAN_POINT('',(29.3013349848595,44.2383840734879,24.2));
#27482=CARTESIAN_POINT('',(29.2327038004797,44.3775006619728,24.2));
#27483=CARTESIAN_POINT('',(29.3013349848595,44.2383840734879,11.5));
#27484=CARTESIAN_POINT('',(29.3013349848595,44.2383840734879,14.5));
#27485=CARTESIAN_POINT('Ctrl Pts',(29.3013349848595,44.2383840734879,11.5));
#27486=CARTESIAN_POINT('Ctrl Pts',(29.2118129715843,44.4198467306414,11.4654707447276));
#27487=CARTESIAN_POINT('Ctrl Pts',(29.0963295409359,44.6539336263215,11.2969997378715));
#27488=CARTESIAN_POINT('Origin',(29.972739626032,44.4364138889502,11.25));
#27489=CARTESIAN_POINT('',(30.0406421838457,43.7397150712088,11.5));
#27490=CARTESIAN_POINT('Origin',(29.972739626032,44.4364138889502,11.5));
#27491=CARTESIAN_POINT('',(30.5027294109855,43.705304935887,11.2969997378715));
#27492=CARTESIAN_POINT('Ctrl Pts',(30.5027294109855,43.705304935887,11.2969997378715));
#27493=CARTESIAN_POINT('Ctrl Pts',(30.242426966194,43.7246888137001,11.4654707447276));
#27494=CARTESIAN_POINT('Ctrl Pts',(30.0406421838457,43.7397150712088,11.5));
#27495=CARTESIAN_POINT('Ctrl Pts',(30.5027294109855,43.705304935887,11.2969997378715));
#27496=CARTESIAN_POINT('Ctrl Pts',(30.5038101116606,43.5847156812369,11.1987310576086));
#27497=CARTESIAN_POINT('Ctrl Pts',(30.4977655643985,43.4649486358398,11.0971961933879));
#27498=CARTESIAN_POINT('Ctrl Pts',(30.4882748868283,43.3527979999583,11.));
#27499=CARTESIAN_POINT('Ctrl Pts',(29.0963295409359,44.6539336263215,11.2969997378715));
#27500=CARTESIAN_POINT('Ctrl Pts',(28.9841162933916,44.609762104652,11.1987310576086));
#27501=CARTESIAN_POINT('Ctrl Pts',(28.8753345498489,44.5592921731428,11.0971961933878));
#27502=CARTESIAN_POINT('Ctrl Pts',(28.774905561374,44.5084802024738,11.));
#27503=CARTESIAN_POINT('Origin',(29.972739626032,44.4364138889502,11.));
#27504=CARTESIAN_POINT('',(30.0406421838457,43.7397150712088,24.2));
#27505=CARTESIAN_POINT('Origin',(29.972739626032,44.4364138889502,24.2));
#27506=CARTESIAN_POINT('',(30.0406421838457,43.7397150712088,14.5));
#27507=CARTESIAN_POINT('Origin',(32.1531051159017,42.4843455428814,14.5));
#27508=CARTESIAN_POINT('',(32.3158720826212,42.086663788759,11.0622545443403));
#27509=CARTESIAN_POINT('',(31.9903381491823,42.8820272970037,11.5));
#27510=CARTESIAN_POINT('Ctrl Pts',(32.3158720826212,42.086663788759,11.0622545443403));
#27511=CARTESIAN_POINT('Ctrl Pts',(32.153773743835,42.4827119120856,11.2776618075211));
#27512=CARTESIAN_POINT('Ctrl Pts',(31.9903381491823,42.8820272970037,11.5));
#27513=CARTESIAN_POINT('',(31.9903381491823,42.8820272970037,24.2));
#27514=CARTESIAN_POINT('',(31.9903381491823,42.8820272970037,14.5));
#27515=CARTESIAN_POINT('',(32.3158720826212,42.0866637887591,24.2));
#27516=CARTESIAN_POINT('',(32.2571123630091,42.2302289656376,24.2));
#27517=CARTESIAN_POINT('',(32.3158720826212,42.0866637887591,14.5));
#27518=CARTESIAN_POINT('Origin',(0.,0.,14.5));
#27519=CARTESIAN_POINT('',(30.8976733488635,43.6758947432898,11.5));
#27520=CARTESIAN_POINT('Origin',(0.,0.,11.5));
#27521=CARTESIAN_POINT('',(30.8976733488635,43.6758947432898,24.2));
#27522=CARTESIAN_POINT('',(30.8976733488635,43.6758947432898,14.5));
#27523=CARTESIAN_POINT('Origin',(0.,0.,24.2));
#27524=CARTESIAN_POINT('Origin',(0.,0.,11.25));
#27525=CARTESIAN_POINT('Ctrl Pts',(32.3467865928173,41.9843470488554,11.));
#27526=CARTESIAN_POINT('Ctrl Pts',(32.3333350107184,42.0190443039229,11.0192759649605));
#27527=CARTESIAN_POINT('Ctrl Pts',(32.3231696871195,42.0535642457408,11.0404458048696));
#27528=CARTESIAN_POINT('Ctrl Pts',(32.3158720826212,42.0866637887589,11.0622545443403));
#27529=CARTESIAN_POINT('Ctrl Pts',(30.8976733488635,43.6758947432898,11.5));
#27530=CARTESIAN_POINT('Ctrl Pts',(30.6998260242344,43.6906277911078,11.3977655520825));
#27531=CARTESIAN_POINT('Ctrl Pts',(30.5027294109855,43.705304935887,11.2969997378715));
#27532=CARTESIAN_POINT('Origin',(30.4691577663546,43.7078049072493,14.5));
#27533=CARTESIAN_POINT('',(30.195338532774,43.728195336432,24.2));
#27534=CARTESIAN_POINT('Origin',(-1.0407366972854,53.2696785416253,14.5));
#27535=CARTESIAN_POINT('',(-0.675303984907617,53.495737816465,24.2));
#27536=CARTESIAN_POINT('',(-1.40616940966319,53.0436192667856,24.2));
#27537=CARTESIAN_POINT('',(-1.27424630420037,53.1252278380639,24.2));
#27538=CARTESIAN_POINT('',(-0.675303984907617,53.495737816465,11.5));
#27539=CARTESIAN_POINT('',(-0.675303984907616,53.495737816465,14.5));
#27540=CARTESIAN_POINT('',(-1.4061694096633,53.0436192667855,11.0622545443403));
#27541=CARTESIAN_POINT('Ctrl Pts',(-0.675303984907617,53.495737816465,11.5));
#27542=CARTESIAN_POINT('Ctrl Pts',(-1.04223785273803,53.268749916186,11.2776618075198));
#27543=CARTESIAN_POINT('Ctrl Pts',(-1.4061694096633,53.0436192667855,11.0622545443403));
#27544=CARTESIAN_POINT('',(-1.40616940966319,53.0436192667856,14.5));
#27545=CARTESIAN_POINT('Origin',(0.,0.,11.25));
#27546=CARTESIAN_POINT('',(0.675303984907623,53.495737816465,11.5));
#27547=CARTESIAN_POINT('Origin',(0.,0.,11.5));
#27548=CARTESIAN_POINT('',(1.4061694096633,53.0436192667855,11.0622545443403));
#27549=CARTESIAN_POINT('Ctrl Pts',(1.4061694096633,53.0436192667855,11.0622545443403));
#27550=CARTESIAN_POINT('Ctrl Pts',(1.04223785273682,53.2687499161868,11.2776618075204));
#27551=CARTESIAN_POINT('Ctrl Pts',(0.675303984907623,53.495737816465,11.5));
#27552=CARTESIAN_POINT('Ctrl Pts',(1.49132004456262,52.9790143785696,11.));
#27553=CARTESIAN_POINT('Ctrl Pts',(1.46004295121972,52.9991784059996,11.0192759649605));
#27554=CARTESIAN_POINT('Ctrl Pts',(1.43152871896432,53.0211305982789,11.0404458048696));
#27555=CARTESIAN_POINT('Ctrl Pts',(1.40616940966333,53.0436192667855,11.0622545443404));
#27556=CARTESIAN_POINT('Ctrl Pts',(-1.40616940966334,53.0436192667855,11.0622545443403));
#27557=CARTESIAN_POINT('Ctrl Pts',(-1.43152871896432,53.0211305982789,11.0404458048696));
#27558=CARTESIAN_POINT('Ctrl Pts',(-1.46004295121971,52.9991784059996,11.0192759649605));
#27559=CARTESIAN_POINT('Ctrl Pts',(-1.49132004456262,52.9790143785696,11.));
#27560=CARTESIAN_POINT('Origin',(0.,0.,14.5));
#27561=CARTESIAN_POINT('',(0.675303984907623,53.495737816465,24.2));
#27562=CARTESIAN_POINT('Origin',(0.,0.,24.2));
#27563=CARTESIAN_POINT('',(0.675303984907623,53.495737816465,14.5));
#27564=CARTESIAN_POINT('Origin',(2.67770341754864,53.2125144041213,14.5));
#27565=CARTESIAN_POINT('',(2.29739178302177,53.0124970957196,11.0622545443404));
#27566=CARTESIAN_POINT('',(2.29739178302177,53.0124970957196,24.2));
#27567=CARTESIAN_POINT('',(2.29739178302177,53.0124970957196,14.5));
#27568=CARTESIAN_POINT('',(3.05801505207551,53.412531712523,24.2));
#27569=CARTESIAN_POINT('',(2.43468625658983,53.0847043819776,24.2));
#27570=CARTESIAN_POINT('',(3.05801505207551,53.412531712523,11.5));
#27571=CARTESIAN_POINT('',(3.0580150520755,53.412531712523,14.5));
#27572=CARTESIAN_POINT('Ctrl Pts',(3.05801505207551,53.412531712523,11.5));
#27573=CARTESIAN_POINT('Ctrl Pts',(2.8050919047221,53.2795118346824,11.352740724576));
#27574=CARTESIAN_POINT('Ctrl Pts',(2.55153997757952,53.14616126267,11.2067970124653));
#27575=CARTESIAN_POINT('Ctrl Pts',(2.29739178302176,53.0124970957196,11.0622545443404));
#27576=CARTESIAN_POINT('Origin',(0.,0.,11.25));
#27577=CARTESIAN_POINT('Ctrl Pts',(2.2079419616008,52.953989389792,11.));
#27578=CARTESIAN_POINT('Ctrl Pts',(2.24054908368457,52.9719223246298,11.0192757561174));
#27579=CARTESIAN_POINT('Ctrl Pts',(2.27052578922379,52.9918323934691,11.0404460254342));
#27580=CARTESIAN_POINT('Ctrl Pts',(2.29739178302177,53.0124970957196,11.0622545443404));
#27581=CARTESIAN_POINT('Origin',(0.,0.,11.5));
#27582=CARTESIAN_POINT('Origin',(0.,0.,11.25));
#27583=CARTESIAN_POINT('Origin',(0.,0.,11.5));
#27584=CARTESIAN_POINT('Origin',(0.,0.,11.25));
#27585=CARTESIAN_POINT('Origin',(0.,0.,11.5));
#27586=CARTESIAN_POINT('Origin',(0.,0.,11.25));
#27587=CARTESIAN_POINT('Origin',(0.,0.,11.5));
#27588=CARTESIAN_POINT('Origin',(0.,0.,11.25));
#27589=CARTESIAN_POINT('Origin',(0.,0.,11.5));
#27590=CARTESIAN_POINT('Origin',(0.,0.,11.25));
#27591=CARTESIAN_POINT('Origin',(0.,0.,11.5));
#27592=CARTESIAN_POINT('Origin',(0.,0.,11.25));
#27593=CARTESIAN_POINT('Origin',(0.,0.,11.5));
#27594=CARTESIAN_POINT('Origin',(0.,0.,11.25));
#27595=CARTESIAN_POINT('Origin',(0.,0.,11.5));
#27596=CARTESIAN_POINT('Origin',(0.,0.,14.5));
#27597=CARTESIAN_POINT('Origin',(0.,0.,24.2));
#27598=CARTESIAN_POINT('Origin',(0.,0.,14.5));
#27599=CARTESIAN_POINT('Origin',(0.,0.,24.2));
#27600=CARTESIAN_POINT('Origin',(0.,0.,14.5));
#27601=CARTESIAN_POINT('Origin',(0.,0.,24.2));
#27602=CARTESIAN_POINT('Origin',(0.,0.,14.5));
#27603=CARTESIAN_POINT('Origin',(0.,0.,24.2));
#27604=CARTESIAN_POINT('Origin',(0.,0.,14.5));
#27605=CARTESIAN_POINT('Origin',(0.,0.,24.2));
#27606=CARTESIAN_POINT('Origin',(0.,0.,14.5));
#27607=CARTESIAN_POINT('Origin',(0.,0.,24.2));
#27608=CARTESIAN_POINT('Origin',(0.,0.,14.5));
#27609=CARTESIAN_POINT('Origin',(0.,0.,24.2));
#27610=CARTESIAN_POINT('Origin',(0.,0.,14.5));
#27611=CARTESIAN_POINT('Origin',(0.,0.,24.2));
#27612=CARTESIAN_POINT('Origin',(1.04073669728541,53.2696785416253,14.5));
#27613=CARTESIAN_POINT('',(1.40616940966319,53.0436192667856,24.2));
#27614=CARTESIAN_POINT('',(1.27424630420038,53.1252278380639,24.2));
#27615=CARTESIAN_POINT('',(1.40616940966319,53.0436192667856,14.5));
#27616=CARTESIAN_POINT('Origin',(1.87061302325406,53.5673483282235,11.));
#27617=CARTESIAN_POINT('Origin',(1.87061302325406,53.5673483282235,24.2));
#27618=CARTESIAN_POINT('Origin',(-35.0383399022473,40.137968579585,14.5));
#27619=CARTESIAN_POINT('',(-34.9037103045182,40.546035650582,24.2));
#27620=CARTESIAN_POINT('',(-35.1729694999764,39.729901508588,24.2));
#27621=CARTESIAN_POINT('',(-35.1243675165795,39.8772158387497,24.2));
#27622=CARTESIAN_POINT('',(-34.9037103045182,40.546035650582,11.5));
#27623=CARTESIAN_POINT('',(-34.9037103045182,40.546035650582,14.5));
#27624=CARTESIAN_POINT('Ctrl Pts',(-34.9037103045182,40.546035650582,11.5));
#27625=CARTESIAN_POINT('Ctrl Pts',(-34.965869317664,40.3576294838967,11.397765552083));
#27626=CARTESIAN_POINT('Ctrl Pts',(-35.027792474811,40.1699382050837,11.2969997378714));
#27627=CARTESIAN_POINT('',(-35.1729694999764,39.729901508588,14.5));
#27628=CARTESIAN_POINT('Origin',(0.,0.,11.25));
#27629=CARTESIAN_POINT('',(-33.8690845744085,41.4141897191236,11.5));
#27630=CARTESIAN_POINT('Origin',(0.,0.,11.5));
#27631=CARTESIAN_POINT('',(-33.4771542514414,41.4710781664026,11.2969997378715));
#27632=CARTESIAN_POINT('Ctrl Pts',(-33.4771542514414,41.4710781664027,11.2969997378715));
#27633=CARTESIAN_POINT('Ctrl Pts',(-33.6727469213818,41.4426880096834,11.3977655520824));
#27634=CARTESIAN_POINT('Ctrl Pts',(-33.8690845744085,41.4141897191236,11.5));
#27635=CARTESIAN_POINT('Ctrl Pts',(-33.4771542514414,41.4710781664027,11.2969997378715));
#27636=CARTESIAN_POINT('Ctrl Pts',(-33.4698204384081,41.3507072752477,11.1987310576087));
#27637=CARTESIAN_POINT('Ctrl Pts',(-33.4554360886017,41.2316536226562,11.0971961933879));
#27638=CARTESIAN_POINT('Ctrl Pts',(-33.4381452969578,41.1204382162877,11.));
#27639=CARTESIAN_POINT('Origin',(0.,0.,14.5));
#27640=CARTESIAN_POINT('',(-33.8690845744085,41.4141897191236,24.2));
#27641=CARTESIAN_POINT('Origin',(0.,0.,24.2));
#27642=CARTESIAN_POINT('',(-33.8690845744085,41.4141897191236,14.5));
#27643=CARTESIAN_POINT('Origin',(-33.443838774836,41.4759138875076,14.5));
#27644=CARTESIAN_POINT('',(-33.0185929752635,41.5376380558916,24.2));
#27645=CARTESIAN_POINT('',(-33.1721089155843,41.5153553108074,24.2));
#27646=CARTESIAN_POINT('',(-33.0185929752635,41.5376380558916,11.5));
#27647=CARTESIAN_POINT('',(-33.0185929752635,41.5376380558916,14.5));
#27648=CARTESIAN_POINT('Ctrl Pts',(-33.0185929752635,41.5376380558916,11.5));
#27649=CARTESIAN_POINT('Ctrl Pts',(-33.2188380412863,41.5085726067192,11.4654707447276));
#27650=CARTESIAN_POINT('Ctrl Pts',(-33.4771542514414,41.4710781664026,11.2969997378715));
#27651=CARTESIAN_POINT('Origin',(-32.1531051159017,42.4843455428814,14.5));
#27652=CARTESIAN_POINT('',(-31.9903381491823,42.8820272970037,24.2));
#27653=CARTESIAN_POINT('',(-32.3158720826212,42.0866637887591,24.2));
#27654=CARTESIAN_POINT('',(-32.2571123630091,42.2302289656376,24.2));
#27655=CARTESIAN_POINT('',(-31.9903381491823,42.8820272970037,11.5));
#27656=CARTESIAN_POINT('',(-31.9903381491823,42.8820272970037,14.5));
#27657=CARTESIAN_POINT('',(-32.140353293127,42.5155015406339,11.2969997378715));
#27658=CARTESIAN_POINT('Ctrl Pts',(-31.9903381491823,42.8820272970037,11.5));
#27659=CARTESIAN_POINT('Ctrl Pts',(-32.0654882959164,42.6984160718386,11.3977655520826));
#27660=CARTESIAN_POINT('Ctrl Pts',(-32.140353293127,42.5155015406339,11.2969997378715));
#27661=CARTESIAN_POINT('',(-32.3158720826212,42.0866637887591,11.5));
#27662=CARTESIAN_POINT('Ctrl Pts',(-32.140353293127,42.5155015406339,11.2969997378715));
#27663=CARTESIAN_POINT('Ctrl Pts',(-32.2392263355501,42.2739291519686,11.4654707447276));
#27664=CARTESIAN_POINT('Ctrl Pts',(-32.3158720826212,42.0866637887591,11.5));
#27665=CARTESIAN_POINT('',(-32.3158720826212,42.0866637887591,14.5));
#27666=CARTESIAN_POINT('Origin',(0.,0.,11.25));
#27667=CARTESIAN_POINT('',(-30.8976733488635,43.6758947432898,11.5));
#27668=CARTESIAN_POINT('Origin',(0.,0.,11.5));
#27669=CARTESIAN_POINT('',(-30.5027294109855,43.705304935887,11.2969997378715));
#27670=CARTESIAN_POINT('Ctrl Pts',(-30.5027294109855,43.705304935887,11.2969997378715));
#27671=CARTESIAN_POINT('Ctrl Pts',(-30.699826024235,43.6906277911078,11.3977655520827));
#27672=CARTESIAN_POINT('Ctrl Pts',(-30.8976733488635,43.6758947432898,11.5));
#27673=CARTESIAN_POINT('Ctrl Pts',(-30.5027294109855,43.705304935887,11.2969997378715));
#27674=CARTESIAN_POINT('Ctrl Pts',(-30.5038101116606,43.5847156812369,11.1987310576086));
#27675=CARTESIAN_POINT('Ctrl Pts',(-30.4977655643985,43.4649486358399,11.0971961933879));
#27676=CARTESIAN_POINT('Ctrl Pts',(-30.4882748868283,43.3527979999583,11.));
#27677=CARTESIAN_POINT('Ctrl Pts',(-32.140353293127,42.5155015406339,11.2969997378715));
#27678=CARTESIAN_POINT('Ctrl Pts',(-32.0253321418224,42.4792652190273,11.1987310576087));
#27679=CARTESIAN_POINT('Ctrl Pts',(-31.9132947806875,42.4365064605718,11.0971961933879));
#27680=CARTESIAN_POINT('Ctrl Pts',(-31.809565968283,42.3928238374073,11.));
#27681=CARTESIAN_POINT('Origin',(0.,0.,14.5));
#27682=CARTESIAN_POINT('',(-30.8976733488635,43.6758947432898,24.2));
#27683=CARTESIAN_POINT('Origin',(0.,0.,24.2));
#27684=CARTESIAN_POINT('',(-30.8976733488635,43.6758947432898,14.5));
#27685=CARTESIAN_POINT('Origin',(-30.4691577663546,43.7078049072493,14.5));
#27686=CARTESIAN_POINT('',(-30.0406421838457,43.7397150712088,24.2));
#27687=CARTESIAN_POINT('',(-30.195338532774,43.728195336432,24.2));
#27688=CARTESIAN_POINT('',(-30.0406421838457,43.7397150712088,11.5));
#27689=CARTESIAN_POINT('',(-30.0406421838457,43.7397150712088,14.5));
#27690=CARTESIAN_POINT('Ctrl Pts',(-30.0406421838457,43.7397150712088,11.5));
#27691=CARTESIAN_POINT('Ctrl Pts',(-30.242426966194,43.7246888137001,11.4654707447276));
#27692=CARTESIAN_POINT('Ctrl Pts',(-30.5027294109855,43.705304935887,11.2969997378715));
#27693=CARTESIAN_POINT('Origin',(-29.1112236334504,44.6237430452042,14.5));
#27694=CARTESIAN_POINT('',(-28.9211122820413,45.0091020169205,24.2));
#27695=CARTESIAN_POINT('',(-29.3013349848595,44.2383840734879,24.2));
#27696=CARTESIAN_POINT('',(-29.2327038004797,44.3775006619728,24.2));
#27697=CARTESIAN_POINT('',(-28.9211122820413,45.0091020169205,11.5));
#27698=CARTESIAN_POINT('',(-28.9211122820413,45.0091020169205,14.5));
#27699=CARTESIAN_POINT('',(-29.0963295409359,44.6539336263215,11.2969997378715));
#27700=CARTESIAN_POINT('Ctrl Pts',(-28.9211122820413,45.0091020169205,11.5));
#27701=CARTESIAN_POINT('Ctrl Pts',(-29.0088874384022,44.8311802687095,11.3977655520828));
#27702=CARTESIAN_POINT('Ctrl Pts',(-29.0963295409359,44.6539336263215,11.2969997378715));
#27703=CARTESIAN_POINT('',(-29.3013349848595,44.2383840734879,11.5));
#27704=CARTESIAN_POINT('Ctrl Pts',(-29.0963295409359,44.6539336263215,11.2969997378715));
#27705=CARTESIAN_POINT('Ctrl Pts',(-29.2118129715843,44.4198467306414,11.4654707447276));
#27706=CARTESIAN_POINT('Ctrl Pts',(-29.3013349848595,44.2383840734879,11.5));
#27707=CARTESIAN_POINT('',(-29.3013349848595,44.2383840734879,14.5));
#27708=CARTESIAN_POINT('Origin',(0.,0.,11.25));
#27709=CARTESIAN_POINT('',(-27.7757317645856,45.7248151985527,11.5));
#27710=CARTESIAN_POINT('Origin',(0.,0.,11.5));
#27711=CARTESIAN_POINT('',(-27.3796983389629,45.7266038529658,11.2969997378715));
#27712=CARTESIAN_POINT('Ctrl Pts',(-27.3796983389629,45.7266038529658,11.2969997378715));
#27713=CARTESIAN_POINT('Ctrl Pts',(-27.5773386606337,45.7257112257008,11.3977655520832));
#27714=CARTESIAN_POINT('Ctrl Pts',(-27.7757317645856,45.7248151985527,11.5));
#27715=CARTESIAN_POINT('Ctrl Pts',(-27.3796983389629,45.7266038529658,11.2969997378715));
#27716=CARTESIAN_POINT('Ctrl Pts',(-27.3891882882814,45.6063837335474,11.1987310576087));
#27717=CARTESIAN_POINT('Ctrl Pts',(-27.3915129919902,45.4864867883511,11.0971961933879));
#27718=CARTESIAN_POINT('Ctrl Pts',(-27.3898686661209,45.3739473095812,11.));
#27719=CARTESIAN_POINT('Ctrl Pts',(-29.0963295409359,44.6539336263215,11.2969997378715));
#27720=CARTESIAN_POINT('Ctrl Pts',(-28.9841162933917,44.6097621046521,11.1987310576087));
#27721=CARTESIAN_POINT('Ctrl Pts',(-28.875334549849,44.5592921731428,11.0971961933879));
#27722=CARTESIAN_POINT('Ctrl Pts',(-28.774905561374,44.5084802024738,11.));
#27723=CARTESIAN_POINT('Origin',(0.,0.,14.5));
#27724=CARTESIAN_POINT('',(-27.7757317645856,45.7248151985527,24.2));
#27725=CARTESIAN_POINT('Origin',(0.,0.,24.2));
#27726=CARTESIAN_POINT('',(-27.7757317645856,45.7248151985527,14.5));
#27727=CARTESIAN_POINT('Origin',(-27.3460340839842,45.7267558949762,14.5));
#27728=CARTESIAN_POINT('',(-26.9163364033829,45.7286965913998,24.2));
#27729=CARTESIAN_POINT('',(-27.0714594958567,45.7279959899203,24.2));
#27730=CARTESIAN_POINT('',(-26.9163364033829,45.7286965913998,11.5));
#27731=CARTESIAN_POINT('',(-26.9163364033829,45.7286965913998,14.5));
#27732=CARTESIAN_POINT('Ctrl Pts',(-26.9163364033829,45.7286965913998,11.5));
#27733=CARTESIAN_POINT('Ctrl Pts',(-27.1186778268805,45.7277827319711,11.4654707447276));
#27734=CARTESIAN_POINT('Ctrl Pts',(-27.3796983389629,45.7266038529658,11.2969997378715));
#27735=CARTESIAN_POINT('Origin',(-25.927515195707,46.5457381569737,14.5));
#27736=CARTESIAN_POINT('',(-25.7109856630023,46.91689691611,24.2));
#27737=CARTESIAN_POINT('',(-26.1440447284116,46.1745793978375,24.2));
#27738=CARTESIAN_POINT('',(-26.0658764434955,46.3085696358935,24.2));
#27739=CARTESIAN_POINT('',(-25.7109856630023,46.91689691611,11.5));
#27740=CARTESIAN_POINT('',(-25.7109856630023,46.91689691611,14.5));
#27741=CARTESIAN_POINT('',(-25.9105513959742,46.5748162359794,11.2969997378715));
#27742=CARTESIAN_POINT('Ctrl Pts',(-25.7109856630023,46.91689691611,11.5));
#27743=CARTESIAN_POINT('Ctrl Pts',(-25.8109581972516,46.7455314617252,11.3977655520827));
#27744=CARTESIAN_POINT('Ctrl Pts',(-25.9105513959742,46.5748162359794,11.2969997378715));
#27745=CARTESIAN_POINT('',(-26.1440447284116,46.1745793978375,11.5));
#27746=CARTESIAN_POINT('Ctrl Pts',(-25.9105513959742,46.5748162359794,11.2969997378715));
#27747=CARTESIAN_POINT('Ctrl Pts',(-26.042082591182,46.3493552811099,11.4654707447276));
#27748=CARTESIAN_POINT('Ctrl Pts',(-26.1440447284116,46.1745793978375,11.5));
#27749=CARTESIAN_POINT('',(-26.1440447284116,46.1745793978375,14.5));
#27750=CARTESIAN_POINT('Origin',(0.,0.,11.25));
#27751=CARTESIAN_POINT('',(-24.5184696071579,47.5509689504102,11.5));
#27752=CARTESIAN_POINT('Origin',(0.,0.,11.5));
#27753=CARTESIAN_POINT('',(-24.1232761288307,47.5251273524949,11.2969997378715));
#27754=CARTESIAN_POINT('Ctrl Pts',(-24.1232761288307,47.5251273524949,11.2969997378715));
#27755=CARTESIAN_POINT('Ctrl Pts',(-24.3204972751416,47.5380235915344,11.3977655520831));
#27756=CARTESIAN_POINT('Ctrl Pts',(-24.5184696071579,47.5509689504102,11.5));
#27757=CARTESIAN_POINT('Ctrl Pts',(-24.1232761288307,47.5251273524949,11.2969997378715));
#27758=CARTESIAN_POINT('Ctrl Pts',(-24.1411290927132,47.4058620686457,11.1987310576086));
#27759=CARTESIAN_POINT('Ctrl Pts',(-24.1518117216703,47.2864193495151,11.0971961933879));
#27760=CARTESIAN_POINT('Ctrl Pts',(-24.1580217584921,47.174039308885,11.));
#27761=CARTESIAN_POINT('Ctrl Pts',(-25.9105513959742,46.5748162359794,11.2969997378715));
#27762=CARTESIAN_POINT('Ctrl Pts',(-25.8016927438527,46.5229247134606,11.1987310576086));
#27763=CARTESIAN_POINT('Ctrl Pts',(-25.6966965916221,46.4649894933305,11.0971961933879));
#27764=CARTESIAN_POINT('Ctrl Pts',(-25.6000567070134,46.4072957259707,11.));
#27765=CARTESIAN_POINT('Origin',(0.,0.,14.5));
#27766=CARTESIAN_POINT('',(-24.5184696071579,47.5509689504102,24.2));
#27767=CARTESIAN_POINT('Origin',(0.,0.,24.2));
#27768=CARTESIAN_POINT('',(-24.5184696071579,47.5509689504102,14.5));
#27769=CARTESIAN_POINT('Origin',(-24.0896832723708,47.5229307244201,14.5));
#27770=CARTESIAN_POINT('',(-23.6608969375837,47.49489249843,24.2));
#27771=CARTESIAN_POINT('',(-23.8156910294893,47.5050144435077,24.2));
#27772=CARTESIAN_POINT('',(-23.6608969375837,47.49489249843,11.5));
#27773=CARTESIAN_POINT('',(-23.6608969375837,47.49489249843,14.5));
#27774=CARTESIAN_POINT('Ctrl Pts',(-23.6608969375837,47.49489249843,11.5));
#27775=CARTESIAN_POINT('Ctrl Pts',(-23.8628092151544,47.5080954893125,11.4654707447276));
#27776=CARTESIAN_POINT('Ctrl Pts',(-24.1232761288307,47.5251273524949,11.2969997378715));
#27777=CARTESIAN_POINT('Origin',(-22.6174905101547,48.2409671112037,14.5));
#27778=CARTESIAN_POINT('',(-22.3755977062724,48.5961174095941,24.2));
#27779=CARTESIAN_POINT('',(-22.859383314037,47.8858168128132,24.2));
#27780=CARTESIAN_POINT('',(-22.7720587566113,48.0140279134694,24.2));
#27781=CARTESIAN_POINT('',(-22.3755977062724,48.5961174095941,11.5));
#27782=CARTESIAN_POINT('',(-22.3755977062724,48.5961174095941,14.5));
#27783=CARTESIAN_POINT('',(-22.5985396491308,48.2687910226197,11.2969997378715));
#27784=CARTESIAN_POINT('Ctrl Pts',(-22.3755977062724,48.5961174095941,11.5));
#27785=CARTESIAN_POINT('Ctrl Pts',(-22.4872805622725,48.4321431243035,11.3977655520824));
#27786=CARTESIAN_POINT('Ctrl Pts',(-22.5985396491308,48.2687910226197,11.2969997378715));
#27787=CARTESIAN_POINT('',(-22.859383314037,47.8858168128132,11.5));
#27788=CARTESIAN_POINT('Ctrl Pts',(-22.5985396491308,48.2687910226197,11.2969997378715));
#27789=CARTESIAN_POINT('Ctrl Pts',(-22.7454778021365,48.0530544316697,11.4654707447276));
#27790=CARTESIAN_POINT('Ctrl Pts',(-22.859383314037,47.8858168128132,11.5));
#27791=CARTESIAN_POINT('',(-22.859383314037,47.8858168128132,14.5));
#27792=CARTESIAN_POINT('Origin',(0.,0.,11.25));
#27793=CARTESIAN_POINT('',(-21.1417559303918,49.1454591613482,11.5));
#27794=CARTESIAN_POINT('Origin',(0.,0.,11.5));
#27795=CARTESIAN_POINT('',(-20.7493277422619,49.0921132087718,11.2969997378715));
#27796=CARTESIAN_POINT('Ctrl Pts',(-20.7493277422619,49.0921132087718,11.2969997378715));
#27797=CARTESIAN_POINT('Ctrl Pts',(-20.9451688716126,49.1187354849356,11.397765552083));
#27798=CARTESIAN_POINT('Ctrl Pts',(-21.1417559303918,49.1454591613482,11.5));
#27799=CARTESIAN_POINT('Ctrl Pts',(-20.7493277422619,49.0921132087718,11.2969997378715));
#27800=CARTESIAN_POINT('Ctrl Pts',(-20.7754567428632,48.9743838089661,11.1987310576086));
#27801=CARTESIAN_POINT('Ctrl Pts',(-20.7944452523739,48.8559772288225,11.0971961933878));
#27802=CARTESIAN_POINT('Ctrl Pts',(-20.8084793972118,48.7443041305937,11.));
#27803=CARTESIAN_POINT('Ctrl Pts',(-22.5985396491308,48.2687910226197,11.2969997378715));
#27804=CARTESIAN_POINT('Ctrl Pts',(-22.4935659408428,48.2094323095331,11.1987310576086));
#27805=CARTESIAN_POINT('Ctrl Pts',(-22.3928669106238,48.1443140553513,11.0971961933879));
#27806=CARTESIAN_POINT('Ctrl Pts',(-22.300486949685,48.0800195695356,11.));
#27807=CARTESIAN_POINT('Origin',(0.,0.,14.5));
#27808=CARTESIAN_POINT('',(-21.1417559303918,49.1454591613482,24.2));
#27809=CARTESIAN_POINT('Origin',(0.,0.,24.2));
#27810=CARTESIAN_POINT('',(-21.1417559303918,49.1454591613482,14.5));
#27811=CARTESIAN_POINT('Origin',(-20.7159699453406,49.087578612363,14.5));
#27812=CARTESIAN_POINT('',(-20.2901839602894,49.0296980633778,24.2));
#27813=CARTESIAN_POINT('',(-20.4438949103711,49.0505932419138,24.2));
#27814=CARTESIAN_POINT('',(-20.2901839602894,49.0296980633778,11.5));
#27815=CARTESIAN_POINT('',(-20.2901839602894,49.0296980633778,14.5));
#27816=CARTESIAN_POINT('Ctrl Pts',(-20.2901839602894,49.0296980633778,11.5));
#27817=CARTESIAN_POINT('Ctrl Pts',(-20.4906833956133,49.056953580927,11.4654707447276));
#27818=CARTESIAN_POINT('Ctrl Pts',(-20.7493277422619,49.0921132087718,11.2969997378715));
#27819=CARTESIAN_POINT('Origin',(-19.1972756843392,49.7011709228329,14.5));
#27820=CARTESIAN_POINT('',(-18.9311980867048,50.0385825039234,24.2));
#27821=CARTESIAN_POINT('',(-19.4633532819736,49.3637593417425,24.2));
#27822=CARTESIAN_POINT('',(-19.3672978885042,49.485566673404,24.2));
#27823=CARTESIAN_POINT('',(-18.9311980867048,50.0385825039234,11.5));
#27824=CARTESIAN_POINT('',(-18.9311980867048,50.0385825039234,14.5));
#27825=CARTESIAN_POINT('',(-19.1764300887141,49.7276051113597,11.2969997378715));
#27826=CARTESIAN_POINT('Ctrl Pts',(-18.9311980867048,50.0385825039234,11.5));
#27827=CARTESIAN_POINT('Ctrl Pts',(-19.0540471568067,49.8827982539635,11.397765552083));
#27828=CARTESIAN_POINT('Ctrl Pts',(-19.1764300887141,49.7276051113597,11.2969997378715));
#27829=CARTESIAN_POINT('',(-19.4633532819736,49.3637593417425,11.5));
#27830=CARTESIAN_POINT('Ctrl Pts',(-19.1764300887141,49.7276051113597,11.2969997378715));
#27831=CARTESIAN_POINT('Ctrl Pts',(-19.3380593316064,49.5226439313145,11.4654707447276));
#27832=CARTESIAN_POINT('Ctrl Pts',(-19.4633532819736,49.3637593417425,11.5));
#27833=CARTESIAN_POINT('',(-19.4633532819736,49.3637593417425,14.5));
#27834=CARTESIAN_POINT('Origin',(0.,0.,11.25));
#27835=CARTESIAN_POINT('',(-17.6620417438945,50.5005176353365,11.5));
#27836=CARTESIAN_POINT('Origin',(0.,0.,11.5));
#27837=CARTESIAN_POINT('',(-17.274290716648,50.4199272242177,11.2969997378715));
#27838=CARTESIAN_POINT('Ctrl Pts',(-17.274290716648,50.4199272242177,11.2969997378715));
#27839=CARTESIAN_POINT('Ctrl Pts',(-17.4677977107421,50.4601458364523,11.397765552083));
#27840=CARTESIAN_POINT('Ctrl Pts',(-17.6620417438945,50.5005176353365,11.5));
#27841=CARTESIAN_POINT('Ctrl Pts',(-17.274290716648,50.4199272242177,11.2969997378715));
#27842=CARTESIAN_POINT('Ctrl Pts',(-17.3085684561035,50.3043072742572,11.1987310576086));
#27843=CARTESIAN_POINT('Ctrl Pts',(-17.3357703360584,50.1875136980568,11.0971961933879));
#27844=CARTESIAN_POINT('Ctrl Pts',(-17.3575602159693,50.0770916023385,11.));
#27845=CARTESIAN_POINT('Ctrl Pts',(-19.1764300887141,49.7276051113597,11.2969997378715));
#27846=CARTESIAN_POINT('Ctrl Pts',(-19.0758527456144,49.6610683973889,11.1987310576086));
#27847=CARTESIAN_POINT('Ctrl Pts',(-18.9799414329601,49.5890843587438,11.0971961933879));
#27848=CARTESIAN_POINT('Ctrl Pts',(-18.8922714615747,49.5185023907445,11.));
#27849=CARTESIAN_POINT('Origin',(0.,0.,14.5));
#27850=CARTESIAN_POINT('',(-17.6620417438945,50.5005176353365,24.2));
#27851=CARTESIAN_POINT('Origin',(0.,0.,24.2));
#27852=CARTESIAN_POINT('',(-17.6620417438945,50.5005176353365,14.5));
#27853=CARTESIAN_POINT('Origin',(-17.2413304950986,50.4130767515726,14.5));
#27854=CARTESIAN_POINT('',(-16.8206192463027,50.3256358678088,24.2));
#27855=CARTESIAN_POINT('',(-16.9724981902626,50.3572024805937,24.2));
#27856=CARTESIAN_POINT('',(-16.8206192463027,50.3256358678088,11.5));
#27857=CARTESIAN_POINT('',(-16.8206192463027,50.3256358678088,14.5));
#27858=CARTESIAN_POINT('Ctrl Pts',(-16.8206192463027,50.3256358678088,11.5));
#27859=CARTESIAN_POINT('Ctrl Pts',(-17.0187290262849,50.366811125883,11.4654707447276));
#27860=CARTESIAN_POINT('Ctrl Pts',(-17.274290716648,50.4199272242177,11.2969997378715));
#27861=CARTESIAN_POINT('Origin',(-15.683533661093,50.9192356256704,14.5));
#27862=CARTESIAN_POINT('',(-15.3945675730161,51.2372646541542,24.2));
#27863=CARTESIAN_POINT('',(-15.9724997491698,50.6012065971865,24.2));
#27864=CARTESIAN_POINT('',(-15.8681814918784,50.7160167267776,24.2));
#27865=CARTESIAN_POINT('',(-15.3945675730161,51.2372646541542,11.5));
#27866=CARTESIAN_POINT('',(-15.3945675730161,51.2372646541542,14.5));
#27867=CARTESIAN_POINT('',(-15.6608948885132,50.9441513065986,11.2969997378715));
#27868=CARTESIAN_POINT('Ctrl Pts',(-15.3945675730161,51.2372646541542,11.5));
#27869=CARTESIAN_POINT('Ctrl Pts',(-15.5279843488997,51.0904294047306,11.397765552083));
#27870=CARTESIAN_POINT('Ctrl Pts',(-15.6608948885132,50.9441513065986,11.2969997378715));
#27871=CARTESIAN_POINT('',(-15.9724997491698,50.6012065971865,11.5));
#27872=CARTESIAN_POINT('Ctrl Pts',(-15.6608948885132,50.9441513065986,11.2969997378715));
#27873=CARTESIAN_POINT('Ctrl Pts',(-15.8364277798677,50.7509640877247,11.4654707447276));
#27874=CARTESIAN_POINT('Ctrl Pts',(-15.9724997491698,50.6012065971865,11.5));
#27875=CARTESIAN_POINT('',(-15.9724997491698,50.6012065971865,14.5));
#27876=CARTESIAN_POINT('Origin',(0.,0.,11.25));
#27877=CARTESIAN_POINT('',(-14.0962798654037,51.6095426636995,11.5));
#27878=CARTESIAN_POINT('Origin',(0.,0.,11.5));
#27879=CARTESIAN_POINT('',(-13.7150950830682,51.5021004224203,11.2969997378715));
#27880=CARTESIAN_POINT('Ctrl Pts',(-13.7150950830682,51.5021004224203,11.2969997378715));
#27881=CARTESIAN_POINT('Ctrl Pts',(-13.9053251952821,51.5557194296898,11.3977655520829));
#27882=CARTESIAN_POINT('Ctrl Pts',(-14.0962798654037,51.6095426636995,11.5));
#27883=CARTESIAN_POINT('Ctrl Pts',(-13.7150950830682,51.5021004224203,11.2969997378715));
#27884=CARTESIAN_POINT('Ctrl Pts',(-13.7573545636769,51.3891532110793,11.1987310576086));
#27885=CARTESIAN_POINT('Ctrl Pts',(-13.7926372892511,51.2745416453855,11.0971961933879));
#27886=CARTESIAN_POINT('Ctrl Pts',(-13.8220767461304,51.1659085175284,11.));
#27887=CARTESIAN_POINT('Ctrl Pts',(-15.6608948885132,50.9441513065986,11.2969997378715));
#27888=CARTESIAN_POINT('Ctrl Pts',(-15.5652039133075,50.8707607519257,11.1987310576086));
#27889=CARTESIAN_POINT('Ctrl Pts',(-15.474547588492,50.7922616278179,11.0971961933879));
#27890=CARTESIAN_POINT('Ctrl Pts',(-15.3920147259482,50.7157360458881,11.));
#27891=CARTESIAN_POINT('Origin',(0.,0.,14.5));
#27892=CARTESIAN_POINT('',(-14.0962798654037,51.6095426636995,24.2));
#27893=CARTESIAN_POINT('Origin',(0.,0.,24.2));
#27894=CARTESIAN_POINT('',(-14.0962798654037,51.6095426636995,14.5));
#27895=CARTESIAN_POINT('Origin',(-13.6826930157773,51.4929674483533,14.5));
#27896=CARTESIAN_POINT('',(-13.269106166151,51.3763922330071,24.2));
#27897=CARTESIAN_POINT('',(-13.4184131650408,51.4184764906763,24.2));
#27898=CARTESIAN_POINT('',(-13.269106166151,51.3763922330071,11.5));
#27899=CARTESIAN_POINT('',(-13.269106166151,51.3763922330071,14.5));
#27900=CARTESIAN_POINT('Ctrl Pts',(-13.269106166151,51.3763922330071,11.5));
#27901=CARTESIAN_POINT('Ctrl Pts',(-13.4638611198573,51.4312866298879,11.4654707447276));
#27902=CARTESIAN_POINT('Ctrl Pts',(-13.7150950830682,51.5021004224203,11.2969997378715));
#27903=CARTESIAN_POINT('Origin',(-12.0933830383532,51.8892269309232,14.5));
#27904=CARTESIAN_POINT('',(-11.7829362735682,52.1863240013419,24.2));
#27905=CARTESIAN_POINT('',(-12.4038298031382,51.5921298605045,24.2));
#27906=CARTESIAN_POINT('',(-12.2917569100881,51.6993834446145,24.2));
#27907=CARTESIAN_POINT('',(-11.7829362735682,52.1863240013419,11.5));
#27908=CARTESIAN_POINT('',(-11.7829362735682,52.1863240013419,14.5));
#27909=CARTESIAN_POINT('',(-12.0690613826432,51.9125027175599,11.2969997378715));
#27910=CARTESIAN_POINT('Ctrl Pts',(-11.7829362735682,52.1863240013419,11.5));
#27911=CARTESIAN_POINT('Ctrl Pts',(-11.9262707621139,52.0491531190285,11.397765552082));
#27912=CARTESIAN_POINT('Ctrl Pts',(-12.0690613826432,51.9125027175599,11.2969997378715));
#27913=CARTESIAN_POINT('',(-12.4038298031382,51.5921298605045,11.5));
#27914=CARTESIAN_POINT('Ctrl Pts',(-12.0690613826432,51.9125027175599,11.2969997378715));
#27915=CARTESIAN_POINT('Ctrl Pts',(-12.2576427438576,51.7320306485686,11.4654707447276));
#27916=CARTESIAN_POINT('Ctrl Pts',(-12.4038298031382,51.5921298605045,11.5));
#27917=CARTESIAN_POINT('',(-12.4038298031382,51.5921298605045,14.5));
#27918=CARTESIAN_POINT('Origin',(0.,0.,11.25));
#27919=CARTESIAN_POINT('',(-10.4618423283614,52.4671311879781,11.5));
#27920=CARTESIAN_POINT('Origin',(0.,0.,11.5));
#27921=CARTESIAN_POINT('',(-10.0890808848803,52.3333605643381,11.2969997378715));
#27922=CARTESIAN_POINT('Ctrl Pts',(-10.0890808848803,52.3333605643381,11.2969997378715));
#27923=CARTESIAN_POINT('Ctrl Pts',(-10.275107333228,52.4001187402283,11.3977655520824));
#27924=CARTESIAN_POINT('Ctrl Pts',(-10.4618423283614,52.4671311879781,11.5));
#27925=CARTESIAN_POINT('Ctrl Pts',(-10.0890808848803,52.3333605643381,11.2969997378715));
#27926=CARTESIAN_POINT('Ctrl Pts',(-10.1391162227005,52.2236363590767,11.1987310576086));
#27927=CARTESIAN_POINT('Ctrl Pts',(-10.1823079000016,52.1117651799166,11.0971961933879));
#27928=CARTESIAN_POINT('Ctrl Pts',(-10.2192535077747,52.0054502696,11.));
#27929=CARTESIAN_POINT('Ctrl Pts',(-12.0690613826432,51.9125027175599,11.2969997378715));
#27930=CARTESIAN_POINT('Ctrl Pts',(-11.9787229721437,51.8326158735901,11.1987310576086));
#27931=CARTESIAN_POINT('Ctrl Pts',(-11.8937633036688,51.7479841038615,11.0971961933879));
#27932=CARTESIAN_POINT('Ctrl Pts',(-11.8167696417768,51.6658877329441,11.));
#27933=CARTESIAN_POINT('Origin',(0.,0.,14.5));
#27934=CARTESIAN_POINT('',(-10.4618423283614,52.4671311879781,24.2));
#27935=CARTESIAN_POINT('Origin',(0.,0.,24.2));
#27936=CARTESIAN_POINT('',(-10.4618423283614,52.4671311879781,14.5));
#27937=CARTESIAN_POINT('Origin',(-10.0573948314625,52.3219895837806,14.5));
#27938=CARTESIAN_POINT('',(-9.65294733456354,52.1768479795831,24.2));
#27939=CARTESIAN_POINT('',(-9.79895497969307,52.2292448518636,24.2));
#27940=CARTESIAN_POINT('',(-9.65294733456354,52.1768479795831,11.5));
#27941=CARTESIAN_POINT('',(-9.65294733456354,52.1768479795831,14.5));
#27942=CARTESIAN_POINT('Ctrl Pts',(-9.65294733456354,52.1768479795831,11.5));
#27943=CARTESIAN_POINT('Ctrl Pts',(-9.84339863543628,52.2451940752868,11.4654707447276));
#27944=CARTESIAN_POINT('Ctrl Pts',(-10.0890808848803,52.3333605643381,11.2969997378715));
#27945=CARTESIAN_POINT('Origin',(-8.44431466907315,52.6064191384554,14.5));
#27946=CARTESIAN_POINT('',(-8.11389969301203,52.8811368237459,24.2));
#27947=CARTESIAN_POINT('',(-8.77472964513426,52.3317014531649,24.2));
#27948=CARTESIAN_POINT('',(-8.65544812419494,52.430875963113,24.2));
#27949=CARTESIAN_POINT('',(-8.11389969301203,52.8811368237459,11.5));
#27950=CARTESIAN_POINT('',(-8.11389969301203,52.8811368237459,14.5));
#27951=CARTESIAN_POINT('',(-8.41842862289464,52.6279416335077,11.2969997378715));
#27952=CARTESIAN_POINT('Ctrl Pts',(-8.11389969301203,52.8811368237459,11.5));
#27953=CARTESIAN_POINT('Ctrl Pts',(-8.26645358299714,52.7542985912954,11.3977655520826));
#27954=CARTESIAN_POINT('Ctrl Pts',(-8.41842862289464,52.6279416335077,11.2969997378715));
#27955=CARTESIAN_POINT('',(-8.77472964513426,52.3317014531649,11.5));
#27956=CARTESIAN_POINT('Ctrl Pts',(-8.41842862289464,52.6279416335077,11.2969997378715));
#27957=CARTESIAN_POINT('Ctrl Pts',(-8.61913970453336,52.4610639561783,11.4654707447276));
#27958=CARTESIAN_POINT('Ctrl Pts',(-8.77472964513426,52.3317014531649,11.5));
#27959=CARTESIAN_POINT('',(-8.77472964513426,52.3317014531649,14.5));
#27960=CARTESIAN_POINT('Origin',(0.,0.,11.25));
#27961=CARTESIAN_POINT('',(-6.77643574711567,53.0691051230866,11.5));
#27962=CARTESIAN_POINT('Origin',(0.,0.,11.5));
#27963=CARTESIAN_POINT('',(-6.413913698772,52.9096578341174,11.2969997378716));
#27964=CARTESIAN_POINT('Ctrl Pts',(-6.413913698772,52.9096578341174,11.2969997378716));
#27965=CARTESIAN_POINT('Ctrl Pts',(-6.59483018109817,52.9892299395067,11.397765552083));
#27966=CARTESIAN_POINT('Ctrl Pts',(-6.77643574711567,53.0691051230866,11.5));
#27967=CARTESIAN_POINT('Ctrl Pts',(-6.413913698772,52.9096578341174,11.2969997378716));
#27968=CARTESIAN_POINT('Ctrl Pts',(-6.47148112666752,52.8036912002342,11.1987310576087));
#27969=CARTESIAN_POINT('Ctrl Pts',(-6.5223713301853,52.6951054327476,11.0971961933879));
#27970=CARTESIAN_POINT('Ctrl Pts',(-6.56664309356486,52.5916266955276,11.));
#27971=CARTESIAN_POINT('Ctrl Pts',(-8.41842862289464,52.6279416335077,11.2969997378715));
#27972=CARTESIAN_POINT('Ctrl Pts',(-8.33388289675662,52.5419477009146,11.1987310576086));
#27973=CARTESIAN_POINT('Ctrl Pts',(-8.25503379958713,52.4515956030403,11.0971961933879));
#27974=CARTESIAN_POINT('Ctrl Pts',(-8.18395444372814,52.3643284084021,11.));
#27975=CARTESIAN_POINT('Origin',(0.,0.,14.5));
#27976=CARTESIAN_POINT('',(-6.77643574711567,53.0691051230866,24.2));
#27977=CARTESIAN_POINT('Origin',(0.,0.,24.2));
#27978=CARTESIAN_POINT('',(-6.77643574711567,53.0691051230866,14.5));
#27979=CARTESIAN_POINT('Origin',(-4.75410644754495,53.0673181599239,14.5));
#27980=CARTESIAN_POINT('',(-5.102879886332,52.8163182567097,24.2));
#27981=CARTESIAN_POINT('',(-4.97697086508332,52.9069305242525,24.2));
#27982=CARTESIAN_POINT('',(-5.102879886332,52.8163182567097,11.5));
#27983=CARTESIAN_POINT('Ctrl Pts',(-4.72678212511287,53.0869825079594,11.2969997378715));
#27984=CARTESIAN_POINT('Ctrl Pts',(-4.93864508296155,52.9345122335611,11.4654707447276));
#27985=CARTESIAN_POINT('Ctrl Pts',(-5.102879886332,52.8163182567097,11.5));
#27986=CARTESIAN_POINT('',(-5.102879886332,52.8163182567097,14.5));
#27987=CARTESIAN_POINT('Origin',(-5.60272563114623,53.3063735917395,11.));
#27988=CARTESIAN_POINT('',(-5.98976031387287,52.7231033676009,11.5));
#27989=CARTESIAN_POINT('Origin',(-5.60272563114623,53.3063735917395,11.5));
#27990=CARTESIAN_POINT('',(-5.98976031387287,52.7231033676009,24.2));
#27991=CARTESIAN_POINT('',(-5.98976031387287,52.7231033676009,14.5));
#27992=CARTESIAN_POINT('Origin',(-5.60272563114623,53.3063735917395,24.2));
#27993=CARTESIAN_POINT('Origin',(-5.60272563114623,53.3063735917395,11.25));
#27994=CARTESIAN_POINT('Ctrl Pts',(-5.98976031387287,52.7231033676009,11.5));
#27995=CARTESIAN_POINT('Ctrl Pts',(-6.1749801023183,52.8045681868194,11.4654707447276));
#27996=CARTESIAN_POINT('Ctrl Pts',(-6.413913698772,52.9096578341174,11.2969997378716));
#27997=CARTESIAN_POINT('Origin',(-6.38309803049427,52.8961042453437,14.5));
#27998=CARTESIAN_POINT('',(-6.13175727067174,52.785557582198,24.2));
#27999=CARTESIAN_POINT('Origin',(-32.9994550774553,42.2373763933203,11.25));
#28000=CARTESIAN_POINT('Origin',(-32.9994550774553,42.2373763933203,11.5));
#28001=CARTESIAN_POINT('Origin',(-29.972739626032,44.4364138889502,11.25));
#28002=CARTESIAN_POINT('Origin',(-29.972739626032,44.4364138889502,11.5));
#28003=CARTESIAN_POINT('Origin',(-26.8,46.4189616428459,11.25));
#28004=CARTESIAN_POINT('Origin',(-26.8,46.4189616428459,11.5));
#28005=CARTESIAN_POINT('Origin',(-23.4966934678946,48.1753608816354,11.25));
#28006=CARTESIAN_POINT('Origin',(-23.4966934678946,48.1753608816354,11.5));
#28007=CARTESIAN_POINT('Origin',(-20.0789134070929,49.6970546047798,11.25));
#28008=CARTESIAN_POINT('Origin',(-20.0789134070929,49.6970546047798,11.5));
#28009=CARTESIAN_POINT('Origin',(-16.5633108984972,50.9766292734202,11.25));
#28010=CARTESIAN_POINT('Origin',(-16.5633108984972,50.9766292734202,11.5));
#28011=CARTESIAN_POINT('Origin',(-12.9670136041422,52.0078509283934,11.25));
#28012=CARTESIAN_POINT('Origin',(-12.9670136041422,52.0078509283934,11.5));
#28013=CARTESIAN_POINT('Origin',(-9.30754232294747,52.7856955614544,11.25));
#28014=CARTESIAN_POINT('Origin',(-9.30754232294747,52.7856955614544,11.5));
#28015=CARTESIAN_POINT('Origin',(-9.30754232294747,52.7856955614544,11.));
#28016=CARTESIAN_POINT('Origin',(-9.30754232294747,52.7856955614544,24.2));
#28017=CARTESIAN_POINT('Origin',(-12.9670136041422,52.0078509283934,11.));
#28018=CARTESIAN_POINT('Origin',(-12.9670136041422,52.0078509283934,24.2));
#28019=CARTESIAN_POINT('Origin',(-16.5633108984972,50.9766292734202,11.));
#28020=CARTESIAN_POINT('Origin',(-16.5633108984972,50.9766292734202,24.2));
#28021=CARTESIAN_POINT('Origin',(-20.0789134070929,49.6970546047798,11.));
#28022=CARTESIAN_POINT('Origin',(-20.0789134070929,49.6970546047798,24.2));
#28023=CARTESIAN_POINT('Origin',(-23.4966934678946,48.1753608816354,11.));
#28024=CARTESIAN_POINT('Origin',(-23.4966934678946,48.1753608816354,24.2));
#28025=CARTESIAN_POINT('Origin',(-26.8,46.4189616428459,11.));
#28026=CARTESIAN_POINT('Origin',(-26.8,46.4189616428459,24.2));
#28027=CARTESIAN_POINT('Origin',(-29.972739626032,44.4364138889502,11.));
#28028=CARTESIAN_POINT('Origin',(-29.972739626032,44.4364138889502,24.2));
#28029=CARTESIAN_POINT('Origin',(-32.9994550774553,42.2373763933203,11.));
#28030=CARTESIAN_POINT('Origin',(-32.9994550774553,42.2373763933203,24.2));
#28031=CARTESIAN_POINT('Origin',(0.,0.,11.25));
#28032=CARTESIAN_POINT('',(-49.5,-6.0620016557794E-15,11.5));
#28033=CARTESIAN_POINT('Origin',(0.,0.,11.5));
#28034=CARTESIAN_POINT('',(-49.75,-6.09261782575808E-15,11.25));
#28035=CARTESIAN_POINT('Origin',(0.,0.,11.));
#28036=CARTESIAN_POINT('',(-49.5,-6.0620016557794E-15,14.5));
#28037=CARTESIAN_POINT('Origin',(0.,0.,14.5));
#28038=CARTESIAN_POINT('',(-49.5,-6.0620016557794E-15,11.));
#28039=CARTESIAN_POINT('Origin',(-51.9391184236626,11.8772792412203,14.5));
#28040=CARTESIAN_POINT('',(-51.8081802498931,11.4680127538716,24.2));
#28041=CARTESIAN_POINT('',(-51.8081802498931,11.4680127538716,14.5));
#28042=CARTESIAN_POINT('',(-51.8554496100851,11.6157600795601,24.2));
#28043=CARTESIAN_POINT('Origin',(-51.5236269022939,14.7741622717912,11.25));
#28044=CARTESIAN_POINT('Origin',(-51.5236269022939,14.7741622717912,11.5));
#28045=CARTESIAN_POINT('Origin',(-50.3675244741247,18.3322796822559,11.25));
#28046=CARTESIAN_POINT('Origin',(-50.3675244741247,18.3322796822559,11.5));
#28047=CARTESIAN_POINT('Origin',(-48.9660365296434,21.8010840688629,11.25));
#28048=CARTESIAN_POINT('Origin',(-48.9660365296434,21.8010840688629,11.5));
#28049=CARTESIAN_POINT('Origin',(-47.3259909772385,25.1636757653237,11.25));
#28050=CARTESIAN_POINT('Origin',(-47.3259909772385,25.1636757653237,11.5));
#28051=CARTESIAN_POINT('Origin',(-45.4553779539844,28.4036725628998,11.25));
#28052=CARTESIAN_POINT('Origin',(-45.4553779539844,28.4036725628998,11.5));
#28053=CARTESIAN_POINT('Origin',(-43.3633108984972,31.5052895228766,11.25));
#28054=CARTESIAN_POINT('Origin',(-43.3633108984972,31.5052895228766,11.5));
#28055=CARTESIAN_POINT('Origin',(-41.0599821511772,34.4534158791985,11.25));
#28056=CARTESIAN_POINT('Origin',(-41.0599821511772,34.4534158791985,11.5));
#28057=CARTESIAN_POINT('Origin',(-38.5566132981517,37.2336886566023,11.25));
#28058=CARTESIAN_POINT('Origin',(-38.5566132981517,37.2336886566023,11.5));
#28059=CARTESIAN_POINT('Origin',(-35.8654005008348,39.8325626455883,11.));
#28060=CARTESIAN_POINT('Origin',(-35.8654005008348,39.8325626455883,24.2));
#28061=CARTESIAN_POINT('Origin',(-38.5566132981517,37.2336886566023,11.));
#28062=CARTESIAN_POINT('Origin',(-38.5566132981517,37.2336886566023,24.2));
#28063=CARTESIAN_POINT('Origin',(-41.0599821511772,34.4534158791985,11.));
#28064=CARTESIAN_POINT('Origin',(-41.0599821511772,34.4534158791985,24.2));
#28065=CARTESIAN_POINT('Origin',(-43.3633108984972,31.5052895228766,11.));
#28066=CARTESIAN_POINT('Origin',(-43.3633108984972,31.5052895228766,24.2));
#28067=CARTESIAN_POINT('Origin',(-45.4553779539844,28.4036725628998,11.));
#28068=CARTESIAN_POINT('Origin',(-45.4553779539844,28.4036725628998,24.2));
#28069=CARTESIAN_POINT('Origin',(-47.3259909772385,25.1636757653237,11.));
#28070=CARTESIAN_POINT('Origin',(-47.3259909772385,25.1636757653237,24.2));
#28071=CARTESIAN_POINT('Origin',(-48.9660365296434,21.8010840688629,11.));
#28072=CARTESIAN_POINT('Origin',(-48.9660365296434,21.8010840688629,24.2));
#28073=CARTESIAN_POINT('Origin',(-50.3675244741247,18.3322796822559,11.));
#28074=CARTESIAN_POINT('Origin',(-50.3675244741247,18.3322796822559,24.2));
#28075=CARTESIAN_POINT('Origin',(-51.5236269022939,14.7741622717912,11.));
#28076=CARTESIAN_POINT('Origin',(-51.5236269022939,14.7741622717912,24.2));
#28077=CARTESIAN_POINT('Origin',(-52.2796703973459,10.2751081719876,14.5));
#28078=CARTESIAN_POINT('',(-52.5657520484127,9.95448198475441,24.2));
#28079=CARTESIAN_POINT('',(-52.5657520484127,9.95448198475441,14.5));
#28080=CARTESIAN_POINT('',(-51.9935887462791,10.5957343592208,24.2));
#28081=CARTESIAN_POINT('',(-52.0968657068422,10.479986641844,24.2));
#28082=CARTESIAN_POINT('',(-51.9935887462791,10.5957343592208,14.5));
#28083=CARTESIAN_POINT('Origin',(-52.428711399332,11.1440666278319,11.));
#28084=CARTESIAN_POINT('Origin',(-52.428711399332,11.1440666278319,24.2));
#28085=CARTESIAN_POINT('Origin',(-51.4355644344078,-13.8969239803295,14.5));
#28086=CARTESIAN_POINT('',(-51.7433149571624,-13.5970348695551,24.2));
#28087=CARTESIAN_POINT('',(-51.238913447339,-14.0885515659373,24.2));
#28088=CARTESIAN_POINT('',(-51.7433149571624,-13.5970348695551,11.5));
#28089=CARTESIAN_POINT('',(-51.7433149571624,-13.5970348695551,14.5));
#28090=CARTESIAN_POINT('Ctrl Pts',(-51.7433149571624,-13.597034869555,11.5));
#28091=CARTESIAN_POINT('Ctrl Pts',(-51.5386479847417,-13.7964736741256,
11.3527407245756));
#28092=CARTESIAN_POINT('Ctrl Pts',(-51.3334721998344,-13.9964082936921,
11.2067970124651));
#28093=CARTESIAN_POINT('Ctrl Pts',(-51.1278139116532,-14.196813091104,11.0622545443405));
#28094=CARTESIAN_POINT('Origin',(0.,0.,11.25));
#28095=CARTESIAN_POINT('',(-52.0700565974321,-12.286545728569,11.5));
#28096=CARTESIAN_POINT('Origin',(0.,0.,11.5));
#28097=CARTESIAN_POINT('',(-51.8081802498931,-11.4680127538716,11.0622545443405));
#28098=CARTESIAN_POINT('Ctrl Pts',(-52.0700565974321,-12.2865457285691,
11.5));
#28099=CARTESIAN_POINT('Ctrl Pts',(-51.9829772340572,-12.0143663927572,
11.3527407245753));
#28100=CARTESIAN_POINT('Ctrl Pts',(-51.8956813869633,-11.7415104052958,
11.206797012465));
#28101=CARTESIAN_POINT('Ctrl Pts',(-51.8081802498931,-11.4680127538716,
11.0622545443405));
#28102=CARTESIAN_POINT('Ctrl Pts',(-51.8081802498931,-11.4680127538716,
11.0622545443405));
#28103=CARTESIAN_POINT('Ctrl Pts',(-51.7924969656688,-11.4379708252779,
11.0404491452634));
#28104=CARTESIAN_POINT('Ctrl Pts',(-51.7780931636949,-11.4049897426814,
11.0192767711182));
#28105=CARTESIAN_POINT('Ctrl Pts',(-51.766094205967,-11.3697621197168,11.));
#28106=CARTESIAN_POINT('Origin',(-51.9391184236626,-11.8772792412203,14.5));
#28107=CARTESIAN_POINT('',(-52.0700565974321,-12.286545728569,24.2));
#28108=CARTESIAN_POINT('',(-52.0700565974321,-12.286545728569,14.5));
#28109=CARTESIAN_POINT('',(-51.8081802498931,-11.4680127538716,24.2));
#28110=CARTESIAN_POINT('',(-51.8554496100851,-11.6157600795601,24.2));
#28111=CARTESIAN_POINT('',(-51.8081802498931,-11.4680127538716,14.5));
#28112=CARTESIAN_POINT('Origin',(-52.428711399332,-11.1440666278319,11.));
#28113=CARTESIAN_POINT('',(-51.9935887462792,-10.5957343592207,24.2));
#28114=CARTESIAN_POINT('Origin',(-52.428711399332,-11.1440666278319,24.2));
#28115=CARTESIAN_POINT('',(-51.9935887462792,-10.5957343592207,11.0622545443405));
#28116=CARTESIAN_POINT('',(-51.9935887462792,-10.5957343592207,14.5));
#28117=CARTESIAN_POINT('Ctrl Pts',(-51.9151790989041,-10.6683728435365,
11.));
#28118=CARTESIAN_POINT('Ctrl Pts',(-51.9404677257214,-10.641072661922,11.0192757561174));
#28119=CARTESIAN_POINT('Ctrl Pts',(-51.967038401854,-10.6168030742446,11.0404460254343));
#28120=CARTESIAN_POINT('Ctrl Pts',(-51.9935887462792,-10.5957343592207,
11.0622545443405));
#28121=CARTESIAN_POINT('Origin',(-53.0866482765094,4.5331622039544,14.5));
#28122=CARTESIAN_POINT('',(-52.9000254978828,4.14610174160448,11.0622545443405));
#28123=CARTESIAN_POINT('',(-52.9000254978828,4.14610174160448,24.2));
#28124=CARTESIAN_POINT('',(-52.9000254978828,4.14610174160448,14.5));
#28125=CARTESIAN_POINT('',(-53.273271055136,4.92022266630433,24.2));
#28126=CARTESIAN_POINT('',(-52.9673972893853,4.28583257703743,24.2));
#28127=CARTESIAN_POINT('',(-53.2732710551359,4.92022266630433,11.5));
#28128=CARTESIAN_POINT('',(-53.2732710551359,4.92022266630433,14.5));
#28129=CARTESIAN_POINT('Ctrl Pts',(-53.2732710551359,4.92022266630432,11.5));
#28130=CARTESIAN_POINT('Ctrl Pts',(-53.1491590999574,4.66281126610928,11.3527407245754));
#28131=CARTESIAN_POINT('Ctrl Pts',(-53.024738596156,4.40475992810223,11.206797012465));
#28132=CARTESIAN_POINT('Ctrl Pts',(-52.9000254978828,4.14610174160447,11.0622545443405));
#28133=CARTESIAN_POINT('Origin',(0.,0.,11.25));
#28134=CARTESIAN_POINT('',(-53.1320940795741,6.26343186434476,11.5));
#28135=CARTESIAN_POINT('Origin',(0.,0.,11.5));
#28136=CARTESIAN_POINT('Ctrl Pts',(-53.1320940795741,6.26343186434476,11.5));
#28137=CARTESIAN_POINT('Ctrl Pts',(-52.9571754289436,6.48941388139495,11.3527407245755));
#28138=CARTESIAN_POINT('Ctrl Pts',(-52.7818219216653,6.71595770121494,11.206797012465));
#28139=CARTESIAN_POINT('Ctrl Pts',(-52.6060560429105,6.94303427461877,11.0622545443404));
#28140=CARTESIAN_POINT('Ctrl Pts',(-52.8446751870164,4.05466452110769,11.));
#28141=CARTESIAN_POINT('Ctrl Pts',(-52.8614592254452,4.08787763021397,11.0192757561174));
#28142=CARTESIAN_POINT('Ctrl Pts',(-52.8803109936724,4.11853092613597,11.0404460254343));
#28143=CARTESIAN_POINT('Ctrl Pts',(-52.9000254978828,4.14610174160448,11.0622545443405));
#28144=CARTESIAN_POINT('Origin',(-52.8690750612423,6.60323306948177,14.5));
#28145=CARTESIAN_POINT('',(-53.1320940795741,6.26343186434476,24.2));
#28146=CARTESIAN_POINT('',(-53.1320940795741,6.26343186434476,14.5));
#28147=CARTESIAN_POINT('',(-52.7010072733802,6.82036427627618,24.2));
#28148=CARTESIAN_POINT('Origin',(-53.4694330939266,3.73894699268513,11.));
#28149=CARTESIAN_POINT('',(-52.9622319224432,3.25650842494217,11.0622545443405));
#28150=CARTESIAN_POINT('Ctrl Pts',(-52.9622319224432,3.25650842494217,11.0622545443405));
#28151=CARTESIAN_POINT('Ctrl Pts',(-52.9388755042427,3.28106368122768,11.0404491452187));
#28152=CARTESIAN_POINT('Ctrl Pts',(-52.9159388628609,3.3087969065593,11.0192767711931));
#28153=CARTESIAN_POINT('Ctrl Pts',(-52.8946946754776,3.33935251029227,11.));
#28154=CARTESIAN_POINT('',(-52.9622319224432,3.25650842494217,24.2));
#28155=CARTESIAN_POINT('',(-52.9622319224432,3.25650842494217,14.5));
#28156=CARTESIAN_POINT('Origin',(-53.4694330939266,3.73894699268513,24.2));
#28157=CARTESIAN_POINT('Origin',(-52.279670397346,-10.2751081719874,14.5));
#28158=CARTESIAN_POINT('',(-52.5657520484127,-9.95448198475411,24.2));
#28159=CARTESIAN_POINT('',(-52.0968657068422,-10.479986641844,24.2));
#28160=CARTESIAN_POINT('',(-52.5657520484127,-9.95448198475412,11.5));
#28161=CARTESIAN_POINT('',(-52.5657520484127,-9.95448198475411,14.5));
#28162=CARTESIAN_POINT('Ctrl Pts',(-52.5657520484127,-9.95448198475411,
11.5));
#28163=CARTESIAN_POINT('Ctrl Pts',(-52.3754957821853,-10.167711812708,11.352740724576));
#28164=CARTESIAN_POINT('Ctrl Pts',(-52.184766529218,-10.381471740843,11.2067970124653));
#28165=CARTESIAN_POINT('Ctrl Pts',(-51.9935887462792,-10.5957343592207,
11.0622545443405));
#28166=CARTESIAN_POINT('Origin',(0.,0.,11.25));
#28167=CARTESIAN_POINT('',(-52.8002826611136,-8.62439278479999,11.5));
#28168=CARTESIAN_POINT('Origin',(0.,0.,11.5));
#28169=CARTESIAN_POINT('',(-52.4819462572372,-7.82612128585089,11.0622545443405));
#28170=CARTESIAN_POINT('Ctrl Pts',(-52.8002826611136,-8.62439278479999,
11.5));
#28171=CARTESIAN_POINT('Ctrl Pts',(-52.6944291479996,-8.35895081349672,
11.352740724576));
#28172=CARTESIAN_POINT('Ctrl Pts',(-52.5883124776762,-8.09284893997223,
11.2067970124653));
#28173=CARTESIAN_POINT('Ctrl Pts',(-52.4819462572372,-7.82612128585088,
11.0622545443405));
#28174=CARTESIAN_POINT('Ctrl Pts',(-52.4819462572372,-7.82612128585089,
11.0622545443405));
#28175=CARTESIAN_POINT('Ctrl Pts',(-52.4642055576654,-7.79724654843031,
11.0404491452187));
#28176=CARTESIAN_POINT('Ctrl Pts',(-52.4475361986995,-7.76535056472022,
11.0192767711931));
#28177=CARTESIAN_POINT('Ctrl Pts',(-52.4331091150171,-7.73104575932095,
11.));
#28178=CARTESIAN_POINT('Origin',(-52.6411144591754,-8.22525703532544,14.5));
#28179=CARTESIAN_POINT('',(-52.8002826611136,-8.62439278479999,24.2));
#28180=CARTESIAN_POINT('',(-52.8002826611136,-8.62439278479999,14.5));
#28181=CARTESIAN_POINT('',(-52.4819462572372,-7.82612128585089,24.2));
#28182=CARTESIAN_POINT('',(-52.5394068040886,-7.97021136259661,24.2));
#28183=CARTESIAN_POINT('',(-52.4819462572372,-7.82612128585089,14.5));
#28184=CARTESIAN_POINT('Origin',(-53.0783684845482,-7.45967821145951,11.));
#28185=CARTESIAN_POINT('',(-52.6060560429105,-6.94303427461878,24.2));
#28186=CARTESIAN_POINT('Origin',(-53.0783684845482,-7.45967821145951,24.2));
#28187=CARTESIAN_POINT('',(-52.6060560429105,-6.94303427461879,11.0622545443404));
#28188=CARTESIAN_POINT('',(-52.6060560429105,-6.94303427461879,14.5));
#28189=CARTESIAN_POINT('Ctrl Pts',(-52.5329044020197,-7.02096539574592,
11.));
#28190=CARTESIAN_POINT('Ctrl Pts',(-52.556227062611,-6.9919676705692,11.0192757561174));
#28191=CARTESIAN_POINT('Ctrl Pts',(-52.5810400530563,-6.96590372571557,
11.0404460254343));
#28192=CARTESIAN_POINT('Ctrl Pts',(-52.6060560429105,-6.94303427461878,
11.0622545443404));
#28193=CARTESIAN_POINT('Origin',(-53.2735492796914,0.818982261997372,14.5));
#28194=CARTESIAN_POINT('',(-53.0603811317945,0.445882806437586,11.0622545443404));
#28195=CARTESIAN_POINT('',(-53.0603811317945,0.445882806437586,24.2));
#28196=CARTESIAN_POINT('',(-53.0603811317945,0.445882806437586,14.5));
#28197=CARTESIAN_POINT('',(-53.4867174275882,1.19208171755716,24.2));
#28198=CARTESIAN_POINT('',(-53.1373359393522,0.580573645973276,24.2));
#28199=CARTESIAN_POINT('',(-53.4867174275882,1.19208171755716,11.5));
#28200=CARTESIAN_POINT('',(-53.4867174275882,1.19208171755716,14.5));
#28201=CARTESIAN_POINT('Ctrl Pts',(-53.4867174275882,1.19208171755716,11.5));
#28202=CARTESIAN_POINT('Ctrl Pts',(-53.3449516913153,0.943954970938035,
11.3527407245752));
#28203=CARTESIAN_POINT('Ctrl Pts',(-53.2028335182235,0.69521136862767,11.2067970124649));
#28204=CARTESIAN_POINT('Ctrl Pts',(-53.0603811317945,0.445882806437587,
11.0622545443404));
#28205=CARTESIAN_POINT('Origin',(0.,0.,11.25));
#28206=CARTESIAN_POINT('',(-53.4395818891992,2.5418669334897,11.5));
#28207=CARTESIAN_POINT('Origin',(0.,0.,11.5));
#28208=CARTESIAN_POINT('Ctrl Pts',(-53.4395818891992,2.54186693348971,11.5));
#28209=CARTESIAN_POINT('Ctrl Pts',(-53.280853040249,2.77950017796476,11.3527407245753));
#28210=CARTESIAN_POINT('Ctrl Pts',(-53.1217295833205,3.01772419075198,11.206797012465));
#28211=CARTESIAN_POINT('Ctrl Pts',(-52.9622319224432,3.25650842494217,11.0622545443405));
#28212=CARTESIAN_POINT('Ctrl Pts',(-52.9987873134328,0.35852936492104,11.));
#28213=CARTESIAN_POINT('Ctrl Pts',(-53.0178472961609,0.390490773226822,
11.0192757561174));
#28214=CARTESIAN_POINT('Ctrl Pts',(-53.0387914082603,0.419754366385184,
11.0404460254343));
#28215=CARTESIAN_POINT('Ctrl Pts',(-53.0603811317945,0.445882806437586,
11.0622545443404));
#28216=CARTESIAN_POINT('Origin',(-53.2009069058212,2.89918767921594,14.5));
#28217=CARTESIAN_POINT('',(-53.4395818891992,2.5418669334897,24.2));
#28218=CARTESIAN_POINT('',(-53.4395818891992,2.5418669334897,14.5));
#28219=CARTESIAN_POINT('',(-53.048394829969,3.12751378153497,24.2));
#28220=CARTESIAN_POINT('Origin',(-53.6,6.56410684342981E-15,11.));
#28221=CARTESIAN_POINT('',(-53.0603811317945,-0.445882806437573,11.0622545443404));
#28222=CARTESIAN_POINT('Ctrl Pts',(-53.0603811317945,-0.445882806437573,
11.0622545443404));
#28223=CARTESIAN_POINT('Ctrl Pts',(-53.0387944967453,-0.419758104149289,
11.0404491452186));
#28224=CARTESIAN_POINT('Ctrl Pts',(-53.0178482998738,-0.390492456338415,
11.0192767711931));
#28225=CARTESIAN_POINT('Ctrl Pts',(-52.9987873134328,-0.358529364921027,
11.));
#28226=CARTESIAN_POINT('',(-53.0603811317945,-0.445882806437573,24.2));
#28227=CARTESIAN_POINT('',(-53.0603811317945,-0.445882806437573,14.5));
#28228=CARTESIAN_POINT('Origin',(-53.6,6.56410684342981E-15,24.2));
#28229=CARTESIAN_POINT('Origin',(-52.8690750612423,-6.60323306948178,14.5));
#28230=CARTESIAN_POINT('',(-53.1320940795741,-6.26343186434478,24.2));
#28231=CARTESIAN_POINT('',(-52.7010072733802,-6.82036427627619,24.2));
#28232=CARTESIAN_POINT('',(-53.1320940795741,-6.26343186434478,11.5));
#28233=CARTESIAN_POINT('',(-53.1320940795741,-6.26343186434477,14.5));
#28234=CARTESIAN_POINT('Ctrl Pts',(-53.1320940795741,-6.26343186434478,
11.5));
#28235=CARTESIAN_POINT('Ctrl Pts',(-52.9571754289434,-6.48941388139521,
11.3527407245754));
#28236=CARTESIAN_POINT('Ctrl Pts',(-52.7818219216652,-6.71595770121507,
11.206797012465));
#28237=CARTESIAN_POINT('Ctrl Pts',(-52.6060560429105,-6.94303427461878,
11.0622545443404));
#28238=CARTESIAN_POINT('Origin',(0.,0.,11.25));
#28239=CARTESIAN_POINT('',(-53.273271055136,-4.920222666304,11.5));
#28240=CARTESIAN_POINT('Origin',(0.,0.,11.5));
#28241=CARTESIAN_POINT('',(-52.9000254978827,-4.1461017416044,11.0622545443404));
#28242=CARTESIAN_POINT('Ctrl Pts',(-53.273271055136,-4.920222666304,11.5));
#28243=CARTESIAN_POINT('Ctrl Pts',(-53.1491590999572,-4.6628112661087,11.3527407245752));
#28244=CARTESIAN_POINT('Ctrl Pts',(-53.0247385961559,-4.40475992810191,
11.2067970124649));
#28245=CARTESIAN_POINT('Ctrl Pts',(-52.9000254978827,-4.1461017416044,11.0622545443404));
#28246=CARTESIAN_POINT('Ctrl Pts',(-52.9000254978827,-4.1461017416044,11.0622545443404));
#28247=CARTESIAN_POINT('Ctrl Pts',(-52.8803138139007,-4.11853487023683,
11.0404491452186));
#28248=CARTESIAN_POINT('Ctrl Pts',(-52.8614601093052,-4.08787937924104,
11.0192767711931));
#28249=CARTESIAN_POINT('Ctrl Pts',(-52.8446751870164,-4.05466452110769,
11.));
#28250=CARTESIAN_POINT('Origin',(-53.0866482765093,-4.5331622039542,14.5));
#28251=CARTESIAN_POINT('',(-53.273271055136,-4.920222666304,24.2));
#28252=CARTESIAN_POINT('',(-53.273271055136,-4.920222666304,14.5));
#28253=CARTESIAN_POINT('',(-52.9000254978827,-4.1461017416044,24.2));
#28254=CARTESIAN_POINT('',(-52.9673972893853,-4.2858325770374,24.2));
#28255=CARTESIAN_POINT('',(-52.9000254978827,-4.1461017416044,14.5));
#28256=CARTESIAN_POINT('Origin',(-53.4694330939266,-3.73894699268512,11.));
#28257=CARTESIAN_POINT('',(-52.9622319224432,-3.25650842494215,24.2));
#28258=CARTESIAN_POINT('Origin',(-53.4694330939266,-3.73894699268512,24.2));
#28259=CARTESIAN_POINT('',(-52.9622319224432,-3.25650842494215,11.0622545443405));
#28260=CARTESIAN_POINT('',(-52.9622319224432,-3.25650842494215,14.5));
#28261=CARTESIAN_POINT('Ctrl Pts',(-52.8946946754777,-3.33935251029225,
11.));
#28262=CARTESIAN_POINT('Ctrl Pts',(-52.9159377441851,-3.30879851555543,
11.0192757561174));
#28263=CARTESIAN_POINT('Ctrl Pts',(-52.9388721625479,-3.28106719444495,
11.0404460254343));
#28264=CARTESIAN_POINT('Ctrl Pts',(-52.9622319224432,-3.25650842494215,
11.0622545443405));
#28265=CARTESIAN_POINT('Origin',(-53.2009069058212,-2.89918767921592,14.5));
#28266=CARTESIAN_POINT('',(-53.4395818891992,-2.54186693348969,24.2));
#28267=CARTESIAN_POINT('',(-53.048394829969,-3.12751378153496,24.2));
#28268=CARTESIAN_POINT('',(-53.4395818891992,-2.54186693348969,11.5));
#28269=CARTESIAN_POINT('',(-53.4395818891992,-2.54186693348969,14.5));
#28270=CARTESIAN_POINT('Ctrl Pts',(-53.4395818891992,-2.54186693348969,
11.5));
#28271=CARTESIAN_POINT('Ctrl Pts',(-53.280853040249,-2.7795001779648,11.3527407245752));
#28272=CARTESIAN_POINT('Ctrl Pts',(-53.1217295833205,-3.01772419075199,
11.2067970124649));
#28273=CARTESIAN_POINT('Ctrl Pts',(-52.9622319224432,-3.25650842494215,
11.0622545443405));
#28274=CARTESIAN_POINT('Origin',(0.,0.,11.25));
#28275=CARTESIAN_POINT('',(-53.4867174275882,-1.19208171755714,11.5));
#28276=CARTESIAN_POINT('Origin',(0.,0.,11.5));
#28277=CARTESIAN_POINT('Ctrl Pts',(-53.4867174275882,-1.19208171755715,
11.5));
#28278=CARTESIAN_POINT('Ctrl Pts',(-53.3449516913151,-0.943954970937745,
11.3527407245751));
#28279=CARTESIAN_POINT('Ctrl Pts',(-53.2028335182234,-0.695211368627523,
11.2067970124648));
#28280=CARTESIAN_POINT('Ctrl Pts',(-53.0603811317945,-0.445882806437576,
11.0622545443404));
#28281=CARTESIAN_POINT('Origin',(-53.2735492796914,-0.818982261997359,14.5));
#28282=CARTESIAN_POINT('',(-53.4867174275882,-1.19208171755714,24.2));
#28283=CARTESIAN_POINT('',(-53.4867174275882,-1.19208171755714,14.5));
#28284=CARTESIAN_POINT('',(-53.1373359393522,-0.580573645973263,24.2));
#28285=CARTESIAN_POINT('Origin',(0.,-1.62429660857958E-15,24.8232233047034));
#28286=CARTESIAN_POINT('',(-53.0535533905933,-1.29943728686367E-14,24.6464466094067));
#28287=CARTESIAN_POINT('Origin',(0.,-3.24859321715916E-15,24.6464466094067));
#28288=CARTESIAN_POINT('',(-52.2,6.39265629154918E-15,25.));
#28289=CARTESIAN_POINT('',(-52.6267766952966,3.19632814577459E-15,24.8232233047034));
#28290=CARTESIAN_POINT('Origin',(0.,0.,25.));
#28291=CARTESIAN_POINT('Origin',(0.,0.,25.));
#28292=CARTESIAN_POINT('',(-51.1,-6.25794514364297E-15,25.));
#28293=CARTESIAN_POINT('Origin',(0.,0.,25.));
#28294=CARTESIAN_POINT('Origin',(0.,0.,24.6));
#28295=CARTESIAN_POINT('',(-53.5,-6.55186037543834E-15,24.2));
#28296=CARTESIAN_POINT('',(-53.1,-6.50287450347244E-15,24.6));
#28297=CARTESIAN_POINT('Origin',(0.,0.,24.2));
#28298=CARTESIAN_POINT('Origin',(0.,0.,24.2));
#28299=CARTESIAN_POINT('Origin',(0.,0.,24.2));
#28300=CARTESIAN_POINT('Origin',(0.,0.,24.2));
#28301=CARTESIAN_POINT('Origin',(0.,0.,24.2));
#28302=CARTESIAN_POINT('Origin',(0.,0.,24.2));
#28303=CARTESIAN_POINT('Origin',(0.,0.,24.2));
#28304=CARTESIAN_POINT('Origin',(0.,0.,24.2));
#28305=CARTESIAN_POINT('Origin',(0.,0.,24.2));
#28306=CARTESIAN_POINT('Origin',(0.,0.,24.2));
#28307=CARTESIAN_POINT('Origin',(0.,0.,24.2));
#28308=CARTESIAN_POINT('Origin',(0.,0.,24.2));
#28309=CARTESIAN_POINT('Origin',(0.,0.,24.2));
#28310=CARTESIAN_POINT('Origin',(0.,0.,24.2));
#28311=CARTESIAN_POINT('Origin',(0.,0.,24.2));
#28312=CARTESIAN_POINT('Origin',(0.,0.,24.2));
#28313=CARTESIAN_POINT('Origin',(0.,0.,24.2));
#28314=CARTESIAN_POINT('Origin',(0.,0.,24.2));
#28315=CARTESIAN_POINT('Origin',(0.,0.,24.2));
#28316=CARTESIAN_POINT('Origin',(0.,0.,24.2));
#28317=CARTESIAN_POINT('Origin',(0.,0.,24.2));
#28318=CARTESIAN_POINT('Origin',(0.,0.,24.2));
#28319=CARTESIAN_POINT('Origin',(0.,0.,24.2));
#28320=CARTESIAN_POINT('Origin',(0.,0.,24.2));
#28321=CARTESIAN_POINT('Origin',(0.,0.,24.2));
#28322=CARTESIAN_POINT('Origin',(0.,0.,24.2));
#28323=CARTESIAN_POINT('Origin',(0.,0.,24.2));
#28324=CARTESIAN_POINT('Origin',(0.,0.,24.2));
#28325=CARTESIAN_POINT('Origin',(0.,0.,24.2));
#28326=CARTESIAN_POINT('Origin',(0.,0.,24.2));
#28327=CARTESIAN_POINT('Origin',(0.,0.,24.2));
#28328=CARTESIAN_POINT('Origin',(0.,0.,24.2));
#28329=CARTESIAN_POINT('Origin',(0.,0.,24.2));
#28330=CARTESIAN_POINT('Origin',(0.,0.,24.2));
#28331=CARTESIAN_POINT('Origin',(0.,0.,24.2));
#28332=CARTESIAN_POINT('Origin',(0.,0.,24.2));
#28333=CARTESIAN_POINT('Origin',(0.,0.,24.2));
#28334=CARTESIAN_POINT('Origin',(0.,0.,24.2));
#28335=CARTESIAN_POINT('Origin',(0.,0.,24.2));
#28336=CARTESIAN_POINT('Origin',(0.,0.,24.2));
#28337=CARTESIAN_POINT('Origin',(0.,0.,24.2));
#28338=CARTESIAN_POINT('Origin',(0.,0.,24.2));
#28339=CARTESIAN_POINT('Origin',(0.,0.,24.2));
#28340=CARTESIAN_POINT('Origin',(0.,0.,24.2));
#28341=CARTESIAN_POINT('Origin',(0.,0.,24.2));
#28342=CARTESIAN_POINT('Origin',(0.,0.,24.2));
#28343=CARTESIAN_POINT('Origin',(0.,0.,24.2));
#28344=CARTESIAN_POINT('Origin',(0.,0.,24.2));
#28345=CARTESIAN_POINT('Origin',(0.,0.,24.2));
#28346=CARTESIAN_POINT('Origin',(0.,0.,24.2));
#28347=CARTESIAN_POINT('Origin',(0.,0.,24.2));
#28348=CARTESIAN_POINT('Origin',(0.,0.,24.2));
#28349=CARTESIAN_POINT('Origin',(0.,0.,24.2));
#28350=CARTESIAN_POINT('Origin',(0.,0.,24.2));
#28351=CARTESIAN_POINT('Origin',(0.,0.,24.2));
#28352=CARTESIAN_POINT('Origin',(0.,0.,24.2));
#28353=CARTESIAN_POINT('Origin',(0.,0.,24.2));
#28354=CARTESIAN_POINT('Origin',(0.,0.,24.2));
#28355=CARTESIAN_POINT('Origin',(0.,0.,24.2));
#28356=CARTESIAN_POINT('Origin',(0.,0.,24.2));
#28357=CARTESIAN_POINT('Origin',(0.,0.,24.2));
#28358=CARTESIAN_POINT('Origin',(0.,0.,24.2));
#28359=CARTESIAN_POINT('Origin',(0.,0.,24.2));
#28360=CARTESIAN_POINT('Origin',(0.,0.,24.2));
#28361=CARTESIAN_POINT('Origin',(0.,0.,24.2));
#28362=CARTESIAN_POINT('Origin',(0.,0.,24.2));
#28363=CARTESIAN_POINT('Origin',(0.,0.,24.2));
#28364=CARTESIAN_POINT('Origin',(0.,0.,24.2));
#28365=CARTESIAN_POINT('Origin',(0.,0.,24.2));
#28366=CARTESIAN_POINT('Origin',(0.,0.,24.2));
#28367=CARTESIAN_POINT('Origin',(0.,0.,24.2));
#28368=CARTESIAN_POINT('Origin',(0.,0.,24.2));
#28369=CARTESIAN_POINT('Origin',(0.,0.,24.2));
#28370=CARTESIAN_POINT('Origin',(0.,0.,24.2));
#28371=CARTESIAN_POINT('Origin',(0.,0.,24.2));
#28372=CARTESIAN_POINT('Origin',(0.,0.,24.2));
#28373=CARTESIAN_POINT('Origin',(0.,0.,24.2));
#28374=CARTESIAN_POINT('Origin',(0.,0.,24.2));
#28375=CARTESIAN_POINT('Origin',(0.,0.,24.2));
#28376=CARTESIAN_POINT('Origin',(0.,0.,24.2));
#28377=CARTESIAN_POINT('Origin',(0.,0.,24.2));
#28378=CARTESIAN_POINT('Origin',(0.,0.,24.2));
#28379=CARTESIAN_POINT('Origin',(0.,0.,24.2));
#28380=CARTESIAN_POINT('Origin',(0.,0.,24.2));
#28381=CARTESIAN_POINT('Origin',(0.,0.,24.2));
#28382=CARTESIAN_POINT('Origin',(0.,0.,24.2));
#28383=CARTESIAN_POINT('Origin',(0.,0.,24.2));
#28384=CARTESIAN_POINT('Origin',(0.,0.,24.2));
#28385=CARTESIAN_POINT('Origin',(0.,0.,24.2));
#28386=CARTESIAN_POINT('Origin',(0.,0.,24.2));
#28387=CARTESIAN_POINT('Origin',(0.,0.,24.2));
#28388=CARTESIAN_POINT('Origin',(0.,0.,24.2));
#28389=CARTESIAN_POINT('Origin',(0.,0.,24.2));
#28390=CARTESIAN_POINT('Origin',(0.,0.,24.2));
#28391=CARTESIAN_POINT('Origin',(0.,0.,24.2));
#28392=CARTESIAN_POINT('Origin',(0.,0.,24.2));
#28393=CARTESIAN_POINT('Origin',(0.,0.,24.2));
#28394=CARTESIAN_POINT('Origin',(0.,0.,24.2));
#28395=CARTESIAN_POINT('Origin',(0.,0.,24.2));
#28396=CARTESIAN_POINT('Origin',(0.,0.,24.2));
#28397=CARTESIAN_POINT('Origin',(0.,0.,24.2));
#28398=CARTESIAN_POINT('Origin',(9.57952682562336,-29.4827520051498,22.3));
#28399=CARTESIAN_POINT('',(-3.32047317437664,-29.4827520051498,22.5));
#28400=CARTESIAN_POINT('Origin',(9.57952682562336,-29.4827520051498,22.5));
#28401=CARTESIAN_POINT('',(-2.92047317437664,-29.4827520051498,22.1));
#28402=CARTESIAN_POINT('',(-3.12047317437664,-29.4827520051498,22.3));
#28403=CARTESIAN_POINT('Origin',(9.57952682562336,-29.4827520051498,22.1));
#28404=CARTESIAN_POINT('Origin',(0.,0.,22.5));
#28405=CARTESIAN_POINT('',(-50.5,-6.18446633569413E-15,22.5));
#28406=CARTESIAN_POINT('Origin',(0.,0.,22.5));
#28407=CARTESIAN_POINT('',(18.1,-1.57979437090009E-15,22.5));
#28408=CARTESIAN_POINT('Origin',(31.,0.,22.5));
#28409=CARTESIAN_POINT('',(-37.9795268256234,18.2213428210667,22.5));
#28410=CARTESIAN_POINT('Origin',(-25.0795268256234,18.2213428210667,22.5));
#28411=CARTESIAN_POINT('',(-5.025,-6.15385016571545E-16,22.5));
#28412=CARTESIAN_POINT('Origin',(0.,0.,22.5));
#28413=CARTESIAN_POINT('',(-37.9795268256234,-18.2213428210667,22.5));
#28414=CARTESIAN_POINT('Origin',(-25.0795268256234,-18.2213428210667,22.5));
#28415=CARTESIAN_POINT('',(-3.32047317437663,29.4827520051498,22.5));
#28416=CARTESIAN_POINT('Origin',(9.57952682562337,29.4827520051498,22.5));
#28417=CARTESIAN_POINT('Origin',(9.57952682562336,-29.4827520051498,22.5));
#28418=CARTESIAN_POINT('',(-2.92047317437664,-29.4827520051498,14.5));
#28419=CARTESIAN_POINT('',(-2.92047317437664,-29.4827520051498,22.5));
#28420=CARTESIAN_POINT('Origin',(9.57952682562336,-29.4827520051498,14.5));
#28421=CARTESIAN_POINT('Origin',(31.,0.,22.3));
#28422=CARTESIAN_POINT('',(18.5,1.53080849893419E-15,22.1));
#28423=CARTESIAN_POINT('',(18.3,-1.55530143491714E-15,22.3));
#28424=CARTESIAN_POINT('Origin',(31.,0.,22.1));
#28425=CARTESIAN_POINT('Origin',(31.,0.,22.5));
#28426=CARTESIAN_POINT('',(18.5,-1.53080849893419E-15,14.5));
#28427=CARTESIAN_POINT('',(18.5,1.53080849893419E-15,22.5));
#28428=CARTESIAN_POINT('Origin',(31.,0.,14.5));
#28429=CARTESIAN_POINT('Origin',(9.57952682562337,29.4827520051498,22.3));
#28430=CARTESIAN_POINT('',(-2.92047317437663,29.4827520051498,22.1));
#28431=CARTESIAN_POINT('',(-3.12047317437663,29.4827520051498,22.3));
#28432=CARTESIAN_POINT('Origin',(9.57952682562337,29.4827520051498,22.1));
#28433=CARTESIAN_POINT('Origin',(9.57952682562337,29.4827520051498,22.5));
#28434=CARTESIAN_POINT('',(-2.92047317437663,29.4827520051498,14.5));
#28435=CARTESIAN_POINT('',(-2.92047317437663,29.4827520051498,22.5));
#28436=CARTESIAN_POINT('Origin',(9.57952682562337,29.4827520051498,14.5));
#28437=CARTESIAN_POINT('Origin',(-25.0795268256234,18.2213428210667,22.3));
#28438=CARTESIAN_POINT('',(-37.5795268256234,18.2213428210667,22.1));
#28439=CARTESIAN_POINT('',(-37.7795268256234,18.2213428210667,22.3));
#28440=CARTESIAN_POINT('Origin',(-25.0795268256234,18.2213428210667,22.1));
#28441=CARTESIAN_POINT('Origin',(-25.0795268256234,18.2213428210667,22.5));
#28442=CARTESIAN_POINT('',(-37.5795268256234,18.2213428210667,14.5));
#28443=CARTESIAN_POINT('',(-37.5795268256234,18.2213428210667,22.5));
#28444=CARTESIAN_POINT('Origin',(-25.0795268256234,18.2213428210667,14.5));
#28445=CARTESIAN_POINT('Origin',(-25.0795268256234,-18.2213428210667,22.3));
#28446=CARTESIAN_POINT('',(-37.5795268256234,-18.2213428210667,22.1));
#28447=CARTESIAN_POINT('',(-37.7795268256234,-18.2213428210667,22.3));
#28448=CARTESIAN_POINT('Origin',(-25.0795268256234,-18.2213428210667,22.1));
#28449=CARTESIAN_POINT('Origin',(-25.0795268256234,-18.2213428210667,22.5));
#28450=CARTESIAN_POINT('',(-37.5795268256234,-18.2213428210667,14.5));
#28451=CARTESIAN_POINT('',(-37.5795268256234,-18.2213428210667,22.5));
#28452=CARTESIAN_POINT('Origin',(-25.0795268256234,-18.2213428210667,14.5));
#28453=CARTESIAN_POINT('Origin',(0.,0.,24.7));
#28454=CARTESIAN_POINT('',(-50.5,6.18446633569413E-15,24.4));
#28455=CARTESIAN_POINT('',(-50.8,-6.22120573966855E-15,24.7));
#28456=CARTESIAN_POINT('Origin',(0.,0.,24.4));
#28457=CARTESIAN_POINT('Origin',(0.,0.,22.5));
#28458=CARTESIAN_POINT('',(-50.5,-6.18446633569413E-15,22.5));
#28459=CARTESIAN_POINT('Origin',(0.,0.,14.5));
#28460=CARTESIAN_POINT('Origin',(0.,0.,14.5));
#28461=CARTESIAN_POINT('Origin',(0.,0.,14.5));
#28462=CARTESIAN_POINT('Origin',(0.,0.,14.5));
#28463=CARTESIAN_POINT('Origin',(0.,0.,14.5));
#28464=CARTESIAN_POINT('Origin',(0.,0.,14.5));
#28465=CARTESIAN_POINT('Origin',(0.,0.,14.5));
#28466=CARTESIAN_POINT('Origin',(0.,0.,14.5));
#28467=CARTESIAN_POINT('Origin',(0.,0.,14.5));
#28468=CARTESIAN_POINT('Origin',(0.,0.,14.5));
#28469=CARTESIAN_POINT('Origin',(53.4694330939266,-3.73894699268513,24.2));
#28470=CARTESIAN_POINT('Origin',(53.0783684845482,-7.45967821145953,24.2));
#28471=CARTESIAN_POINT('Origin',(52.428711399332,-11.1440666278319,24.2));
#28472=CARTESIAN_POINT('Origin',(51.5236269022939,-14.7741622717911,24.2));
#28473=CARTESIAN_POINT('Origin',(50.3675244741247,-18.3322796822558,24.2));
#28474=CARTESIAN_POINT('Origin',(48.9660365296434,-21.8010840688629,24.2));
#28475=CARTESIAN_POINT('Origin',(47.3259909772385,-25.1636757653237,11.));
#28476=CARTESIAN_POINT('Origin',(47.3259909772385,-25.1636757653237,24.2));
#28477=CARTESIAN_POINT('Origin',(47.3259909772385,-25.1636757653237,24.2));
#28478=CARTESIAN_POINT('Origin',(45.4553779539844,-28.4036725628998,24.2));
#28479=CARTESIAN_POINT('Origin',(43.3633108984972,-31.5052895228766,24.2));
#28480=CARTESIAN_POINT('Origin',(41.0599821511772,-34.4534158791985,24.2));
#28481=CARTESIAN_POINT('Origin',(38.5566132981517,-37.2336886566023,24.2));
#28482=CARTESIAN_POINT('Origin',(35.8654005008348,-39.8325626455884,24.2));
#28483=CARTESIAN_POINT('Origin',(32.9994550774553,-42.2373763933203,24.2));
#28484=CARTESIAN_POINT('Origin',(29.972739626032,-44.4364138889502,24.2));
#28485=CARTESIAN_POINT('Origin',(26.8,-46.4189616428459,24.2));
#28486=CARTESIAN_POINT('Origin',(23.4966934678945,-48.1753608816354,24.2));
#28487=CARTESIAN_POINT('Origin',(20.0789134070929,-49.6970546047798,11.));
#28488=CARTESIAN_POINT('Origin',(20.0789134070929,-49.6970546047798,24.2));
#28489=CARTESIAN_POINT('Origin',(20.0789134070929,-49.6970546047798,24.2));
#28490=CARTESIAN_POINT('Origin',(16.5633108984972,-50.9766292734202,24.2));
#28491=CARTESIAN_POINT('Origin',(12.9670136041422,-52.0078509283934,24.2));
#28492=CARTESIAN_POINT('Origin',(9.30754232294745,-52.7856955614544,24.2));
#28493=CARTESIAN_POINT('Origin',(5.6027256311462,-53.3063735917395,24.2));
#28494=CARTESIAN_POINT('Origin',(1.87061302325407,-53.5673483282235,24.2));
#28495=CARTESIAN_POINT('Origin',(-1.87061302325404,-53.5673483282235,24.2));
#28496=CARTESIAN_POINT('Origin',(-5.60272563114622,-53.3063735917395,24.2));
#28497=CARTESIAN_POINT('Origin',(-9.30754232294747,-52.7856955614544,24.2));
#28498=CARTESIAN_POINT('Origin',(-12.9670136041422,-52.0078509283934,24.2));
#28499=CARTESIAN_POINT('Origin',(-16.5633108984972,-50.9766292734202,11.));
#28500=CARTESIAN_POINT('Origin',(-16.5633108984972,-50.9766292734202,24.2));
#28501=CARTESIAN_POINT('Origin',(-16.5633108984972,-50.9766292734202,24.2));
#28502=CARTESIAN_POINT('Origin',(-20.0789134070929,-49.6970546047798,24.2));
#28503=CARTESIAN_POINT('Origin',(-23.4966934678946,-48.1753608816353,24.2));
#28504=CARTESIAN_POINT('Origin',(-26.8,-46.4189616428459,24.2));
#28505=CARTESIAN_POINT('Origin',(-29.972739626032,-44.4364138889502,24.2));
#28506=CARTESIAN_POINT('Origin',(-32.9994550774553,-42.2373763933203,24.2));
#28507=CARTESIAN_POINT('Origin',(-35.8654005008348,-39.8325626455883,24.2));
#28508=CARTESIAN_POINT('Origin',(-38.5566132981517,-37.2336886566023,24.2));
#28509=CARTESIAN_POINT('Origin',(-41.0599821511772,-34.4534158791985,24.2));
#28510=CARTESIAN_POINT('Origin',(-43.3633108984972,-31.5052895228766,24.2));
#28511=CARTESIAN_POINT('Origin',(-45.4553779539844,-28.4036725628998,24.2));
#28512=CARTESIAN_POINT('Origin',(-47.3259909772385,-25.1636757653237,24.2));
#28513=CARTESIAN_POINT('Origin',(-48.9660365296434,-21.8010840688629,24.2));
#28514=CARTESIAN_POINT('Origin',(-50.3675244741247,-18.3322796822558,24.2));
#28515=CARTESIAN_POINT('Origin',(-51.5236269022939,-14.7741622717911,24.2));
#28516=CARTESIAN_POINT('Origin',(-52.428711399332,-11.1440666278319,24.2));
#28517=CARTESIAN_POINT('Origin',(-53.0783684845482,-7.45967821145951,24.2));
#28518=CARTESIAN_POINT('Origin',(-53.4694330939266,-3.73894699268512,24.2));
#28519=CARTESIAN_POINT('Origin',(-53.6,6.56410684342981E-15,24.2));
#28520=CARTESIAN_POINT('Origin',(-53.4694330939266,3.73894699268513,24.2));
#28521=CARTESIAN_POINT('Origin',(-53.0783684845482,7.4596782114595,24.2));
#28522=CARTESIAN_POINT('Origin',(-52.428711399332,11.1440666278319,24.2));
#28523=CARTESIAN_POINT('Origin',(-51.5236269022939,14.7741622717912,24.2));
#28524=CARTESIAN_POINT('Origin',(-50.3675244741247,18.3322796822559,24.2));
#28525=CARTESIAN_POINT('Origin',(-48.9660365296434,21.8010840688629,24.2));
#28526=CARTESIAN_POINT('Origin',(-47.3259909772385,25.1636757653237,24.2));
#28527=CARTESIAN_POINT('Origin',(-45.4553779539844,28.4036725628998,24.2));
#28528=CARTESIAN_POINT('Origin',(-43.3633108984972,31.5052895228766,24.2));
#28529=CARTESIAN_POINT('Origin',(-41.0599821511772,34.4534158791985,24.2));
#28530=CARTESIAN_POINT('Origin',(-38.5566132981517,37.2336886566023,24.2));
#28531=CARTESIAN_POINT('Origin',(-35.8654005008348,39.8325626455883,24.2));
#28532=CARTESIAN_POINT('Origin',(-32.9994550774553,42.2373763933203,24.2));
#28533=CARTESIAN_POINT('Origin',(-29.972739626032,44.4364138889502,24.2));
#28534=CARTESIAN_POINT('Origin',(-26.8,46.4189616428459,24.2));
#28535=CARTESIAN_POINT('Origin',(-23.4966934678946,48.1753608816354,24.2));
#28536=CARTESIAN_POINT('Origin',(-20.0789134070929,49.6970546047798,24.2));
#28537=CARTESIAN_POINT('Origin',(-16.5633108984972,50.9766292734202,24.2));
#28538=CARTESIAN_POINT('Origin',(-12.9670136041422,52.0078509283934,24.2));
#28539=CARTESIAN_POINT('Origin',(-9.30754232294747,52.7856955614544,24.2));
#28540=CARTESIAN_POINT('Origin',(-5.60272563114623,53.3063735917395,24.2));
#28541=CARTESIAN_POINT('Origin',(-1.87061302325405,53.5673483282235,24.2));
#28542=CARTESIAN_POINT('Origin',(-1.87061302325405,53.5673483282235,24.2));
#28543=CARTESIAN_POINT('Origin',(-1.87061302325405,53.5673483282235,11.));
#28544=CARTESIAN_POINT('Origin',(1.87061302325406,53.5673483282235,24.2));
#28545=CARTESIAN_POINT('Origin',(5.60272563114623,53.3063735917395,24.2));
#28546=CARTESIAN_POINT('Origin',(9.30754232294747,52.7856955614544,24.2));
#28547=CARTESIAN_POINT('Origin',(12.9670136041422,52.0078509283934,24.2));
#28548=CARTESIAN_POINT('Origin',(16.5633108984972,50.9766292734202,24.2));
#28549=CARTESIAN_POINT('Origin',(20.0789134070929,49.6970546047798,24.2));
#28550=CARTESIAN_POINT('Origin',(23.4966934678946,48.1753608816354,24.2));
#28551=CARTESIAN_POINT('Origin',(26.8,46.4189616428459,24.2));
#28552=CARTESIAN_POINT('Origin',(29.972739626032,44.4364138889502,24.2));
#28553=CARTESIAN_POINT('Origin',(32.9994550774553,42.2373763933203,11.));
#28554=CARTESIAN_POINT('Origin',(32.9994550774553,42.2373763933203,24.2));
#28555=CARTESIAN_POINT('Origin',(32.9994550774553,42.2373763933203,24.2));
#28556=CARTESIAN_POINT('Origin',(35.8654005008348,39.8325626455883,24.2));
#28557=CARTESIAN_POINT('Origin',(38.5566132981517,37.2336886566023,24.2));
#28558=CARTESIAN_POINT('Origin',(41.0599821511772,34.4534158791985,24.2));
#28559=CARTESIAN_POINT('Origin',(43.3633108984972,31.5052895228766,24.2));
#28560=CARTESIAN_POINT('Origin',(45.4553779539844,28.4036725628998,24.2));
#28561=CARTESIAN_POINT('Origin',(47.3259909772385,25.1636757653237,24.2));
#28562=CARTESIAN_POINT('Origin',(48.9660365296434,21.8010840688629,24.2));
#28563=CARTESIAN_POINT('Origin',(50.3675244741247,18.3322796822558,24.2));
#28564=CARTESIAN_POINT('Origin',(51.5236269022939,14.7741622717912,24.2));
#28565=CARTESIAN_POINT('Origin',(52.428711399332,11.1440666278319,11.));
#28566=CARTESIAN_POINT('Origin',(52.428711399332,11.1440666278319,24.2));
#28567=CARTESIAN_POINT('Origin',(52.428711399332,11.1440666278319,24.2));
#28568=CARTESIAN_POINT('Origin',(53.0783684845482,7.45967821145951,24.2));
#28569=CARTESIAN_POINT('Origin',(53.4694330939266,3.73894699268512,24.2));
#28570=CARTESIAN_POINT('Origin',(53.6,0.,24.2));
#28571=CARTESIAN_POINT('Origin',(-6.18033988749895,-19.0211303259031,14.5));
#28572=CARTESIAN_POINT('',(-7.68033988749895,-19.0211303259031,14.5));
#28573=CARTESIAN_POINT('Origin',(-6.18033988749895,-19.0211303259031,14.5));
#28574=CARTESIAN_POINT('',(-6.18033988749895,-19.0211303259031,16.));
#28575=CARTESIAN_POINT('',(-7.68033988749895,-19.0211303259031,14.5));
#28576=CARTESIAN_POINT('Origin',(-20.,2.44929359829471E-15,14.5));
#28577=CARTESIAN_POINT('',(-21.5,2.2655965784226E-15,14.5));
#28578=CARTESIAN_POINT('Origin',(-20.,2.44929359829471E-15,14.5));
#28579=CARTESIAN_POINT('',(-20.,2.44929359829471E-15,16.));
#28580=CARTESIAN_POINT('',(-21.5,2.2655965784226E-15,14.5));
#28581=CARTESIAN_POINT('Origin',(-6.18033988749895,19.0211303259031,14.5));
#28582=CARTESIAN_POINT('',(-7.68033988749895,19.0211303259031,14.5));
#28583=CARTESIAN_POINT('Origin',(-6.18033988749895,19.0211303259031,14.5));
#28584=CARTESIAN_POINT('',(-6.18033988749895,19.0211303259031,16.));
#28585=CARTESIAN_POINT('',(-7.68033988749895,19.0211303259031,14.5));
#28586=CARTESIAN_POINT('Origin',(16.1803398874989,11.7557050458495,14.5));
#28587=CARTESIAN_POINT('',(14.6803398874989,11.7557050458495,14.5));
#28588=CARTESIAN_POINT('Origin',(16.1803398874989,11.7557050458495,14.5));
#28589=CARTESIAN_POINT('',(16.1803398874989,11.7557050458495,16.));
#28590=CARTESIAN_POINT('',(14.6803398874989,11.7557050458495,14.5));
#28591=CARTESIAN_POINT('Origin',(16.1803398874989,-11.7557050458495,14.5));
#28592=CARTESIAN_POINT('',(14.6803398874989,-11.7557050458495,14.5));
#28593=CARTESIAN_POINT('Origin',(16.1803398874989,-11.7557050458495,14.5));
#28594=CARTESIAN_POINT('',(16.1803398874989,-11.7557050458495,16.));
#28595=CARTESIAN_POINT('',(14.6803398874989,-11.7557050458495,14.5));
#28596=CARTESIAN_POINT('Origin',(0.,0.,22.5));
#28597=CARTESIAN_POINT('',(-5.025,-6.15385016571545E-16,14.5));
#28598=CARTESIAN_POINT('',(-5.025,6.15385016571545E-16,22.5));
#28599=CARTESIAN_POINT('Origin',(0.,0.,14.5));
#28600=CARTESIAN_POINT('Origin',(0.,0.,14.5));
#38503=UNCERTAINTY_MEASURE_WITH_UNIT(LENGTH_MEASURE(0.01),#38529,
'DISTANCE_ACCURACY_VALUE',
'Maximum model space distance between geometric entities at asserted c
onnectivities');
#38514=UNCERTAINTY_MEASURE_WITH_UNIT(LENGTH_MEASURE(0.01),#38529,
'DISTANCE_ACCURACY_VALUE',
'Maximum model space distance between geometric entities at asserted c
onnectivities');
#38517=(
GEOMETRIC_REPRESENTATION_CONTEXT(3)
GLOBAL_UNCERTAINTY_ASSIGNED_CONTEXT((#38503))
GLOBAL_UNIT_ASSIGNED_CONTEXT((#38529,#38531,#38532))
REPRESENTATION_CONTEXT('','3D')
);
#38528=(
GEOMETRIC_REPRESENTATION_CONTEXT(3)
GLOBAL_UNCERTAINTY_ASSIGNED_CONTEXT((#38514))
GLOBAL_UNIT_ASSIGNED_CONTEXT((#38529,#38531,#38532))
REPRESENTATION_CONTEXT('','3D')
);
#38529=(
LENGTH_UNIT()
NAMED_UNIT(*)
SI_UNIT(.MILLI.,.METRE.)
);
#38531=(
NAMED_UNIT(*)
PLANE_ANGLE_UNIT()
SI_UNIT($,.RADIAN.)
);
#38532=(
NAMED_UNIT(*)
SI_UNIT($,.STERADIAN.)
SOLID_ANGLE_UNIT()
);
#38535=SHAPE_DEFINITION_REPRESENTATION(#38548,#38577);
#38548=PRODUCT_DEFINITION_SHAPE('',$,#38591);
#38577=SHAPE_REPRESENTATION('',(#17323),#38517);
#38588=PRODUCT_DEFINITION_CONTEXT('part definition',#38629,'design');
#38591=PRODUCT_DEFINITION('2026-10-20-13-39-04-258',
'02_Revolving_Objective_Disc_D107',#38604,#38588);
#38604=PRODUCT_DEFINITION_FORMATION('',$,#38633);
#38629=APPLICATION_CONTEXT(
'Core Data for Automotive Mechanical Design Process');
#38630=PRODUCT_CONTEXT('part definition',#38629,'mechanical');
#38633=PRODUCT('2026-10-20-13-39-04-258',
'02_Revolving_Objective_Disc_D107',$,(#38630));
#38714=COLOUR_RGB('Off White',0.89,0.88,0.83);
#38715=FILL_AREA_STYLE_COLOUR('',#38714);
#38716=FILL_AREA_STYLE('',(#38715));
#38717=SURFACE_STYLE_FILL_AREA(#38716);
#38718=SURFACE_SIDE_STYLE('',(#38717));
#38719=SURFACE_STYLE_USAGE(.BOTH.,#38718);
#38720=PRESENTATION_STYLE_ASSIGNMENT((#38719));
ENDSEC;
END-ISO-10303-21;
